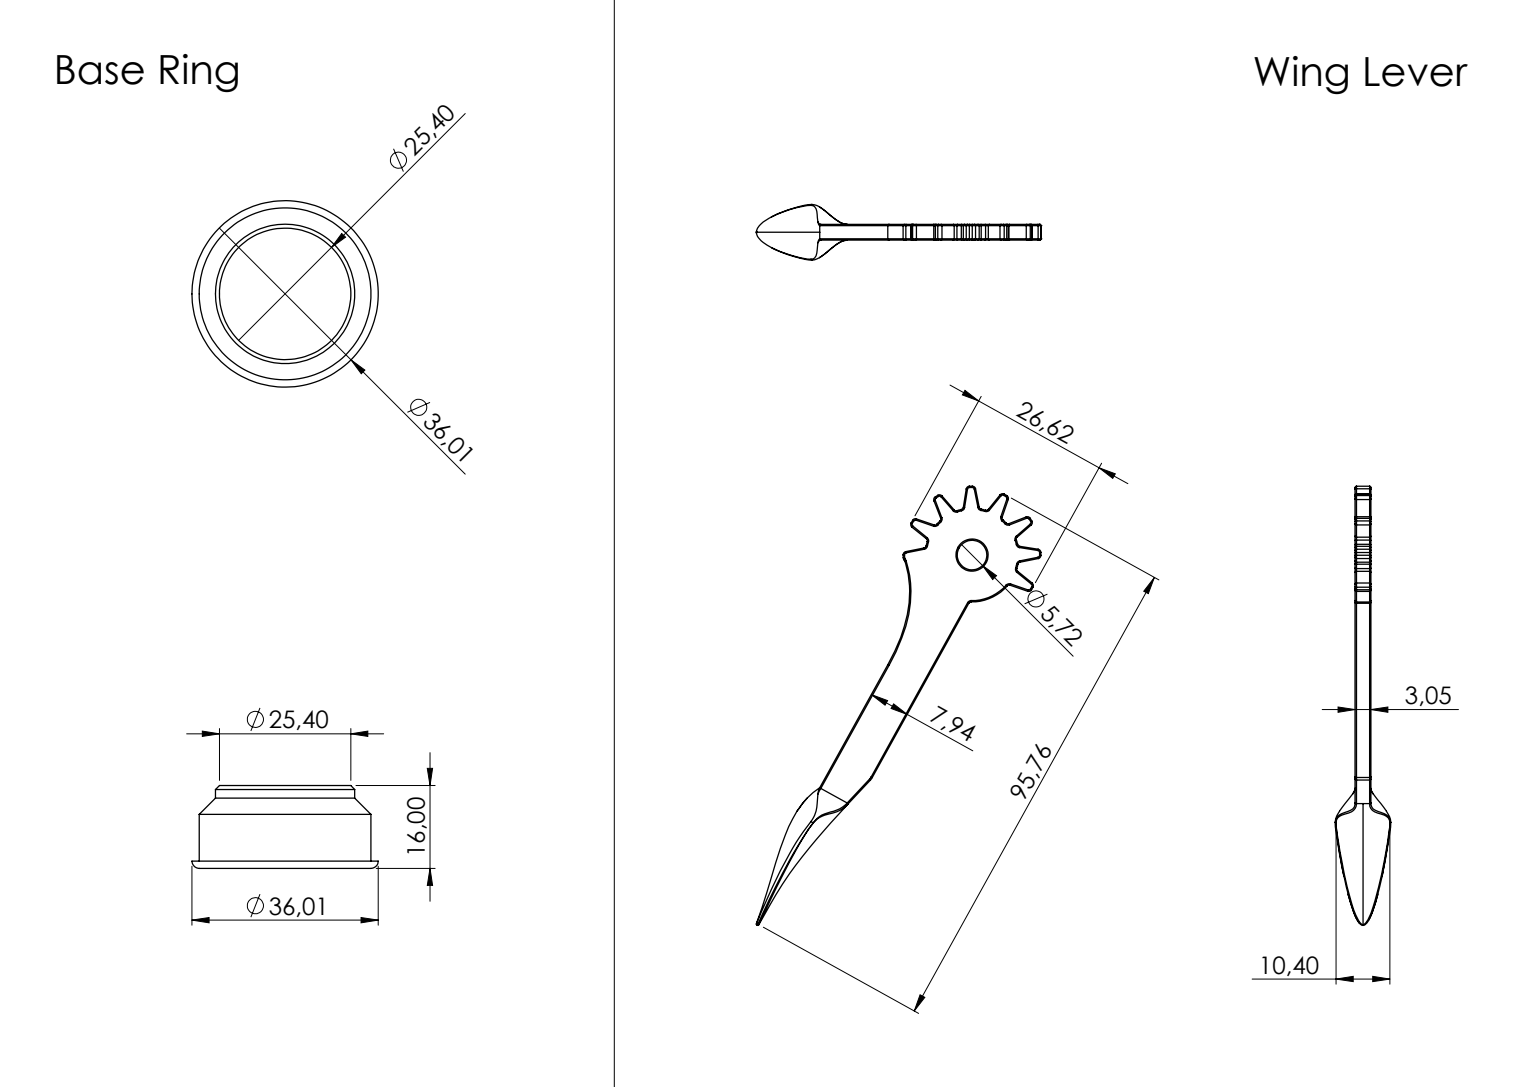
ISO-10303-21;
HEADER;
FILE_DESCRIPTION (('STEP AP214'),
    '1' );
FILE_NAME ('Wing Lever.step',
    '2026-10-06T14:27:08',
    ( '' ),
    ( '' ),
    'SwSTEP 2.0',
    'SolidWorks 2020',
    '' );
FILE_SCHEMA (( 'AUTOMOTIVE_DESIGN' ));
ENDSEC;

DATA;
#7=CARTESIAN_POINT ( 'NONE',  ( -47.84919564605845466, 19.39087073395056393, 5.212699772323899694 ) ) ;
#16=ORIENTED_EDGE ( 'NONE', *, *, #18091, .T. ) ;
#25=VERTEX_POINT ( 'NONE', #23978 ) ;
#26=CARTESIAN_POINT ( 'NONE',  ( -45.52520984822221095, 18.49555408152312452, 0.5880787195337303652 ) ) ;
#39=CARTESIAN_POINT ( 'NONE',  ( -8.428339483816529309, 74.57444062528223583, -1.523999999999996913 ) ) ;
#40=CARTESIAN_POINT ( 'NONE',  ( -58.67410397513675235, -0.3138866149764163449, 0.3147537707000222507 ) ) ;
#41=DIRECTION ( 'NONE',  ( -5.188838149069471174E-16, 1.699382548006136313E-16, 1.000000000000000000 ) ) ;
#44=AXIS2_PLACEMENT_3D ( 'NONE', #23205, #7689, #33679 ) ;
#57=FACE_OUTER_BOUND ( 'NONE', #41013, .T. ) ;
#58=DIRECTION ( 'NONE',  ( 0.6850534820564689875, -0.7284927773988614241, 8.537024980200769556E-16 ) ) ;
#64=( BOUNDED_SURFACE ( )  B_SPLINE_SURFACE ( 3, 2, ( 
 ( #13288, #26273, #2675 ),
 ( #25450, #22223, #6076 ),
 ( #23483, #20083, #948 ),
 ( #10925, #7750, #33106 ),
 ( #39712, #10513, #30310 ),
 ( #17523, #39496, #3725 ),
 ( #3937, #26910, #7329 ),
 ( #23697, #40345, #23915 ),
 ( #16896, #36508, #14119 ),
 ( #36717, #7538, #17320 ),
 ( #27333, #20287, #27119 ),
 ( #20500, #33315, #33527 ),
 ( #4144, #29899, #40134 ),
 ( #37135, #17106, #30523 ),
 ( #16684, #30108, #10716 ),
 ( #4360, #1154, #36307 ) ),
 .UNSPECIFIED., .F., .F., .T. ) 
 B_SPLINE_SURFACE_WITH_KNOTS ( ( 4, 2, 2, 2, 2, 2, 2, 4 ),
 ( 3, 3 ),
 ( -4.336808689942017736E-17, 0.002643305330645566355, 0.003964957995968371000, 0.005286610661291176079, 0.01057322132258239553, 0.01321652665322800395, 0.01585983198387361237, 0.02114644264516483269 ),
 ( 0.000000000000000000, 1.000000000000000000 ),
 .UNSPECIFIED. ) 
 GEOMETRIC_REPRESENTATION_ITEM ( )  RATIONAL_B_SPLINE_SURFACE ( (
 ( 1.000000000000000000, 0.7071067811865429098, 1.000000000000000000),
 ( 1.000000000000000000, 0.7071067811865429098, 1.000000000000000000),
 ( 1.000000000000000000, 0.7071067811865475727, 1.000000000000000000),
 ( 1.000000000000000000, 0.7071067811865475727, 1.000000000000000000),
 ( 1.000000000000000000, 0.7071067811865481278, 1.000000000000000000),
 ( 1.000000000000000000, 0.7071067811865481278, 1.000000000000000000),
 ( 1.000000000000000000, 0.7071067811865477948, 1.000000000000000000),
 ( 1.000000000000000000, 0.7071067811865477948, 1.000000000000000000),
 ( 1.000000000000000000, 0.7071067811865477948, 1.000000000000000000),
 ( 1.000000000000000000, 0.7071067811865477948, 1.000000000000000000),
 ( 1.000000000000000000, 0.7071067811865481278, 1.000000000000000000),
 ( 1.000000000000000000, 0.7071067811865481278, 1.000000000000000000),
 ( 1.000000000000000000, 0.7071067811865477948, 1.000000000000000000),
 ( 1.000000000000000000, 0.7071067811865477948, 1.000000000000000000),
 ( 1.000000000000000000, 0.7071067811865521247, 1.000000000000000000),
 ( 1.000000000000000000, 0.7071067811865521247, 1.000000000000000000) ) ) 
 REPRESENTATION_ITEM ( '' )  SURFACE ( )  );
#65=ORIENTED_EDGE ( 'NONE', *, *, #10499, .F. ) ;
#69=AXIS2_PLACEMENT_3D ( 'NONE', #15499, #34901, #12099 ) ;
#72=EDGE_CURVE ( 'NONE', #18166, #40365, #25788, .T. ) ;
#73=CARTESIAN_POINT ( 'NONE',  ( -58.60980283399052837, -0.2526951616049680216, -0.4333512024961975739 ) ) ;
#75=CARTESIAN_POINT ( 'NONE',  ( -58.36994270878630431, -0.2918297664318836304, -0.01629410684330124051 ) ) ;
#79=DIRECTION ( 'NONE',  ( -0.8745520943968315697, 0.4849315768086414624, -4.878299988686196152E-16 ) ) ;
#84=ORIENTED_EDGE ( 'NONE', *, *, #36137, .T. ) ;
#88=ORIENTED_EDGE ( 'NONE', *, *, #11328, .F. ) ;
#96=CARTESIAN_POINT ( 'NONE',  ( -46.78089565521681692, 25.32111429335293451, 1.738356225806948929 ) ) ;
#100=DIRECTION ( 'NONE',  ( 0.9998501190848640974, 0.01731298258485272981, 8.537024980200786319E-16 ) ) ;
#101=ADVANCED_FACE ( 'NONE', ( #2270 ), #4717, .T. ) ;
#102=EDGE_CURVE ( 'NONE', #36001, #40376, #18003, .T. ) ;
#103=CARTESIAN_POINT ( 'NONE',  ( -49.81365592435692236, 14.60358288955459294, -2.185970286000775253 ) ) ;
#108=FACE_OUTER_BOUND ( 'NONE', #15765, .T. ) ;
#109=CARTESIAN_POINT ( 'NONE',  ( -48.74093372970734350, 18.21380663047653314, 5.157544856658800470 ) ) ;
#111=ADVANCED_FACE ( 'NONE', ( #24605 ), #3343, .T. ) ;
#114=CARTESIAN_POINT ( 'NONE',  ( -53.63638764239521350, 11.23543775674477807, 3.971736527645110648 ) ) ;
#115=CARTESIAN_POINT ( 'NONE',  ( -55.41603145274652320, 6.826612083464994818, 3.210495615568572436 ) ) ;
#118=CARTESIAN_POINT ( 'NONE',  ( -51.90232906080404263, 16.51944673254565643, -2.845700375512763891 ) ) ;
#120=VERTEX_POINT ( 'NONE', #22037 ) ;
#128=CARTESIAN_POINT ( 'NONE',  ( -25.81615557310160369, 74.46796499802707103, -1.270000000000005791 ) ) ;
#135=CARTESIAN_POINT ( 'NONE',  ( -58.30601194912756569, -0.1568608524855368003, -0.3211567528579405972 ) ) ;
#140=AXIS2_PLACEMENT_3D ( 'NONE', #10662, #17050, #30466 ) ;
#147=ORIENTED_EDGE ( 'NONE', *, *, #35169, .T. ) ;
#151=CARTESIAN_POINT ( 'NONE',  ( -47.20791569504334717, 21.28685671521062517, -4.803936552638846891 ) ) ;
#152=ORIENTED_EDGE ( 'NONE', *, *, #37062, .F. ) ;
#155=ADVANCED_FACE ( 'NONE', ( #14807 ), #32569, .T. ) ;
#156=CARTESIAN_POINT ( 'NONE',  ( -9.795036404550216957, 65.29837086945681790, -1.523999999999996025 ) ) ;
#163=AXIS2_PLACEMENT_3D ( 'NONE', #1534, #902, #4938 ) ;
#171=CARTESIAN_POINT ( 'NONE',  ( -31.57591258916109922, 52.94298397416076085, 1.523999999999993582 ) ) ;
#177=DIRECTION ( 'NONE',  ( -0.8745520943968251304, 0.4849315768086532863, -5.424246918827961050E-16 ) ) ;
#187=ORIENTED_EDGE ( 'NONE', *, *, #10423, .F. ) ;
#192=ORIENTED_EDGE ( 'NONE', *, *, #36999, .T. ) ;
#200=CARTESIAN_POINT ( 'NONE',  ( -46.74948388161530488, 25.87427737361800339, 1.400905913749466380 ) ) ;
#201=CARTESIAN_POINT ( 'NONE',  ( -47.14788814370446346, 23.76379789425250166, 2.690610990139707059 ) ) ;
#204=CARTESIAN_POINT ( 'NONE',  ( -53.68435271313694557, 11.12367579685427721, 3.945100831076007619 ) ) ;
#208=ORIENTED_EDGE ( 'NONE', *, *, #17060, .T. ) ;
#214=CARTESIAN_POINT ( 'NONE',  ( -46.68395179480138069, 26.03198510454123848, -1.397000000000007569 ) ) ;
#216=AXIS2_PLACEMENT_3D ( 'NONE', #23878, #24296, #37504 ) ;
#228=ORIENTED_EDGE ( 'NONE', *, *, #36703, .T. ) ;
#229=DIRECTION ( 'NONE',  ( -0.8745520943968235761, 0.4849315768086558398, -5.691349986800547879E-16 ) ) ;
#234=CIRCLE ( 'NONE', #18562, 0.6350000000000036726 ) ;
#237=CARTESIAN_POINT ( 'NONE',  ( -43.02406770836220318, 21.15087974136648086, 0.6363192884523977133 ) ) ;
#250=DIRECTION ( 'NONE',  ( -5.188838149069471174E-16, 1.699382548006136313E-16, 1.000000000000000000 ) ) ;
#252=CARTESIAN_POINT ( 'NONE',  ( -6.135835944515187101, 77.40800365160224317, 1.270000000000003793 ) ) ;
#253=CARTESIAN_POINT ( 'NONE',  ( -58.64207371057519680, -0.3086014758121452539, 0.3447476069572601998 ) ) ;
#257=CIRCLE ( 'NONE', #34949, 0.6350000000000006750 ) ;
#261=EDGE_CURVE ( 'NONE', #2461, #25488, #15017, .T. ) ;
#267=DIRECTION ( 'NONE',  ( -5.188838149069471174E-16, 1.699382548006136313E-16, 1.000000000000000000 ) ) ;
#277=DIRECTION ( 'NONE',  ( 0.8572391118119510045, 0.5149185422762100339, 3.573031421855330583E-16 ) ) ;
#285=CARTESIAN_POINT ( 'NONE',  ( -58.63219855361986532, -0.2943491849813937300, -0.3701125355236437042 ) ) ;
#287=CARTESIAN_POINT ( 'NONE',  ( -17.76856900107737403, 61.81127730225986738, 1.269999999999999352 ) ) ;
#294=CARTESIAN_POINT ( 'NONE',  ( -57.83637253161431602, 2.237724655402451024, -1.757929103219309397 ) ) ;
#295=CIRCLE ( 'NONE', #24741, 0.7620000000000015650 ) ;
#302=EDGE_CURVE ( 'NONE', #37691, #28646, #26431, .T. ) ;
#310=AXIS2_PLACEMENT_3D ( 'NONE', #29921, #20311, #10947 ) ;
#311=EDGE_CURVE ( 'NONE', #34241, #32706, #19639, .T. ) ;
#314=DIRECTION ( 'NONE',  ( -0.8745520943968235761, 0.4849315768086558398, -5.691349986800547879E-16 ) ) ;
#316=CARTESIAN_POINT ( 'NONE',  ( -46.49274047292066570, 18.53875678104565594, -2.063467562158697088 ) ) ;
#318=DIRECTION ( 'NONE',  ( -0.8572391118119438991, -0.5149185422762221354, -3.573031421855274870E-16 ) ) ;
#319=CARTESIAN_POINT ( 'NONE',  ( -46.79329363240532302, 25.76054971305726937, -1.464668473915645253 ) ) ;
#324=CARTESIAN_POINT ( 'NONE',  ( -25.56614996202194590, 73.65611136973726047, -1.524000000000005572 ) ) ;
#325=CARTESIAN_POINT ( 'NONE',  ( -57.34105142390577470, 4.241571993195747403, 0.1395372036359874557 ) ) ;
#326=CARTESIAN_POINT ( 'NONE',  ( -57.57967628038989005, 1.451576601202181349, 1.494865757154131725 ) ) ;
#330=CARTESIAN_POINT ( 'NONE',  ( -50.78366386294959511, 19.84645248585079003, -1.614153572948420212 ) ) ;
#332=VERTEX_POINT ( 'NONE', #9690 ) ;
#347=ORIENTED_EDGE ( 'NONE', *, *, #18115, .F. ) ;
#349=FACE_OUTER_BOUND ( 'NONE', #29106, .T. ) ;
#355=DIRECTION ( 'NONE',  ( -0.8745520943968243532, 0.4849315768086547296, -6.829619984160642269E-16 ) ) ;
#356=EDGE_CURVE ( 'NONE', #12580, #5531, #25752, .T. ) ;
#364=CARTESIAN_POINT ( 'NONE',  ( -47.07934102874902749, 22.98505637820369429, -3.579966862081945145 ) ) ;
#365=ORIENTED_EDGE ( 'NONE', *, *, #1402, .T. ) ;
#367=CYLINDRICAL_SURFACE ( 'NONE', #41319, 0.2540000000000012248 ) ;
#374=CARTESIAN_POINT ( 'NONE',  ( -58.36930655268525214, -0.2905277127126757453, 0.02713858147964411452 ) ) ;
#378=ORIENTED_EDGE ( 'NONE', *, *, #26047, .T. ) ;
#386=ORIENTED_EDGE ( 'NONE', *, *, #4860, .T. ) ;
#390=DIRECTION ( 'NONE',  ( -0.8745520943968240202, 0.4849315768086553402, -6.829619984160650158E-16 ) ) ;
#396=CARTESIAN_POINT ( 'NONE',  ( -14.38915334913366806, 80.27078028363496287, -1.270000000000000906 ) ) ;
#400=ORIENTED_EDGE ( 'NONE', *, *, #39413, .T. ) ;
#405=CARTESIAN_POINT ( 'NONE',  ( -46.47694366848595848, 20.52739116796146135, 4.723822614977957635 ) ) ;
#408=ORIENTED_EDGE ( 'NONE', *, *, #24603, .T. ) ;
#416=CARTESIAN_POINT ( 'NONE',  ( -48.72131418994864305, 18.20897304993750865, 5.123370244626707759 ) ) ;
#417=CARTESIAN_POINT ( 'NONE',  ( -49.93085365557847410, 21.08514737284949803, 1.613137678015111209 ) ) ;
#419=CARTESIAN_POINT ( 'NONE',  ( -53.17586183559576085, 10.67386474145934372, 4.017225210190868978 ) ) ;
#420=CARTESIAN_POINT ( 'NONE',  ( -58.76893202732499333, -0.3048440090616499898, 0.2012342470266328676 ) ) ;
#422=CARTESIAN_POINT ( 'NONE',  ( -58.11144429832075531, 0.1746852717545294142, -1.017628075538466478E-14 ) ) ;
#424=ORIENTED_EDGE ( 'NONE', *, *, #18869, .T. ) ;
#425=CARTESIAN_POINT ( 'NONE',  ( -47.11704014324646295, 20.18577099567727373, 5.127035723291425207 ) ) ;
#437=AXIS2_PLACEMENT_3D ( 'NONE', #20686, #27092, #27925 ) ;
#442=DIRECTION ( 'NONE',  ( -5.188838149069472160E-16, 1.699382548006136559E-16, 1.000000000000000000 ) ) ;
#451=CARTESIAN_POINT ( 'NONE',  ( -46.43071087740785430, 19.11736041196146374, 2.831212230509037031 ) ) ;
#457=DIRECTION ( 'NONE',  ( 5.188838149069472160E-16, -1.699382548006136559E-16, -1.000000000000000000 ) ) ;
#458=EDGE_CURVE ( 'NONE', #25310, #10068, #9439, .T. ) ;
#467=FACE_OUTER_BOUND ( 'NONE', #8526, .T. ) ;
#468=TOROIDAL_SURFACE ( 'NONE', #24241, 0.7620000000000000107, 0.2540000000000000036 ) ;
#472=FACE_OUTER_BOUND ( 'NONE', #6866, .T. ) ;
#480=CARTESIAN_POINT ( 'NONE',  ( -7.921807157844599878, 72.80702234259206307, 1.524000000000002242 ) ) ;
#484=DIRECTION ( 'NONE',  ( 5.188838149069472160E-16, -1.699382548006136559E-16, -1.000000000000000000 ) ) ;
#485=CARTESIAN_POINT ( 'NONE',  ( -19.21741104974024594, 79.92823415920659613, -1.270000000000003348 ) ) ;
#499=CARTESIAN_POINT ( 'NONE',  ( -58.67914983968596232, -0.3139907887120958474, -0.3103399889725807492 ) ) ;
#500=VERTEX_POINT ( 'NONE', #19477 ) ;
#502=AXIS2_PLACEMENT_3D ( 'NONE', #34156, #17941, #1783 ) ;
#509=CARTESIAN_POINT ( 'NONE',  ( -57.69570286664291103, 2.558035660193719529, -1.875687456014384802 ) ) ;
#510=ORIENTED_EDGE ( 'NONE', *, *, #6687, .F. ) ;
#514=VERTEX_POINT ( 'NONE', #32485 ) ;
#518=VECTOR ( 'NONE', #3109, 1000.000000000000114 ) ;
#519=CARTESIAN_POINT ( 'NONE',  ( -58.36994270878681590, -0.2918297664328134422, 0.01629410684326380171 ) ) ;
#525=DIRECTION ( 'NONE',  ( -5.188838149069471174E-16, 1.699382548006136313E-16, 1.000000000000000000 ) ) ;
#526=VECTOR ( 'NONE', #36681, 1000.000000000000000 ) ;
#527=CARTESIAN_POINT ( 'NONE',  ( -55.83515739322318439, 4.224161455597882586, -1.000857388952954637E-14 ) ) ;
#531=CARTESIAN_POINT ( 'NONE',  ( -7.842268484490568348, 73.30875693322846587, -1.269999999999996243 ) ) ;
#534=CARTESIAN_POINT ( 'NONE',  ( -57.40598286442868670, 3.481741809872221260, 1.566274799519910887 ) ) ;
#535=CARTESIAN_POINT ( 'NONE',  ( -58.24002838079472610, 0.001074765447070524793, 0.6562585879479657658 ) ) ;
#537=VERTEX_POINT ( 'NONE', #16279 ) ;
#538=CARTESIAN_POINT ( 'NONE',  ( -51.27035844764527184, 15.91047978596967560, -4.316378984520668816 ) ) ;
#547=CIRCLE ( 'NONE', #3954, 0.3810000000000032250 ) ;
#553=DIRECTION ( 'NONE',  ( 0.9876665170007974393, -0.1565721916417901483, 8.537024980200831679E-16 ) ) ;
#555=ORIENTED_EDGE ( 'NONE', *, *, #38050, .F. ) ;
#557=CARTESIAN_POINT ( 'NONE',  ( -58.01365450750562047, 0.4748094611197187787, -0.8404086423206994505 ) ) ;
#564=EDGE_CURVE ( 'NONE', #9964, #36869, #25095, .T. ) ;
#567=ORIENTED_EDGE ( 'NONE', *, *, #41507, .F. ) ;
#572=CARTESIAN_POINT ( 'NONE',  ( -47.16890147375937659, 22.20336809214646578, -4.187060126831891438 ) ) ;
#573=LINE ( 'NONE', #23318, #10916 ) ;
#575=CARTESIAN_POINT ( 'NONE',  ( -27.88833342972739615, 78.11058938209563962, -1.270000000000007345 ) ) ;
#604=CARTESIAN_POINT ( 'NONE',  ( -47.85244527695891037, 19.39403540832955386, -5.219971639306618449 ) ) ;
#610=EDGE_CURVE ( 'NONE', #41136, #7000, #5386, .T. ) ;
#616=DIRECTION ( 'NONE',  ( -0.4849315768086427392, -0.8745520943968311256, -4.371515779989697137E-15 ) ) ;
#618=ADVANCED_FACE ( 'NONE', ( #13731 ), #41434, .T. ) ;
#629=CARTESIAN_POINT ( 'NONE',  ( -47.23483502501005660, 23.02499599010462816, 3.263444997004413484 ) ) ;
#631=CARTESIAN_POINT ( 'NONE',  ( -55.03109054507046238, 6.816801101491506643, 3.135084751894912980 ) ) ;
#632=CARTESIAN_POINT ( 'NONE',  ( -58.18166364753805908, 0.6689161199004037828, 1.158115574925229874 ) ) ;
#633=EDGE_CURVE ( 'NONE', #4427, #35981, #26379, .T. ) ;
#636=EDGE_LOOP ( 'NONE', ( #9709, #30418, #35800, #17027 ) ) ;
#637=CARTESIAN_POINT ( 'NONE',  ( -43.24646561529713296, 21.63922848039483071, 2.381786957946262273 ) ) ;
#661=CARTESIAN_POINT ( 'NONE',  ( -45.37978287637889707, 19.43610829578849675, 1.699483007375117261 ) ) ;
#674=DIRECTION ( 'NONE',  ( -5.188838149069472160E-16, 1.699382548006136559E-16, 1.000000000000000000 ) ) ;
#675=AXIS2_PLACEMENT_3D ( 'NONE', #9781, #12563, #22749 ) ;
#691=EDGE_CURVE ( 'NONE', #32986, #18705, #32617, .T. ) ;
#692=DIRECTION ( 'NONE',  ( 0.1565721916417901483, 0.9876665170007974393, 0.000000000000000000 ) ) ;
#697=AXIS2_PLACEMENT_3D ( 'NONE', #7791, #34985, #20752 ) ;
#698=ADVANCED_FACE ( 'NONE', ( #22165 ), #38397, .F. ) ;
#699=CARTESIAN_POINT ( 'NONE',  ( -4.095482865093057256, 71.62450171983788039, -1.523999999999994026 ) ) ;
#701=CARTESIAN_POINT ( 'NONE',  ( -8.539387426415398608, 74.43734692935288422, 1.270000000000002460 ) ) ;
#702=VERTEX_POINT ( 'NONE', #31989 ) ;
#708=CARTESIAN_POINT ( 'NONE',  ( -58.61966295912883140, -0.2719594648587958519, -0.4054877843427013850 ) ) ;
#713=DIRECTION ( 'NONE',  ( 0.4849315768086534528, 0.8745520943968250194, 1.030032898892974942E-16 ) ) ;
#717=ORIENTED_EDGE ( 'NONE', *, *, #6839, .T. ) ;
#720=EDGE_LOOP ( 'NONE', ( #24810, #4180, #22560, #38384 ) ) ;
#723=FACE_OUTER_BOUND ( 'NONE', #37524, .T. ) ;
#731=CARTESIAN_POINT ( 'NONE',  ( -55.75614604655159923, 4.795084387130554404, -1.238208353029769393 ) ) ;
#733=DIRECTION ( 'NONE',  ( -0.8745520943968235761, 0.4849315768086558398, -4.268512490100410909E-16 ) ) ;
#734=DIRECTION ( 'NONE',  ( 5.188838149069472160E-16, -1.699382548006136559E-16, -1.000000000000000000 ) ) ;
#735=CARTESIAN_POINT ( 'NONE',  ( -5.719305292821792008, 76.92870498041706639, -1.523999999999995802 ) ) ;
#736=CARTESIAN_POINT ( 'NONE',  ( -26.07955644221209113, 72.55303096390359485, -1.524000000000005794 ) ) ;
#741=CARTESIAN_POINT ( 'NONE',  ( -58.07447437077728125, 1.735896131820596766, 1.499107834811089557 ) ) ;
#742=CARTESIAN_POINT ( 'NONE',  ( -58.40597088826705630, 0.2738206778524349128, 0.9753506901443759203 ) ) ;
#745=CARTESIAN_POINT ( 'NONE',  ( -57.87117896969294861, 2.397448601660856493, -0.9757051360025802422 ) ) ;
#749=VECTOR ( 'NONE', #9550, 1000.000000000000114 ) ;
#759=CARTESIAN_POINT ( 'NONE',  ( -30.44847906516384128, 70.61110078258337808, -1.270000000000007345 ) ) ;
#763=CARTESIAN_POINT ( 'NONE',  ( -57.81393215990352275, 0.9072688167287735750, -1.084054936344124753 ) ) ;
#769=DIRECTION ( 'NONE',  ( 0.9734199927291280474, 0.2290273297124694185, 8.537024980200812943E-16 ) ) ;
#775=CARTESIAN_POINT ( 'NONE',  ( -10.39456080247343905, 81.94606122948148652, -1.523999999999999133 ) ) ;
#778=CARTESIAN_POINT ( 'NONE',  ( -49.66210360255988832, 16.76989353321783227, -4.946330335750499962 ) ) ;
#781=CARTESIAN_POINT ( 'NONE',  ( -5.878298779570172883, 78.21245918282636467, -1.269999999999996243 ) ) ;
#782=VECTOR ( 'NONE', #16189, 1000.000000000000227 ) ;
#787=CARTESIAN_POINT ( 'NONE',  ( -44.21430376968341847, 21.24218795319825404, -2.931160726117711945 ) ) ;
#789=DIRECTION ( 'NONE',  ( 0.5149185422762221354, -0.8572391118119438991, 4.128606161907600514E-16 ) ) ;
#792=EDGE_LOOP ( 'NONE', ( #21978, #15513, #15968, #18508 ) ) ;
#794=DIRECTION ( 'NONE',  ( 0.8745520943968249084, -0.4849315768086533418, 5.311926654347176508E-16 ) ) ;
#799=AXIS2_PLACEMENT_3D ( 'NONE', #34127, #41784, #3016 ) ;
#801=ORIENTED_EDGE ( 'NONE', *, *, #5335, .F. ) ;
#809=CARTESIAN_POINT ( 'NONE',  ( -57.60629982073510291, 1.412843483090786334, -1.546595473639808871 ) ) ;
#810=DIRECTION ( 'NONE',  ( -0.8745520943968243532, 0.4849315768086547296, -6.829619984160642269E-16 ) ) ;
#812=AXIS2_PLACEMENT_3D ( 'NONE', #2923, #3130, #15676 ) ;
#820=ORIENTED_EDGE ( 'NONE', *, *, #9466, .T. ) ;
#823=CARTESIAN_POINT ( 'NONE',  ( -46.59331663807144253, 25.66825226916589031, -1.575831774160291188 ) ) ;
#824=VECTOR ( 'NONE', #37244, 1000.000000000000000 ) ;
#833=CARTESIAN_POINT ( 'NONE',  ( -55.83462464969977646, 5.104280077925408499, 2.555929569707788396 ) ) ;
#834=CARTESIAN_POINT ( 'NONE',  ( -49.70354115100154502, 23.42381831551578486, 0.3024929150989305038 ) ) ;
#836=CARTESIAN_POINT ( 'NONE',  ( -56.80697847991661575, 4.636179106009441497, 2.484889565616565488 ) ) ;
#837=CARTESIAN_POINT ( 'NONE',  ( -58.62921133459555989, -0.2893463222253165879, 0.3783962402783414003 ) ) ;
#842=CARTESIAN_POINT ( 'NONE',  ( -45.39816439898302036, 21.06106408185672763, 4.080402960186377825 ) ) ;
#843=AXIS2_PLACEMENT_3D ( 'NONE', #9004, #2627, #21753 ) ;
#852=EDGE_CURVE ( 'NONE', #35513, #25, #28474, .T. ) ;
#853=LINE ( 'NONE', #4473, #7845 ) ;
#854=CARTESIAN_POINT ( 'NONE',  ( -46.50210365330781315, 20.51386735866382693, 4.739171082384512346 ) ) ;
#864=TOROIDAL_SURFACE ( 'NONE', #11023, 0.3810000000000005604, 0.2540000000000000036 ) ;
#866=ORIENTED_EDGE ( 'NONE', *, *, #18744, .T. ) ;
#867=CARTESIAN_POINT ( 'NONE',  ( -44.09535491252989203, 20.89266065238331294, 2.220044762595780874 ) ) ;
#874=CARTESIAN_POINT ( 'NONE',  ( -3.831877602099685198, 71.07198261757335445, 1.270000000000004459 ) ) ;
#881=CYLINDRICAL_SURFACE ( 'NONE', #38363, 0.6349999999999998979 ) ;
#885=DIRECTION ( 'NONE',  ( -0.8745520943968241312, 0.4849315768086548406, -5.691349986800536046E-16 ) ) ;
#887=VECTOR ( 'NONE', #18519, 1000.000000000000000 ) ;
#889=DIRECTION ( 'NONE',  ( -0.8745520943968240202, 0.4849315768086551737, -5.361993529360572958E-16 ) ) ;
#892=ORIENTED_EDGE ( 'NONE', *, *, #14638, .F. ) ;
#901=DIRECTION ( 'NONE',  ( 0.4849315768086556733, 0.8745520943968236871, -8.647447314816538780E-15 ) ) ;
#902=DIRECTION ( 'NONE',  ( 5.188838149069472160E-16, -1.699382548006136559E-16, -1.000000000000000000 ) ) ;
#908=LINE ( 'NONE', #14083, #2563 ) ;
#915=VERTEX_POINT ( 'NONE', #7696 ) ;
#916=CARTESIAN_POINT ( 'NONE',  ( -41.23752580366542020, 23.26788267949596190, 1.269999999999994245 ) ) ;
#919=CARTESIAN_POINT ( 'NONE',  ( -47.73411474416273137, 19.53609852428665050, 5.217284324673509666 ) ) ;
#925=CIRCLE ( 'NONE', #13125, 0.2540000000000011693 ) ;
#935=CARTESIAN_POINT ( 'NONE',  ( -49.23283723365464937, 17.42967204962415195, 5.014312523175059155 ) ) ;
#942=CARTESIAN_POINT ( 'NONE',  ( -56.37071950982826252, 3.976973756211601874, -2.203872415222129177 ) ) ;
#946=DIRECTION ( 'NONE',  ( -0.8745520943968240202, 0.4849315768086553402, -5.361993529360572958E-16 ) ) ;
#947=CARTESIAN_POINT ( 'NONE',  ( -25.81615557310160014, 74.46796499802707103, -1.524000000000005794 ) ) ;
#948=CARTESIAN_POINT ( 'NONE',  ( -29.67105550542181547, 68.29201113455899019, -1.270000000000484519 ) ) ;
#951=FACE_OUTER_BOUND ( 'NONE', #38983, .T. ) ;
#952=CARTESIAN_POINT ( 'NONE',  ( -58.33777482027512207, 1.113448835244237767, 1.208045587469420701 ) ) ;
#955=ORIENTED_EDGE ( 'NONE', *, *, #9252, .T. ) ;
#956=CARTESIAN_POINT ( 'NONE',  ( -57.93941708942283952, 2.052042089854988483, -1.628789306319528896 ) ) ;
#959=CARTESIAN_POINT ( 'NONE',  ( -17.14500000000466784, 71.11999999999886768, -1.524000000000000909 ) ) ;
#971=ORIENTED_EDGE ( 'NONE', *, *, #2183, .F. ) ;
#974=CARTESIAN_POINT ( 'NONE',  ( -57.67508898341257151, 1.207211884619313835, -1.229746519219142353 ) ) ;
#977=VECTOR ( 'NONE', #10715, 1000.000000000000114 ) ;
#978=CIRCLE ( 'NONE', #24748, 0.7620000000000000107 ) ;
#981=CARTESIAN_POINT ( 'NONE',  ( -44.36446822842629700, 21.81554158013422651, -2.896954608336749892 ) ) ;
#988=CIRCLE ( 'NONE', #32252, 0.5080000000000000071 ) ;
#989=CARTESIAN_POINT ( 'NONE',  ( -58.82991074935231524, -0.2577531494038359794, -1.058401375502683064E-14 ) ) ;
#991=EDGE_CURVE ( 'NONE', #15388, #35792, #6846, .T. ) ;
#992=CARTESIAN_POINT ( 'NONE',  ( -53.75224695799815322, 9.373383622779334345, -3.688627211158436392 ) ) ;
#993=DIRECTION ( 'NONE',  ( -0.8745520943968245753, 0.4849315768086539524, -5.691349986800526185E-16 ) ) ;
#995=CARTESIAN_POINT ( 'NONE',  ( -14.42383115828894624, 69.61113539875873357, 1.270000000000000018 ) ) ;
#1000=CARTESIAN_POINT ( 'NONE',  ( -9.712308604790299782, 65.53852105402241079, -1.523999999999996025 ) ) ;
#1003=VERTEX_POINT ( 'NONE', #3662 ) ;
#1004=CARTESIAN_POINT ( 'NONE',  ( -47.04217617083259029, 23.73857702128102076, -2.948847133965297740 ) ) ;
#1006=FACE_OUTER_BOUND ( 'NONE', #25111, .T. ) ;
#1008=CYLINDRICAL_SURFACE ( 'NONE', #1562, 0.2539999999999931202 ) ;
#1023=CARTESIAN_POINT ( 'NONE',  ( -57.89036626108683237, 0.7933261799619758525, -1.256022413937835092 ) ) ;
#1034=ORIENTED_EDGE ( 'NONE', *, *, #302, .F. ) ;
#1037=CARTESIAN_POINT ( 'NONE',  ( -18.58115504727956591, 80.30342350548193053, -1.524000000000003130 ) ) ;
#1041=CARTESIAN_POINT ( 'NONE',  ( -23.21760062652228385, 78.26400813401573942, -1.270000000000005125 ) ) ;
#1045=CARTESIAN_POINT ( 'NONE',  ( -57.39381155807401313, 1.812545739600947892, 1.491594637569517712 ) ) ;
#1046=CARTESIAN_POINT ( 'NONE',  ( -50.64083584635693569, 22.17031203569813513, -9.591688330814065574E-15 ) ) ;
#1048=CARTESIAN_POINT ( 'NONE',  ( -49.01671973967521012, 18.67808020721676954, 5.174630477995038724 ) ) ;
#1049=CARTESIAN_POINT ( 'NONE',  ( -58.60011173050265398, -0.2330837761818443932, 0.4599256431870107908 ) ) ;
#1053=CARTESIAN_POINT ( 'NONE',  ( -44.90991502375803890, 23.16658271142636139, 2.247441098035892981 ) ) ;
#1062=DIRECTION ( 'NONE',  ( -0.8745520943968367877, 0.4849315768086320255, -4.268512490100441970E-16 ) ) ;
#1065=DIRECTION ( 'NONE',  ( 0.8745520943968253524, -0.4849315768086530087, 8.537024980200771528E-16 ) ) ;
#1074=CARTESIAN_POINT ( 'NONE',  ( -49.14072577824710208, 13.89916973120787524, 0.4067138869237276744 ) ) ;
#1076=AXIS2_PLACEMENT_3D ( 'NONE', #34899, #5731, #18684 ) ;
#1085=CARTESIAN_POINT ( 'NONE',  ( -29.82321757229076908, 71.17901112636586447, -1.524000000000007349 ) ) ;
#1088=VERTEX_POINT ( 'NONE', #7273 ) ;
#1092=CARTESIAN_POINT ( 'NONE',  ( -8.761523658392189162, 74.56051954986229191, 1.270000000000002016 ) ) ;
#1099=VECTOR ( 'NONE', #37403, 1000.000000000000000 ) ;
#1105=CARTESIAN_POINT ( 'NONE',  ( -29.81357423954495189, 70.62209452652477637, 1.269999999999992690 ) ) ;
#1108=DIRECTION ( 'NONE',  ( -0.9876665170007972172, 0.1565721916417913695, -1.707025578116413603E-15 ) ) ;
#1111=ADVANCED_FACE ( 'NONE', ( #472 ), #30359, .T. ) ;
#1115=PLANE ( 'NONE',  #36582 ) ;
#1116=VERTEX_POINT ( 'NONE', #13445 ) ;
#1130=FACE_OUTER_BOUND ( 'NONE', #36755, .T. ) ;
#1135=VECTOR ( 'NONE', #1960, 1000.000000000000114 ) ;
#1136=ORIENTED_EDGE ( 'NONE', *, *, #610, .T. ) ;
#1139=CARTESIAN_POINT ( 'NONE',  ( -49.99157512321825436, 16.20856241626540850, 4.827055480670583876 ) ) ;
#1140=EDGE_CURVE ( 'NONE', #26949, #14480, #27277, .T. ) ;
#1146=CARTESIAN_POINT ( 'NONE',  ( -23.69188486464780752, 78.08202335040543574, 1.523999999999994026 ) ) ;
#1147=EDGE_CURVE ( 'NONE', #25488, #14172, #10631, .T. ) ;
#1148=CARTESIAN_POINT ( 'NONE',  ( -56.40799993875704388, 3.472264316502340797, -0.7602746155037358733 ) ) ;
#1150=AXIS2_PLACEMENT_3D ( 'NONE', #33200, #33825, #37022 ) ;
#1154=CARTESIAN_POINT ( 'NONE',  ( -33.42971872652992005, 49.93539301574497102, -1.524000000000002020 ) ) ;
#1158=CARTESIAN_POINT ( 'NONE',  ( -58.83227707057483968, -0.08366279997992775996, 0.2458995907044888019 ) ) ;
#1162=EDGE_LOOP ( 'NONE', ( #510, #2964, #28536, #33915 ) ) ;
#1163=CARTESIAN_POINT ( 'NONE',  ( -56.90265763162630464, 5.074588416753345044, -1.064700026618667916 ) ) ;
#1164=CARTESIAN_POINT ( 'NONE',  ( -17.14500000000466784, 71.11999999999886768, 1.269999999999998241 ) ) ;
#1178=ORIENTED_EDGE ( 'NONE', *, *, #30777, .T. ) ;
#1181=CARTESIAN_POINT ( 'NONE',  ( -57.38104596627693610, 1.839918025084400055, -1.502438007877956672 ) ) ;
#1186=CARTESIAN_POINT ( 'NONE',  ( -46.40591231939538375, 23.70796668624020853, -2.618124260499401945 ) ) ;
#1187=TOROIDAL_SURFACE ( 'NONE', #27700, 3.111499999999999488, 0.2540000000000000036 ) ;
#1190=EDGE_CURVE ( 'NONE', #24894, #28559, #8603, .T. ) ;
#1192=VERTEX_POINT ( 'NONE', #8730 ) ;
#1195=DIRECTION ( 'NONE',  ( -0.4849315768086535083, -0.8745520943968250194, -1.030032898892974695E-16 ) ) ;
#1197=CARTESIAN_POINT ( 'NONE',  ( -53.68435271313694557, 11.12367579685427721, -3.945100831076026715 ) ) ;
#1198=AXIS2_PLACEMENT_3D ( 'NONE', #531, #13504, #10303 ) ;
#1206=EDGE_CURVE ( 'NONE', #18870, #14176, #19467, .T. ) ;
#1208=CARTESIAN_POINT ( 'NONE',  ( -8.584304875092012566, 68.18838345945393087, 1.270000000000003348 ) ) ;
#1210=CIRCLE ( 'NONE', #37919, 0.3809999999999984510 ) ;
#1211=CARTESIAN_POINT ( 'NONE',  ( -57.76865908382304582, 0.8624112519253351872, 0.3783812474402863946 ) ) ;
#1214=CARTESIAN_POINT ( 'NONE',  ( -46.93283292234357162, 25.30718002661817323, -1.635697237164840834 ) ) ;
#1216=CARTESIAN_POINT ( 'NONE',  ( -47.19079517381227618, 25.11791606914807318, -2.000773461933185615 ) ) ;
#1222=CYLINDRICAL_SURFACE ( 'NONE', #17916, 0.2539999999999997260 ) ;
#1228=CARTESIAN_POINT ( 'NONE',  ( -30.19451713491628198, 70.61549828015994024, -1.270000000000007345 ) ) ;
#1229=CYLINDRICAL_SURFACE ( 'NONE', #37378, 0.5080000000000000071 ) ;
#1236=CARTESIAN_POINT ( 'NONE',  ( -56.60409974985478243, 4.028981045513427617, -2.444348447022182125 ) ) ;
#1241=ORIENTED_EDGE ( 'NONE', *, *, #20043, .F. ) ;
#1245=CARTESIAN_POINT ( 'NONE',  ( -47.32981077577479567, 19.92739019301375336, 5.119713631626648720 ) ) ;
#1256=DIRECTION ( 'NONE',  ( -0.6294287539883864913, -0.7770581983690970640, 0.000000000000000000 ) ) ;
#1258=DIRECTION ( 'NONE',  ( 5.188838149069472160E-16, -1.699382548006136559E-16, -1.000000000000000000 ) ) ;
#1259=CARTESIAN_POINT ( 'NONE',  ( -55.96400101662930382, 4.835333878257412010, 2.481606003085900625 ) ) ;
#1261=CARTESIAN_POINT ( 'NONE',  ( -57.53497731650991653, 2.247686704661286505, 1.882970859819747433 ) ) ;
#1262=CARTESIAN_POINT ( 'NONE',  ( -57.61145207080065234, 1.897832464664358509, 1.722955516460566772 ) ) ;
#1265=VERTEX_POINT ( 'NONE', #17883 ) ;
#1266=CARTESIAN_POINT ( 'NONE',  ( -43.49527490626578441, 22.26612824116996237, 2.150709692269567874 ) ) ;
#1276=CARTESIAN_POINT ( 'NONE',  ( -30.20416046766209917, 71.17241488000101413, 1.269999999999991580 ) ) ;
#1287=ORIENTED_EDGE ( 'NONE', *, *, #17004, .T. ) ;
#1288=CARTESIAN_POINT ( 'NONE',  ( -50.77948459960266092, 12.22376025917672138, 0.7375277020707294851 ) ) ;
#1294=EDGE_LOOP ( 'NONE', ( #9321, #12008, #12666, #41017 ) ) ;
#1295=CIRCLE ( 'NONE', #30513, 0.2540000000000000036 ) ;
#1304=DIRECTION ( 'NONE',  ( 5.188838149069472160E-16, -1.699382548006136559E-16, -1.000000000000000000 ) ) ;
#1306=CIRCLE ( 'NONE', #32565, 0.5080000000000000071 ) ;
#1319=FACE_OUTER_BOUND ( 'NONE', #3397, .T. ) ;
#1321=CARTESIAN_POINT ( 'NONE',  ( -7.842268484490568348, 73.30875693322846587, -1.523999999999996247 ) ) ;
#1326=DIRECTION ( 'NONE',  ( -0.6594218222380416883, -0.7517731442105793915, 0.000000000000000000 ) ) ;
#1332=ORIENTED_EDGE ( 'NONE', *, *, #22941, .T. ) ;
#1333=EDGE_LOOP ( 'NONE', ( #21722, #36591, #25860, #38452 ) ) ;
#1337=CARTESIAN_POINT ( 'NONE',  ( -44.94860120752490218, 21.36157935410335895, 3.600951685817770365 ) ) ;
#1338=CIRCLE ( 'NONE', #14928, 2.857500000000000817 ) ;
#1342=FACE_OUTER_BOUND ( 'NONE', #40799, .T. ) ;
#1345=ORIENTED_EDGE ( 'NONE', *, *, #4341, .F. ) ;
#1347=DIRECTION ( 'NONE',  ( -0.6294287539883844929, -0.7770581983690987293, 0.000000000000000000 ) ) ;
#1348=CARTESIAN_POINT ( 'NONE',  ( -57.55255837555638010, 1.471581310123065700, 1.351947345340770656 ) ) ;
#1355=CARTESIAN_POINT ( 'NONE',  ( -46.79259615289808494, 25.76143605979575923, 1.464524644194001635 ) ) ;
#1356=AXIS2_PLACEMENT_3D ( 'NONE', #28783, #38173, #12177 ) ;
#1358=CARTESIAN_POINT ( 'NONE',  ( -53.01551111795198068, 8.729259440421092364, -0.3204493394367286530 ) ) ;
#1361=CARTESIAN_POINT ( 'NONE',  ( -30.75918919842648336, 69.77432548395512413, 1.269999999999991358 ) ) ;
#1365=DIRECTION ( 'NONE',  ( -0.8745520943968250194, 0.4849315768086532863, -5.361993529360574930E-16 ) ) ;
#1367=CARTESIAN_POINT ( 'NONE',  ( -58.16317756775203662, 1.603007233358586081, 1.028822313162477631 ) ) ;
#1368=EDGE_CURVE ( 'NONE', #6241, #29982, #30885, .T. ) ;
#1372=CARTESIAN_POINT ( 'NONE',  ( -57.96050266256141725, 2.261623006455215634, -0.4698253072426236132 ) ) ;
#1375=DIRECTION ( 'NONE',  ( -0.9998501190848629872, -0.01731298258490746381, -8.537024980200835623E-16 ) ) ;
#1381=CARTESIAN_POINT ( 'NONE',  ( -29.22193451008083542, 63.05474646772795921, 1.269999999999993578 ) ) ;
#1383=CARTESIAN_POINT ( 'NONE',  ( -50.24489010722032845, 15.90173676724104723, -4.871286304140493684 ) ) ;
#1384=ADVANCED_FACE ( 'NONE', ( #1725 ), #14619, .F. ) ;
#1389=CARTESIAN_POINT ( 'NONE',  ( -57.94428360355602337, 0.6253113912629046922, -0.9307620923768729071 ) ) ;
#1393=CARTESIAN_POINT ( 'NONE',  ( -46.91604881613255174, 25.30076613767161220, -1.786867259277528985 ) ) ;
#1400=DIRECTION ( 'NONE',  ( -0.4849315768086535083, -0.8745520943968250194, -1.030032898892974695E-16 ) ) ;
#1402=EDGE_CURVE ( 'NONE', #5536, #5052, #39044, .T. ) ;
#1403=CARTESIAN_POINT ( 'NONE',  ( -51.73272837791831336, 13.19950324185369794, -4.393710239503588078 ) ) ;
#1406=CARTESIAN_POINT ( 'NONE',  ( -11.24191166894635074, 82.34025985790688651, -1.523999999999999799 ) ) ;
#1407=ADVANCED_FACE ( 'NONE', ( #39281 ), #32891, .T. ) ;
#1409=EDGE_CURVE ( 'NONE', #15145, #13978, #34982, .T. ) ;
#1413=CARTESIAN_POINT ( 'NONE',  ( -47.19240717248688810, 20.04893757306798108, -5.078271723505031865 ) ) ;
#1414=AXIS2_PLACEMENT_3D ( 'NONE', #34555, #28573, #25376 ) ;
#1415=DIRECTION ( 'NONE',  ( 0.4849315768086426282, 0.8745520943968310146, 1.030032898892908135E-16 ) ) ;
#1416=CARTESIAN_POINT ( 'NONE',  ( -57.99953387342350908, 0.4830015814202143209, 0.7353922615980046373 ) ) ;
#1419=CARTESIAN_POINT ( 'NONE',  ( -46.81215924274956564, 25.79096025118141711, -0.6894041771339123326 ) ) ;
#1421=LINE ( 'NONE', #23334, #36691 ) ;
#1430=EDGE_LOOP ( 'NONE', ( #22979, #36119, #20047, #567 ) ) ;
#1439=CARTESIAN_POINT ( 'NONE',  ( -55.57144106515218596, 6.156191000079303421, -3.024401744048434537 ) ) ;
#1443=AXIS2_PLACEMENT_3D ( 'NONE', #3067, #22198, #38835 ) ;
#1444=ORIENTED_EDGE ( 'NONE', *, *, #38421, .F. ) ;
#1445=EDGE_CURVE ( 'NONE', #38820, #27671, #9640, .T. ) ;
#1449=CIRCLE ( 'NONE', #38837, 0.6349999999999998979 ) ;
#1450=DIRECTION ( 'NONE',  ( 0.8745520943968240202, -0.4849315768086551182, 4.268512490100404500E-16 ) ) ;
#1452=ORIENTED_EDGE ( 'NONE', *, *, #7804, .T. ) ;
#1455=DIRECTION ( 'NONE',  ( 0.8745520943968240202, -0.4849315768086553402, 6.829619984160650158E-16 ) ) ;
#1462=CARTESIAN_POINT ( 'NONE',  ( -6.318938770521974391, 64.36956080246774548, -1.523999999999994026 ) ) ;
#1464=CARTESIAN_POINT ( 'NONE',  ( -57.72392508873495842, 1.101746749479270093, 1.179667423805870863 ) ) ;
#1467=CARTESIAN_POINT ( 'NONE',  ( -57.09878488423309051, 3.216020309495956742, 2.217633722229532367 ) ) ;
#1468=CARTESIAN_POINT ( 'NONE',  ( -58.46978370654361612, 0.04540555296617620334, 0.7440089614489153735 ) ) ;
#1471=ORIENTED_EDGE ( 'NONE', *, *, #3988, .T. ) ;
#1472=CARTESIAN_POINT ( 'NONE',  ( -53.45432727069204759, 10.77832982246877691, 4.078803160923774485 ) ) ;
#1475=AXIS2_PLACEMENT_3D ( 'NONE', #28043, #11863, #37848 ) ;
#1484=CARTESIAN_POINT ( 'NONE',  ( -47.20408514806452871, 20.03888983422028502, 5.082056583517504222 ) ) ;
#1497=ORIENTED_EDGE ( 'NONE', *, *, #31314, .F. ) ;
#1498=CARTESIAN_POINT ( 'NONE',  ( -48.46138709710082537, 15.22468166490328123, 0.8008350491754776534 ) ) ;
#1503=VERTEX_POINT ( 'NONE', #6481 ) ;
#1504=AXIS2_PLACEMENT_3D ( 'NONE', #20658, #4506, #4090 ) ;
#1506=VECTOR ( 'NONE', #13715, 1000.000000000000227 ) ;
#1515=ADVANCED_FACE ( 'NONE', ( #108 ), #22221, .F. ) ;
#1518=EDGE_CURVE ( 'NONE', #22436, #1811, #13071, .T. ) ;
#1524=ORIENTED_EDGE ( 'NONE', *, *, #34009, .T. ) ;
#1534=CARTESIAN_POINT ( 'NONE',  ( -26.29578028364076658, 73.87584665086983193, -1.270000000000006013 ) ) ;
#1539=ORIENTED_EDGE ( 'NONE', *, *, #17162, .F. ) ;
#1546=ORIENTED_EDGE ( 'NONE', *, *, #5800, .T. ) ;
#1547=PLANE ( 'NONE',  #437 ) ;
#1549=( NAMED_UNIT ( * ) PLANE_ANGLE_UNIT ( ) SI_UNIT ( $, .RADIAN. ) );
#1555=DIRECTION ( 'NONE',  ( -5.188838149069471174E-16, 1.699382548006136313E-16, 1.000000000000000000 ) ) ;
#1556=ORIENTED_EDGE ( 'NONE', *, *, #39881, .F. ) ;
#1562=AXIS2_PLACEMENT_3D ( 'NONE', #13972, #19565, #32574 ) ;
#1563=B_SPLINE_CURVE_WITH_KNOTS ( 'NONE', 3,
 ( #10718, #23699, #40136, #8160, #30110, #11351, #33317, #10515, #17322, #26708 ),
 .UNSPECIFIED., .F., .F.,
 ( 4, 2, 2, 2, 4 ),
 ( -5.999999993416881897E-08, 0.0003259810225990044091, 0.0006520220451979429760, 0.0009780630677968815429, 0.001304104090395820110 ),
 .UNSPECIFIED. ) ;
#1564=CARTESIAN_POINT ( 'NONE',  ( -58.03077483564787542, 0.4858688437074938915, 1.087158688094367331 ) ) ;
#1565=EDGE_CURVE ( 'NONE', #17342, #3974, #14232, .T. ) ;
#1572=CARTESIAN_POINT ( 'NONE',  ( -46.89809204272969367, 25.37679221950173059, 1.718882409580913651 ) ) ;
#1574=CARTESIAN_POINT ( 'NONE',  ( -57.95665747882670615, 0.5159457608236717174, -0.4254811051331304217 ) ) ;
#1577=DIRECTION ( 'NONE',  ( -0.8745520943968240202, 0.4849315768086552292, -5.361993529360572958E-16 ) ) ;
#1579=CARTESIAN_POINT ( 'NONE',  ( -30.15519950990045572, 69.97033940222175374, 1.269999999999991802 ) ) ;
#1581=DIRECTION ( 'NONE',  ( -0.9998501190848635423, -0.01731298258487451447, -5.158639060800523934E-16 ) ) ;
#1582=CARTESIAN_POINT ( 'NONE',  ( -58.64217253742437208, 0.4108157498741576985, 0.3978973257256460672 ) ) ;
#1583=CARTESIAN_POINT ( 'NONE',  ( -58.83227707057486811, -0.08366279997995551554, 0.2458995907044889129 ) ) ;
#1586=CARTESIAN_POINT ( 'NONE',  ( -57.38748718130355542, 3.645894598607590797, -1.236217348619478962 ) ) ;
#1587=ORIENTED_EDGE ( 'NONE', *, *, #19393, .F. ) ;
#1588=CARTESIAN_POINT ( 'NONE',  ( -46.82131867383202461, 20.47688106639290240, -5.000304862135876327 ) ) ;
#1589=COLOUR_RGB ( '', 0.40784314, 0.44705882, 0.49803922) ;
#1593=AXIS2_PLACEMENT_3D ( 'NONE', #22972, #442, #9584 ) ;
#1597=CARTESIAN_POINT ( 'NONE',  ( -49.86239633785145742, 16.51455008844218142, -4.953957629277327968 ) ) ;
#1601=CARTESIAN_POINT ( 'NONE',  ( -56.19876127534764265, 4.345455792799514327, -2.342364202820239605 ) ) ;
#1602=ADVANCED_FACE ( 'NONE', ( #39921 ), #27543, .T. ) ;
#1605=CARTESIAN_POINT ( 'NONE',  ( -42.72397600927682504, 22.83316142988638831, -1.683267422954632275 ) ) ;
#1606=AXIS2_PLACEMENT_3D ( 'NONE', #21223, #5083, #8678 ) ;
#1612=ADVANCED_FACE ( 'NONE', ( #13711 ), #18615, .T. ) ;
#1613=CARTESIAN_POINT ( 'NONE',  ( -56.26318288983030413, 4.268071985104968213, -2.480832006587858185 ) ) ;
#1617=AXIS2_PLACEMENT_3D ( 'NONE', #36632, #26828, #1065 ) ;
#1621=CARTESIAN_POINT ( 'NONE',  ( -11.56352105402813280, 78.55269139521317356, 1.524000000000000465 ) ) ;
#1622=ADVANCED_FACE ( 'NONE', ( #20714 ), #3696, .T. ) ;
#1623=CARTESIAN_POINT ( 'NONE',  ( -42.12253153191132782, 21.94389511927449732, -0.09363185731631336328 ) ) ;
#1625=AXIS2_PLACEMENT_3D ( 'NONE', #5659, #18189, #2460 ) ;
#1626=CARTESIAN_POINT ( 'NONE',  ( -58.32289719230551839, -0.2069853552843642364, 0.1059582036190176574 ) ) ;
#1629=CARTESIAN_POINT ( 'NONE',  ( -46.93527007713159804, 25.91000514300129254, -0.2210822239326209193 ) ) ;
#1632=CIRCLE ( 'NONE', #4390, 0.7620000000000015650 ) ;
#1643=EDGE_CURVE ( 'NONE', #39553, #22515, #28148, .T. ) ;
#1645=CARTESIAN_POINT ( 'NONE',  ( -44.11963993135361051, 21.57970632322487958, -2.906001689204277927 ) ) ;
#1649=CARTESIAN_POINT ( 'NONE',  ( -6.422645615570758970, 77.88548590848095898, 1.524000000000002908 ) ) ;
#1651=CARTESIAN_POINT ( 'NONE',  ( -55.98935619762070104, 5.304184903340836144, -2.807757416349843549 ) ) ;
#1653=CIRCLE ( 'NONE', #9766, 9.048750000000000071 ) ;
#1657=ORIENTED_EDGE ( 'NONE', *, *, #41794, .F. ) ;
#1663=ORIENTED_EDGE ( 'NONE', *, *, #4742, .F. ) ;
#1665=DIRECTION ( 'NONE',  ( -0.4849315768086535083, -0.8745520943968250194, -1.030032898892974695E-16 ) ) ;
#1666=AXIS2_PLACEMENT_3D ( 'NONE', #32390, #6830, #3222 ) ;
#1667=FACE_OUTER_BOUND ( 'NONE', #41630, .T. ) ;
#1672=ADVANCED_FACE ( 'NONE', ( #40343 ), #3935, .T. ) ;
#1676=CARTESIAN_POINT ( 'NONE',  ( -57.32388393874000343, 1.962507715601113034, 1.551164999238653142 ) ) ;
#1677=CARTESIAN_POINT ( 'NONE',  ( -56.40362312693983426, 4.444843175407298119, 2.562861284854979882 ) ) ;
#1681=EDGE_LOOP ( 'NONE', ( #10008, #19257, #555, #25784 ) ) ;
#1682=EDGE_CURVE ( 'NONE', #27418, #37655, #29897, .T. ) ;
#1683=CARTESIAN_POINT ( 'NONE',  ( -50.58884987432006852, 15.93229845861179861, 5.010371253631904942 ) ) ;
#1690=VERTEX_POINT ( 'NONE', #36715 ) ;
#1693=DIRECTION ( 'NONE',  ( -0.8745520943968246863, 0.4849315768086538414, -5.122214988120500191E-16 ) ) ;
#1694=CARTESIAN_POINT ( 'NONE',  ( -44.81960200544693151, 21.09415034428922908, 3.442746975522605002 ) ) ;
#1697=DIRECTION ( 'NONE',  ( -0.8745520943968301264, 0.4849315768086440159, -5.271987356194192020E-16 ) ) ;
#1705=ADVANCED_FACE ( 'NONE', ( #7327 ), #7648, .T. ) ;
#1708=CARTESIAN_POINT ( 'NONE',  ( -47.79679003974130325, 17.22715854250130718, 2.282645788202369186 ) ) ;
#1718=EDGE_LOOP ( 'NONE', ( #13114, #32605, #28225, #34544 ) ) ;
#1725=FACE_OUTER_BOUND ( 'NONE', #7264, .T. ) ;
#1751=ORIENTED_EDGE ( 'NONE', *, *, #28742, .F. ) ;
#1753=DIRECTION ( 'NONE',  ( -0.3582377630123937395, 0.9336303900108844367, -1.442042072394378310E-15 ) ) ;
#1757=CARTESIAN_POINT ( 'NONE',  ( -42.67774669360623108, 22.12976309729135593, 1.921043817380094332 ) ) ;
#1761=DIRECTION ( 'NONE',  ( -0.6294287539884059202, -0.7770581983690814099, -1.945484789722797322E-16 ) ) ;
#1762=ORIENTED_EDGE ( 'NONE', *, *, #691, .F. ) ;
#1765=ORIENTED_EDGE ( 'NONE', *, *, #33196, .F. ) ;
#1768=CARTESIAN_POINT ( 'NONE',  ( -58.07568876781240164, 0.3868594689447146795, 1.028118745743028084 ) ) ;
#1777=CARTESIAN_POINT ( 'NONE',  ( -57.24575050778504703, 1.871741192705528301, -0.5496743666259116257 ) ) ;
#1780=DIRECTION ( 'NONE',  ( 0.9807655518882886225, -0.1951894777626621558, 5.420735302995426205E-16 ) ) ;
#1781=DIRECTION ( 'NONE',  ( 5.188838149069472160E-16, -1.699382548006136559E-16, -1.000000000000000000 ) ) ;
#1782=CARTESIAN_POINT ( 'NONE',  ( -7.994219716368544226, 68.36415334912796027, 1.270000000000003570 ) ) ;
#1783=DIRECTION ( 'NONE',  ( -0.8745520943968241312, 0.4849315768086548406, -5.691349986800536046E-16 ) ) ;
#1786=CARTESIAN_POINT ( 'NONE',  ( -7.868930244179279221, 69.75330307926518003, 1.270000000000003348 ) ) ;
#1791=CARTESIAN_POINT ( 'NONE',  ( -58.55612285180487930, 0.6590214021355705887, -0.05016670522519821318 ) ) ;
#1792=ORIENTED_EDGE ( 'NONE', *, *, #37372, .F. ) ;
#1793=CARTESIAN_POINT ( 'NONE',  ( -44.83891394770831340, 21.39113109692858217, -3.507332325250104965 ) ) ;
#1800=CARTESIAN_POINT ( 'NONE',  ( -51.28922332432183140, 14.16478490540409219, -4.617129769900083502 ) ) ;
#1801=ORIENTED_EDGE ( 'NONE', *, *, #16774, .F. ) ;
#1804=DIRECTION ( 'NONE',  ( 0.9998501190848635423, 0.01731298258487451447, 5.158639060800523934E-16 ) ) ;
#1806=CARTESIAN_POINT ( 'NONE',  ( -49.36007427823454918, 17.22477551487747149, -4.982732351148011496 ) ) ;
#1809=CARTESIAN_POINT ( 'NONE',  ( -48.56815661899837977, 19.24492339269602681, -5.224590812749990931 ) ) ;
#1811=VERTEX_POINT ( 'NONE', #24333 ) ;
#1815=CARTESIAN_POINT ( 'NONE',  ( -57.29531047346088712, 2.067549486662559222, -1.749273462387503031 ) ) ;
#1818=CARTESIAN_POINT ( 'NONE',  ( -5.924740142096584172, 65.21691166894066782, -1.269999999999994023 ) ) ;
#1821=CARTESIAN_POINT ( 'NONE',  ( -57.52317756609133426, 3.014644041894651405, -1.981665235817958948 ) ) ;
#1822=AXIS2_PLACEMENT_3D ( 'NONE', #36149, #6534, #19301 ) ;
#1823=CARTESIAN_POINT ( 'NONE',  ( -44.02811856515548783, 21.20684991433588351, -2.650346054289419495 ) ) ;
#1826=FACE_OUTER_BOUND ( 'NONE', #41958, .T. ) ;
#1827=CARTESIAN_POINT ( 'NONE',  ( -58.37241122568488549, -0.2962816677227891882, -1.036115889661433750E-14 ) ) ;
#1828=CARTESIAN_POINT ( 'NONE',  ( -51.10637697011796377, 21.44594517096482633, -9.676659029908143380E-15 ) ) ;
#1831=CARTESIAN_POINT ( 'NONE',  ( -47.66286930719411430, 20.62480072838431155, -5.054501799269508489 ) ) ;
#1847=ORIENTED_EDGE ( 'NONE', *, *, #4341, .T. ) ;
#1849=EDGE_LOOP ( 'NONE', ( #16707, #10753, #3320, #6175 ) ) ;
#1851=DIRECTION ( 'NONE',  ( -5.188838149069472160E-16, 1.699382548006136559E-16, 1.000000000000000000 ) ) ;
#1853=CARTESIAN_POINT ( 'NONE',  ( -58.63691926683795685, -0.7730888055834101991, -0.03927874230347657564 ) ) ;
#1859=VERTEX_POINT ( 'NONE', #31361 ) ;
#1860=CIRCLE ( 'NONE', #30417, 0.2540000000000013358 ) ;
#1868=DIRECTION ( 'NONE',  ( 0.9454731675810352787, -0.3256999990547799206, 8.013021739297562628E-15 ) ) ;
#1877=CARTESIAN_POINT ( 'NONE',  ( -58.30132030250355513, -0.1468297825097129305, 0.3337338984326744251 ) ) ;
#1882=AXIS2_PLACEMENT_3D ( 'NONE', #15387, #11358, #24546 ) ;
#1884=CARTESIAN_POINT ( 'NONE',  ( -52.26939619200407350, 13.58078015197115818, 4.476849201000069556 ) ) ;
#1889=DIRECTION ( 'NONE',  ( -0.3582377630123937950, 0.9336303900108844367, -3.445432962228676930E-16 ) ) ;
#1896=DIRECTION ( 'NONE',  ( 0.3582377630123966261, -0.9336303900108832154, 0.000000000000000000 ) ) ;
#1897=DIRECTION ( 'NONE',  ( -5.188838149069471174E-16, 1.699382548006136313E-16, 1.000000000000000000 ) ) ;
#1899=DIRECTION ( 'NONE',  ( -0.7770581983690837413, 0.6294287539884032556, -5.101669463485834765E-16 ) ) ;
#1911=CARTESIAN_POINT ( 'NONE',  ( -50.02669608763528686, 12.78473261814649931, -8.015744983012485712E-15 ) ) ;
#1925=EDGE_CURVE ( 'NONE', #11774, #22436, #31578, .T. ) ;
#1928=EDGE_CURVE ( 'NONE', #37721, #4510, #36907, .T. ) ;
#1934=DIRECTION ( 'NONE',  ( 5.188838149069471174E-16, -1.699382548006136313E-16, -1.000000000000000000 ) ) ;
#1937=ORIENTED_EDGE ( 'NONE', *, *, #8400, .F. ) ;
#1938=CYLINDRICAL_SURFACE ( 'NONE', #11847, 0.5080000000000000071 ) ;
#1944=CARTESIAN_POINT ( 'NONE',  ( -10.73808814597608574, 77.14487411131504757, -1.523999999999998467 ) ) ;
#1945=FACE_OUTER_BOUND ( 'NONE', #41913, .T. ) ;
#1946=DIRECTION ( 'NONE',  ( -0.8745520943968243532, 0.4849315768086547296, -6.829619984160642269E-16 ) ) ;
#1952=EDGE_LOOP ( 'NONE', ( #3276, #12265, #13796, #35170 ) ) ;
#1958=ORIENTED_EDGE ( 'NONE', *, *, #31551, .T. ) ;
#1959=ORIENTED_EDGE ( 'NONE', *, *, #28804, .T. ) ;
#1960=DIRECTION ( 'NONE',  ( -0.4849315768086426282, -0.8745520943968310146, -1.030032898892908135E-16 ) ) ;
#1971=ADVANCED_FACE ( 'NONE', ( #38187 ), #8579, .F. ) ;
#1974=CIRCLE ( 'NONE', #6741, 0.7620000000000015650 ) ;
#1975=VECTOR ( 'NONE', #16197, 1000.000000000000000 ) ;
#1977=CARTESIAN_POINT ( 'NONE',  ( -58.42460811326324688, -0.3780437665152627247, 0.3615838660048876774 ) ) ;
#1985=EDGE_CURVE ( 'NONE', #25154, #18870, #41173, .T. ) ;
#1987=CARTESIAN_POINT ( 'NONE',  ( -57.48728866487982714, 1.341405240446180702, -0.2210608495301590037 ) ) ;
#1989=CYLINDRICAL_SURFACE ( 'NONE', #14889, 0.2539999999999996705 ) ;
#1990=CARTESIAN_POINT ( 'NONE',  ( -14.53564353655538177, 79.78436006922240153, 1.269999999999997353 ) ) ;
#1997=EDGE_LOOP ( 'NONE', ( #2346, #1937, #13889, #16961 ) ) ;
#1998=CARTESIAN_POINT ( 'NONE',  ( -58.50860430493788300, 0.7049166599848583070, -0.9756837515128594651 ) ) ;
#2001=VERTEX_POINT ( 'NONE', #41389 ) ;
#2002=CARTESIAN_POINT ( 'NONE',  ( -47.72307967018490871, 19.52623448395591765, -5.191226814325721861 ) ) ;
#2009=CARTESIAN_POINT ( 'NONE',  ( -49.81232696645592029, 16.59374381583211999, -4.964399749387115257 ) ) ;
#2010=VERTEX_POINT ( 'NONE', #21971 ) ;
#2014=CARTESIAN_POINT ( 'NONE',  ( -56.75031417288079183, 3.184683474932036518, -1.986967496122973520 ) ) ;
#2017=CARTESIAN_POINT ( 'NONE',  ( -49.19743978460682143, 17.65503563884207594, -5.190924102448302158 ) ) ;
#2019=ORIENTED_EDGE ( 'NONE', *, *, #35051, .F. ) ;
#2023=CARTESIAN_POINT ( 'NONE',  ( -58.10099831372669854, 0.3475205698689753930, -0.9728495803591354907 ) ) ;
#2024=CIRCLE ( 'NONE', #10859, 0.2540000000000017799 ) ;
#2028=ADVANCED_FACE ( 'NONE', ( #12194 ), #33502, .T. ) ;
#2029=TOROIDAL_SURFACE ( 'NONE', #21730, 0.3810000000000014486, 0.2540000000000000036 ) ;
#2030=ADVANCED_FACE ( 'NONE', ( #40961 ), #17939, .T. ) ;
#2034=CARTESIAN_POINT ( 'NONE',  ( -44.40685758373553682, 19.43703734468912714, -0.2085933842879179878 ) ) ;
#2035=ORIENTED_EDGE ( 'NONE', *, *, #39593, .F. ) ;
#2036=DIRECTION ( 'NONE',  ( 0.9336303900108808840, 0.3582377630124026768, -4.808225039248730429E-15 ) ) ;
#2037=CARTESIAN_POINT ( 'NONE',  ( -57.47393550255000605, 1.325481720219651161, 0.09114234605507165465 ) ) ;
#2038=CARTESIAN_POINT ( 'NONE',  ( -52.43464216547582879, 18.97776253636583732, -1.004568992552039040E-14 ) ) ;
#2040=ORIENTED_EDGE ( 'NONE', *, *, #27411, .T. ) ;
#2041=CARTESIAN_POINT ( 'NONE',  ( -49.70354115100154502, 23.42381831551578486, -0.3024929150989502658 ) ) ;
#2062=CARTESIAN_POINT ( 'NONE',  ( -55.76611385812176280, 5.250064693407995975, -2.603441191291675949 ) ) ;
#2068=EDGE_LOOP ( 'NONE', ( #28107, #7520, #34020, #14291 ) ) ;
#2072=DIRECTION ( 'NONE',  ( 5.188838149069472160E-16, -1.699382548006136559E-16, -1.000000000000000000 ) ) ;
#2073=CARTESIAN_POINT ( 'NONE',  ( -8.480639930781094904, 68.51064353654967931, -1.269999999999995799 ) ) ;
#2076=DIRECTION ( 'NONE',  ( -0.9998501190848638753, -0.01731298258485278532, -8.537024980200814916E-16 ) ) ;
#2077=TOROIDAL_SURFACE ( 'NONE', #9541, 0.3809999999999990616, 0.2540000000000000036 ) ;
#2086=CARTESIAN_POINT ( 'NONE',  ( -58.36801712489022975, -0.2878572300611665358, 0.05073317217019857051 ) ) ;
#2087=FACE_OUTER_BOUND ( 'NONE', #40476, .T. ) ;
#2089=CYLINDRICAL_SURFACE ( 'NONE', #4237, 0.2539999999999942859 ) ;
#2093=CARTESIAN_POINT ( 'NONE',  ( -54.34142964503966056, 9.837102586603037935, 3.694930414371496052 ) ) ;
#2099=VECTOR ( 'NONE', #41623, 1000.000000000000000 ) ;
#2103=CARTESIAN_POINT ( 'NONE',  ( -32.35039025330549123, 51.35812770460057664, 1.523999999999994248 ) ) ;
#2104=CARTESIAN_POINT ( 'NONE',  ( -10.39456080247343905, 81.94606122948148652, -1.269999999999998908 ) ) ;
#2105=DIRECTION ( 'NONE',  ( 0.8745520943968249084, -0.4849315768086533418, 5.271987356194193006E-16 ) ) ;
#2118=ORIENTED_EDGE ( 'NONE', *, *, #37313, .T. ) ;
#2119=CARTESIAN_POINT ( 'NONE',  ( -57.38720131040756200, 1.641502911523470942, 0.7119259365333153733 ) ) ;
#2121=ADVANCED_FACE ( 'NONE', ( #27744 ), #4254, .T. ) ;
#2124=EDGE_LOOP ( 'NONE', ( #28766, #34062, #4168, #38468 ) ) ;
#2127=EDGE_CURVE ( 'NONE', #34427, #9964, #34360, .T. ) ;
#2129=VERTEX_POINT ( 'NONE', #1990 ) ;
#2131=DIRECTION ( 'NONE',  ( -0.8745520943968253524, 0.4849315768086530087, -8.537024980200771528E-16 ) ) ;
#2142=EDGE_CURVE ( 'NONE', #11267, #28559, #22172, .T. ) ;
#2144=ORIENTED_EDGE ( 'NONE', *, *, #14403, .F. ) ;
#2160=EDGE_CURVE ( 'NONE', #15671, #35981, #41599, .T. ) ;
#2171=ADVANCED_FACE ( 'NONE', ( #9830 ), #42101, .T. ) ;
#2173=ORIENTED_EDGE ( 'NONE', *, *, #33952, .F. ) ;
#2180=AXIS2_PLACEMENT_3D ( 'NONE', #28788, #35189, #38591 ) ;
#2182=CARTESIAN_POINT ( 'NONE',  ( -5.580495364573205386, 77.10007210032874525, -1.269999999999995799 ) ) ;
#2183=EDGE_CURVE ( 'NONE', #2010, #24767, #25067, .T. ) ;
#2192=CARTESIAN_POINT ( 'NONE',  ( -52.02227077088271301, 12.92666902008283358, 4.429676403336999968 ) ) ;
#2197=TOROIDAL_SURFACE ( 'NONE', #25981, 0.7620000000000000107, 0.2540000000000000036 ) ;
#2201=CARTESIAN_POINT ( 'NONE',  ( -57.94149553976682654, 0.5275954726333825784, -0.3053296928521576636 ) ) ;
#2208=CARTESIAN_POINT ( 'NONE',  ( -23.43300365160792964, 82.12916405548841681, -1.270000000000006013 ) ) ;
#2214=CARTESIAN_POINT ( 'NONE',  ( -58.83227707057485389, -0.08366279997994163775, -5.798466560119647675E-15 ) ) ;
#2224=CARTESIAN_POINT ( 'NONE',  ( -52.46109226273545545, 12.10756162195068875, -4.274556252865695072 ) ) ;
#2229=CARTESIAN_POINT ( 'NONE',  ( -53.71463501147313480, 9.386209292303481888, -3.577838831676722009 ) ) ;
#2230=EDGE_CURVE ( 'NONE', #40395, #23452, #12158, .T. ) ;
#2233=CARTESIAN_POINT ( 'NONE',  ( -55.41603145274652320, 6.826612083464994818, -3.210495615568592420 ) ) ;
#2241=CARTESIAN_POINT ( 'NONE',  ( -58.73801720703743001, -0.4998429216807459552, -0.2437502737749605297 ) ) ;
#2243=CARTESIAN_POINT ( 'NONE',  ( -33.42971872652992005, 49.93539301574497102, -1.270000000000005569 ) ) ;
#2245=FACE_OUTER_BOUND ( 'NONE', #28960, .T. ) ;
#2249=CARTESIAN_POINT ( 'NONE',  ( -36.43259636504752308, 28.15155085495446485, 1.269999999999995799 ) ) ;
#2251=CARTESIAN_POINT ( 'NONE',  ( -57.92346726745822849, 0.7446056814934959300, 1.206286704679851107 ) ) ;
#2253=VECTOR ( 'NONE', #36473, 1000.000000000000114 ) ;
#2254=DIRECTION ( 'NONE',  ( -0.8745520943968243532, 0.4849315768086547296, -6.829619984160642269E-16 ) ) ;
#2255=CARTESIAN_POINT ( 'NONE',  ( -51.10637696787394191, 21.44594517334857287, 0.3731469903906310948 ) ) ;
#2258=CARTESIAN_POINT ( 'NONE',  ( -48.45250714818473625, 19.88962760504932348, -4.734234960886007926 ) ) ;
#2261=ORIENTED_EDGE ( 'NONE', *, *, #21856, .F. ) ;
#2270=FACE_OUTER_BOUND ( 'NONE', #16307, .T. ) ;
#2273=CARTESIAN_POINT ( 'NONE',  ( -41.09676540851935300, 23.04694042099051998, -1.524000000000031996 ) ) ;
#2275=VERTEX_POINT ( 'NONE', #2833 ) ;
#2277=DIRECTION ( 'NONE',  ( 5.188838149069472160E-16, -1.699382548006136559E-16, -1.000000000000000000 ) ) ;
#2288=CIRCLE ( 'NONE', #26061, 0.3810000000000000053 ) ;
#2289=CARTESIAN_POINT ( 'NONE',  ( -7.994219716368544226, 68.36415334912796027, -1.523999999999995580 ) ) ;
#2292=ORIENTED_EDGE ( 'NONE', *, *, #26205, .F. ) ;
#2294=CARTESIAN_POINT ( 'NONE',  ( -13.99440778436217592, 79.95103047660883533, 1.523999999999998023 ) ) ;
#2300=CARTESIAN_POINT ( 'NONE',  ( -41.97746338594183868, 23.60773098774231826, -1.524000000000005794 ) ) ;
#2303=CARTESIAN_POINT ( 'NONE',  ( -58.12591287054759448, 0.2317919070111071345, 0.6797015115164672938 ) ) ;
#2305=DIRECTION ( 'NONE',  ( 0.9876665170007968841, -0.1565721916417945614, 5.390917751951445902E-16 ) ) ;
#2308=EDGE_LOOP ( 'NONE', ( #25105, #6406, #17355, #34621 ) ) ;
#2309=CARTESIAN_POINT ( 'NONE',  ( -52.50198181065980663, 11.96455506022023307, 4.263607785004571937 ) ) ;
#2315=FACE_OUTER_BOUND ( 'NONE', #3086, .T. ) ;
#2316=VERTEX_POINT ( 'NONE', #3043 ) ;
#2318=CARTESIAN_POINT ( 'NONE',  ( -29.61277755908112042, 68.29894143245043381, 1.523999999991891618 ) ) ;
#2320=CARTESIAN_POINT ( 'NONE',  ( -8.313969523394650452, 67.96940778435646280, -1.269999999999995355 ) ) ;
#2321=AXIS2_PLACEMENT_3D ( 'NONE', #12658, #26490, #15841 ) ;
#2322=CARTESIAN_POINT ( 'NONE',  ( -41.06680163122278060, 23.07855206975584395, 1.270000052244668831 ) ) ;
#2332=AXIS2_PLACEMENT_3D ( 'NONE', #33270, #26866, #7494 ) ;
#2335=CARTESIAN_POINT ( 'NONE',  ( -57.28860081656939229, 2.041040056096066202, 1.590330371070447946 ) ) ;
#2339=AXIS2_PLACEMENT_3D ( 'NONE', #14743, #20499, #27118 ) ;
#2343=EDGE_LOOP ( 'NONE', ( #20259, #24315, #40824, #35579 ) ) ;
#2346=ORIENTED_EDGE ( 'NONE', *, *, #13172, .T. ) ;
#2351=CARTESIAN_POINT ( 'NONE',  ( -17.14500000000466784, 71.11999999999886768, -1.524000000000000909 ) ) ;
#2356=CARTESIAN_POINT ( 'NONE',  ( -16.46263872254443683, 83.91929436251373886, -1.524000000000002464 ) ) ;
#2368=CARTESIAN_POINT ( 'NONE',  ( -58.07447437077728125, 1.735896131820596766, 1.499107834811089557 ) ) ;
#2385=EDGE_CURVE ( 'NONE', #24894, #11397, #1295, .T. ) ;
#2386=ORIENTED_EDGE ( 'NONE', *, *, #21078, .T. ) ;
#2388=DIRECTION ( 'NONE',  ( -0.9876665170007968841, 0.1565721916417935344, -5.390917751951443929E-16 ) ) ;
#2399=ORIENTED_EDGE ( 'NONE', *, *, #29542, .F. ) ;
#2401=DIRECTION ( 'NONE',  ( -0.6559537821943223213, 0.7548010569845299278, -8.537024980200762654E-16 ) ) ;
#2403=CARTESIAN_POINT ( 'NONE',  ( -58.30061145522722654, -0.1075020354536087575, 0.6732717543611356215 ) ) ;
#2414=CARTESIAN_POINT ( 'NONE',  ( -56.89020484191215132, 2.444072280526621288, -0.3054065742134425832 ) ) ;
#2418=DIRECTION ( 'NONE',  ( 5.188838149069472160E-16, -1.699382548006136559E-16, -1.000000000000000000 ) ) ;
#2422=CARTESIAN_POINT ( 'NONE',  ( -28.60507221318228943, 76.72702915747851193, 1.523999999999991806 ) ) ;
#2426=CARTESIAN_POINT ( 'NONE',  ( -58.75091225067960465, 0.1325880516401256592, -0.03773457465075338857 ) ) ;
#2427=ORIENTED_EDGE ( 'NONE', *, *, #7427, .T. ) ;
#2428=CARTESIAN_POINT ( 'NONE',  ( -41.28107547821695533, 23.22158991241120063, -1.524000000000005794 ) ) ;
#2434=EDGE_CURVE ( 'NONE', #33959, #31070, #23011, .T. ) ;
#2436=CARTESIAN_POINT ( 'NONE',  ( -55.85087417899054429, 5.582623226463158339, -2.873287190156892379 ) ) ;
#2439=CARTESIAN_POINT ( 'NONE',  ( -4.466782427718574588, 71.06098887363195615, 1.270000000000004903 ) ) ;
#2442=CARTESIAN_POINT ( 'NONE',  ( -53.77126677436539381, 9.275061619689314085, -3.554206636766655159 ) ) ;
#2445=CARTESIAN_POINT ( 'NONE',  ( -53.65759266121656879, 11.01975743955735432, -4.003319250743225588 ) ) ;
#2446=EDGE_CURVE ( 'NONE', #33959, #30709, #40062, .T. ) ;
#2452=CARTESIAN_POINT ( 'NONE',  ( -58.43690671596436914, -0.4125963578781866037, -0.2423173958219211055 ) ) ;
#2455=CARTESIAN_POINT ( 'NONE',  ( -47.16908398257314872, 25.15707121737544938, 1.640988021989188805 ) ) ;
#2458=CARTESIAN_POINT ( 'NONE',  ( -58.83227707057486811, -0.08366279997995551554, -0.2458995907045101459 ) ) ;
#2460=DIRECTION ( 'NONE',  ( 0.8572391118119481179, 0.5149185422762151410, 0.000000000000000000 ) ) ;
#2461=VERTEX_POINT ( 'NONE', #15793 ) ;
#2463=CARTESIAN_POINT ( 'NONE',  ( -58.11258158571958177, 1.603013069906233934, 1.501710181103012465 ) ) ;
#2464=CARTESIAN_POINT ( 'NONE',  ( -48.96082574602279180, 17.89581470837939747, 5.125304694085289547 ) ) ;
#2468=CARTESIAN_POINT ( 'NONE',  ( -51.41777536269126614, 18.15702087101736595, 2.173118852594992045 ) ) ;
#2472=CARTESIAN_POINT ( 'NONE',  ( -50.64083583777225073, 22.17031204481727258, -0.3653657693499831605 ) ) ;
#2483=DIRECTION ( 'NONE',  ( -0.8745520943968250194, 0.4849315768086534528, -5.361993529360573944E-16 ) ) ;
#2486=CARTESIAN_POINT ( 'NONE',  ( -24.16603736854983708, 76.82831944025377879, 1.269999999999993801 ) ) ;
#2489=ORIENTED_EDGE ( 'NONE', *, *, #26047, .F. ) ;
#2503=CARTESIAN_POINT ( 'NONE',  ( -36.43259636504752308, 28.15155085495446485, -1.524000000000003352 ) ) ;
#2504=EDGE_CURVE ( 'NONE', #35500, #30610, #27110, .T. ) ;
#2505=VECTOR ( 'NONE', #1415, 1000.000000000000114 ) ;
#2506=ORIENTED_EDGE ( 'NONE', *, *, #18795, .T. ) ;
#2513=CARTESIAN_POINT ( 'NONE',  ( -41.18107378286554621, 22.95619949144852967, -1.523999999999998023 ) ) ;
#2515=DIRECTION ( 'NONE',  ( -5.188838149069472160E-16, 1.699382548006136559E-16, 1.000000000000000000 ) ) ;
#2516=CARTESIAN_POINT ( 'NONE',  ( -58.13732371667832410, 0.2071221698984457016, 0.6618190132251328128 ) ) ;
#2519=DIRECTION ( 'NONE',  ( -0.8745520943968243532, 0.4849315768086547296, -6.829619984160642269E-16 ) ) ;
#2522=ORIENTED_EDGE ( 'NONE', *, *, #33625, .T. ) ;
#2523=CARTESIAN_POINT ( 'NONE',  ( -58.50860430493789721, 0.7049166599848305514, 0.9756837515128383709 ) ) ;
#2526=CIRCLE ( 'NONE', #26406, 0.2540000000000013913 ) ;
#2528=CARTESIAN_POINT ( 'NONE',  ( -7.917360960270791281, 70.00264313970245666, 1.270000000000003348 ) ) ;
#2530=ORIENTED_EDGE ( 'NONE', *, *, #33905, .T. ) ;
#2532=CARTESIAN_POINT ( 'NONE',  ( -29.35321563035234149, 61.36487289460320227, 1.269999999999993801 ) ) ;
#2535=CIRCLE ( 'NONE', #502, 0.7620000000000015650 ) ;
#2536=CARTESIAN_POINT ( 'NONE',  ( -28.76494711669534610, 76.52965637509277030, -1.524000000000007793 ) ) ;
#2540=CARTESIAN_POINT ( 'NONE',  ( -26.42106975583004314, 72.48669692073261217, 1.269999999999993356 ) ) ;
#2548=CARTESIAN_POINT ( 'NONE',  ( -56.42052199906244425, 3.302738315264078128, 0.3606658556335657906 ) ) ;
#2552=ORIENTED_EDGE ( 'NONE', *, *, #20644, .F. ) ;
#2557=ORIENTED_EDGE ( 'NONE', *, *, #17066, .T. ) ;
#2563=VECTOR ( 'NONE', #17486, 1000.000000000000114 ) ;
#2565=DIRECTION ( 'NONE',  ( -0.8745520943968235761, 0.4849315768086558398, -5.691349986800547879E-16 ) ) ;
#2566=CARTESIAN_POINT ( 'NONE',  ( -46.93533292561973269, 25.16125026830412281, 1.870414060841448567 ) ) ;
#2570=CARTESIAN_POINT ( 'NONE',  ( -42.79661761208809168, 21.81806929429799879, 2.089873509012810882 ) ) ;
#2571=CARTESIAN_POINT ( 'NONE',  ( -20.79116009376201291, 79.67004825550966984, -1.524000000000004018 ) ) ;
#2573=ORIENTED_EDGE ( 'NONE', *, *, #27983, .T. ) ;
#2578=DIRECTION ( 'NONE',  ( -5.188838149069472160E-16, 1.699382548006136559E-16, 1.000000000000000000 ) ) ;
#2597=ORIENTED_EDGE ( 'NONE', *, *, #13418, .F. ) ;
#2598=EDGE_LOOP ( 'NONE', ( #15570, #5040, #12685, #2552 ) ) ;
#2607=LINE ( 'NONE', #15566, #39955 ) ;
#2611=ORIENTED_EDGE ( 'NONE', *, *, #26308, .F. ) ;
#2614=DIRECTION ( 'NONE',  ( 0.8745520943968240202, -0.4849315768086551182, 4.268512490100404500E-16 ) ) ;
#2615=CARTESIAN_POINT ( 'NONE',  ( -58.66375602224792374, -0.3143320623662654301, 0.3221285174457437228 ) ) ;
#2618=CARTESIAN_POINT ( 'NONE',  ( -13.79703500197642896, 79.79115557309579287, -1.524000000000000687 ) ) ;
#2621=CIRCLE ( 'NONE', #15417, 0.2539999999999967839 ) ;
#2627=DIRECTION ( 'NONE',  ( -0.6825627711659453256, -0.7308269722843194760, -2.299753143848296480E-16 ) ) ;
#2635=ORIENTED_EDGE ( 'NONE', *, *, #39644, .T. ) ;
#2636=CARTESIAN_POINT ( 'NONE',  ( -17.14500000000466784, 71.11999999999886768, -1.270000000000000684 ) ) ;
#2637=ORIENTED_EDGE ( 'NONE', *, *, #17533, .T. ) ;
#2644=CARTESIAN_POINT ( 'NONE',  ( -53.83244890055875231, 9.568295475555508744, -3.789950525193721109 ) ) ;
#2645=ORIENTED_EDGE ( 'NONE', *, *, #24067, .T. ) ;
#2650=VECTOR ( 'NONE', #16472, 1000.000000000000000 ) ;
#2652=VECTOR ( 'NONE', #2483, 1000.000000000000227 ) ;
#2654=CARTESIAN_POINT ( 'NONE',  ( -53.75224695799815322, 9.373383622779334345, -3.688627211158436392 ) ) ;
#2660=CARTESIAN_POINT ( 'NONE',  ( -58.11144429832075531, 0.1746852717545294142, -1.017628075538466478E-14 ) ) ;
#2664=ADVANCED_FACE ( 'NONE', ( #20872 ), #29642, .T. ) ;
#2667=CYLINDRICAL_SURFACE ( 'NONE', #3162, 0.2540000000000046665 ) ;
#2668=AXIS2_PLACEMENT_3D ( 'NONE', #38146, #31316, #11937 ) ;
#2669=CARTESIAN_POINT ( 'NONE',  ( -47.44699234454018466, 15.94620872345373108, -7.864955498886620583E-15 ) ) ;
#2670=VERTEX_POINT ( 'NONE', #11091 ) ;
#2673=CARTESIAN_POINT ( 'NONE',  ( -58.10099831372669854, 0.3475205698689753930, 0.9728495803591148405 ) ) ;
#2674=CARTESIAN_POINT ( 'NONE',  ( -54.68081972647571831, 7.927468599487359491, 3.439372298942311446 ) ) ;
#2675=CARTESIAN_POINT ( 'NONE',  ( -30.15519950990045572, 69.97033940222175374, -1.270000000000007123 ) ) ;
#2676=DIRECTION ( 'NONE',  ( -5.188838149069472160E-16, 1.699382548006136559E-16, 1.000000000000000000 ) ) ;
#2677=CARTESIAN_POINT ( 'NONE',  ( -50.15972161391663064, 17.13814111569222121, 4.955022299345066550 ) ) ;
#2680=ORIENTED_EDGE ( 'NONE', *, *, #14971, .F. ) ;
#2681=CARTESIAN_POINT ( 'NONE',  ( -47.97936104919185851, 23.38005451144316993, -1.568716696360817675 ) ) ;
#2683=CARTESIAN_POINT ( 'NONE',  ( -23.09297118196009890, 77.93920196072180318, 1.269999999999994023 ) ) ;
#2689=FACE_OUTER_BOUND ( 'NONE', #1162, .T. ) ;
#2700=CARTESIAN_POINT ( 'NONE',  ( -58.35383657723647843, -0.2581369473864316699, -0.1573926582942791197 ) ) ;
#2710=EDGE_CURVE ( 'NONE', #1116, #5222, #5495, .T. ) ;
#2716=EDGE_LOOP ( 'NONE', ( #13515, #30906, #40079, #3146, #16029 ) ) ;
#2725=CARTESIAN_POINT ( 'NONE',  ( -58.28013857485719029, -0.1013628303895854899, 0.3875891849807499567 ) ) ;
#2739=CARTESIAN_POINT ( 'NONE',  ( -31.57591258858714767, 52.94298397388165256, 1.523999999999994692 ) ) ;
#2741=CARTESIAN_POINT ( 'NONE',  ( -42.03620417734941839, 22.24401450883962639, 1.718184518069207245 ) ) ;
#2742=EDGE_CURVE ( 'NONE', #41570, #5222, #32715, .T. ) ;
#2743=CARTESIAN_POINT ( 'NONE',  ( -7.772068811996249771, 69.25462295839062676, -1.523999999999995580 ) ) ;
#2746=EDGE_CURVE ( 'NONE', #28854, #5531, #12951, .T. ) ;
#2755=CARTESIAN_POINT ( 'NONE',  ( -56.38098843839168950, 3.837951075127326916, 1.838241461164903612 ) ) ;
#2760=EDGE_CURVE ( 'NONE', #28898, #15081, #36787, .T. ) ;
#2765=FACE_OUTER_BOUND ( 'NONE', #13866, .T. ) ;
#2766=DIRECTION ( 'NONE',  ( -0.8745520943968240202, 0.4849315768086553402, -6.829619984160650158E-16 ) ) ;
#2770=DIRECTION ( 'NONE',  ( 5.188838149069472160E-16, -1.699382548006136559E-16, -1.000000000000000000 ) ) ;
#2775=CARTESIAN_POINT ( 'NONE',  ( -44.90991502375803890, 23.16658271142636139, 2.247441098035892981 ) ) ;
#2780=VERTEX_POINT ( 'NONE', #39543 ) ;
#2785=CARTESIAN_POINT ( 'NONE',  ( -53.77660785250559883, 21.61116079084608188, -1.167830173942146849E-14 ) ) ;
#2789=CARTESIAN_POINT ( 'NONE',  ( -17.64290547347870941, 83.78857423953914463, -1.270000000000003126 ) ) ;
#2797=ORIENTED_EDGE ( 'NONE', *, *, #37350, .T. ) ;
#2812=CARTESIAN_POINT ( 'NONE',  ( -17.76856900107737403, 61.81127730225986738, -1.269999999999999352 ) ) ;
#2813=CIRCLE ( 'NONE', #17073, 0.5080000000000000071 ) ;
#2814=EDGE_CURVE ( 'NONE', #9109, #8970, #573, .T. ) ;
#2818=ORIENTED_EDGE ( 'NONE', *, *, #28206, .T. ) ;
#2820=CARTESIAN_POINT ( 'NONE',  ( -8.723850037987370243, 68.58388863026053173, 1.270000000000003126 ) ) ;
#2821=CARTESIAN_POINT ( 'NONE',  ( -58.81784827865774190, -0.2724209480193806598, 0.09409996577156981568 ) ) ;
#2833=CARTESIAN_POINT ( 'NONE',  ( -11.73534362491071903, 82.73994711668952107, -1.269999999999999796 ) ) ;
#2837=CARTESIAN_POINT ( 'NONE',  ( -47.07934102874902749, 22.98505637820369429, -3.579966862081945145 ) ) ;
#2842=VERTEX_POINT ( 'NONE', #2243 ) ;
#2843=CARTESIAN_POINT ( 'NONE',  ( -10.53334313995851801, 65.32054992887103140, 1.270000000000002904 ) ) ;
#2844=ORIENTED_EDGE ( 'NONE', *, *, #17977, .F. ) ;
#2846=VECTOR ( 'NONE', #6322, 1000.000000000000000 ) ;
#2851=CARTESIAN_POINT ( 'NONE',  ( -53.72989673830909396, 9.763294051742398949, -3.829717019284551771 ) ) ;
#2853=CARTESIAN_POINT ( 'NONE',  ( -56.97096143714185246, 2.717004285893137805, -1.832255202883321443 ) ) ;
#2861=CARTESIAN_POINT ( 'NONE',  ( -55.60486134785667645, 7.243031971518515633, -3.140198620020504094 ) ) ;
#2864=ORIENTED_EDGE ( 'NONE', *, *, #3748, .F. ) ;
#2867=AXIS2_PLACEMENT_3D ( 'NONE', #22531, #29586, #12551 ) ;
#2875=CARTESIAN_POINT ( 'NONE',  ( -50.82551848962686591, 16.13924203555649228, -4.804203053272171786 ) ) ;
#2876=CARTESIAN_POINT ( 'NONE',  ( -47.14728576169839869, 19.79714445405676670, -4.666695388795785604 ) ) ;
#2878=CARTESIAN_POINT ( 'NONE',  ( -17.32429653712378936, 61.56493206124108042, -1.269999999999999130 ) ) ;
#2879=CARTESIAN_POINT ( 'NONE',  ( -46.68310778696854157, 26.02399849596702097, -1.327428962946700874 ) ) ;
#2880=CARTESIAN_POINT ( 'NONE',  ( -49.69646605450807186, 16.77610880525235970, 4.988286919712930256 ) ) ;
#2883=CARTESIAN_POINT ( 'NONE',  ( -57.80205714066466527, 2.371715784325115095, 1.753227392946289154 ) ) ;
#2885=EDGE_LOOP ( 'NONE', ( #25918, #9135, #41042, #16 ) ) ;
#2886=CARTESIAN_POINT ( 'NONE',  ( -50.36444701916330047, 17.30043933429478642, -4.508886934713599359 ) ) ;
#2889=CARTESIAN_POINT ( 'NONE',  ( -8.690931667554782081, 74.34623700195145091, -1.523999999999996913 ) ) ;
#2890=ORIENTED_EDGE ( 'NONE', *, *, #22006, .F. ) ;
#2896=AXIS2_PLACEMENT_3D ( 'NONE', #11932, #9169, #21293 ) ;
#2903=ORIENTED_EDGE ( 'NONE', *, *, #39425, .T. ) ;
#2906=DIRECTION ( 'NONE',  ( 0.7548010569845150508, 0.6559537821943391966, 0.000000000000000000 ) ) ;
#2913=CARTESIAN_POINT ( 'NONE',  ( -17.14500000000466784, 71.11999999999886768, 1.523999999999998689 ) ) ;
#2919=CARTESIAN_POINT ( 'NONE',  ( -43.49527490626578441, 22.26612824116996237, -2.150709692269579865 ) ) ;
#2923=CARTESIAN_POINT ( 'NONE',  ( -28.36525985791271154, 77.02308833105713859, -1.524000000000007571 ) ) ;
#2924=TOROIDAL_SURFACE ( 'NONE', #32831, 0.3810000000000001719, 0.2540000000000000036 ) ;
#2929=DIRECTION ( 'NONE',  ( -0.4849315768086535638, -0.8745520943968251304, -1.030032898892975065E-16 ) ) ;
#2931=AXIS2_PLACEMENT_3D ( 'NONE', #32096, #2929, #10142 ) ;
#2932=EDGE_CURVE ( 'NONE', #31858, #41583, #14310, .T. ) ;
#2938=CARTESIAN_POINT ( 'NONE',  ( -41.25198945386251381, 23.25239630053170714, 1.523999999999992916 ) ) ;
#2940=VERTEX_POINT ( 'NONE', #15201 ) ;
#2942=CARTESIAN_POINT ( 'NONE',  ( -28.95189557067410746, 64.41341631820462510, 1.523999999999993360 ) ) ;
#2944=DIRECTION ( 'NONE',  ( -5.188838149069471174E-16, 1.699382548006136313E-16, 1.000000000000000000 ) ) ;
#2949=CARTESIAN_POINT ( 'NONE',  ( -52.95179419874195048, 11.24610246600658137, -4.133922171301945170 ) ) ;
#2955=AXIS2_PLACEMENT_3D ( 'NONE', #13412, #41977, #3849 ) ;
#2956=EDGE_LOOP ( 'NONE', ( #36714, #1765, #34518, #33198 ) ) ;
#2960=VECTOR ( 'NONE', #14167, 1000.000000000000000 ) ;
#2962=EDGE_CURVE ( 'NONE', #30889, #12049, #40264, .T. ) ;
#2964=ORIENTED_EDGE ( 'NONE', *, *, #11343, .T. ) ;
#2974=CARTESIAN_POINT ( 'NONE',  ( -52.53679969070437750, 11.65360597696575873, 4.035185998988639611 ) ) ;
#2977=CARTESIAN_POINT ( 'NONE',  ( -47.00787117332040310, 24.49876931072293829, 2.333946431867817584 ) ) ;
#2978=CARTESIAN_POINT ( 'NONE',  ( -58.82785807807199063, -0.2608716074412517072, 0.04555283349572796653 ) ) ;
#2982=ORIENTED_EDGE ( 'NONE', *, *, #14629, .T. ) ;
#2983=CARTESIAN_POINT ( 'NONE',  ( -24.32950799593924884, 77.42192949967211746, -1.524000000000005572 ) ) ;
#2990=AXIS2_PLACEMENT_3D ( 'NONE', #3329, #12692, #29300 ) ;
#2994=CARTESIAN_POINT ( 'NONE',  ( -4.345705637489785111, 70.43763872253877878, -1.269999999999994023 ) ) ;
#3002=ORIENTED_EDGE ( 'NONE', *, *, #23149, .F. ) ;
#3004=CIRCLE ( 'NONE', #21326, 8.794749999999993406 ) ;
#3009=VERTEX_POINT ( 'NONE', #5921 ) ;
#3011=CARTESIAN_POINT ( 'NONE',  ( -41.31025181302593552, 22.81788724727718076, 1.523999999999983146 ) ) ;
#3012=EDGE_CURVE ( 'NONE', #34369, #4125, #30049, .T. ) ;
#3016=DIRECTION ( 'NONE',  ( -0.1906721105965087926, 0.9816537812491085147, 0.000000000000000000 ) ) ;
#3019=AXIS2_PLACEMENT_3D ( 'NONE', #16498, #25672, #28871 ) ;
#3021=FACE_OUTER_BOUND ( 'NONE', #32541, .T. ) ;
#3032=LINE ( 'NONE', #15987, #30102 ) ;
#3043=CARTESIAN_POINT ( 'NONE',  ( -23.34387769576312621, 77.71194901948682343, 1.269999999999993134 ) ) ;
#3047=EDGE_CURVE ( 'NONE', #16319, #16174, #16899, .T. ) ;
#3048=DIRECTION ( 'NONE',  ( -0.9454731675810336133, 0.3256999990547843615, -5.459396135145337199E-16 ) ) ;
#3053=DIRECTION ( 'NONE',  ( -0.6594218222380214822, -0.7517731442105972661, -2.144082946226365319E-16 ) ) ;
#3056=CARTESIAN_POINT ( 'NONE',  ( -43.04734275525184728, 21.71211564561841101, -2.244749861974538074 ) ) ;
#3061=CARTESIAN_POINT ( 'NONE',  ( -56.38145225766449187, 4.490824468634439626, -2.575949247650338503 ) ) ;
#3063=CARTESIAN_POINT ( 'NONE',  ( -48.97544177847666447, 17.83334834807594049, -5.075951225172628867 ) ) ;
#3067=CARTESIAN_POINT ( 'NONE',  ( -17.14500000000466784, 71.11999999999886768, 1.523999999999998689 ) ) ;
#3070=CARTESIAN_POINT ( 'NONE',  ( -57.57967628038989005, 1.451576601202181349, -1.494865757154152153 ) ) ;
#3071=ORIENTED_EDGE ( 'NONE', *, *, #31245, .T. ) ;
#3084=DIRECTION ( 'NONE',  ( -0.3582377630123906309, 0.9336303900108855469, 0.000000000000000000 ) ) ;
#3085=CARTESIAN_POINT ( 'NONE',  ( -49.14072577824710208, 13.89916973120787524, -0.4067138869237436061 ) ) ;
#3086=EDGE_LOOP ( 'NONE', ( #8479, #22620, #4696, #3580 ) ) ;
#3088=CARTESIAN_POINT ( 'NONE',  ( -47.66286930719412851, 20.62480072838431155, 5.054501799269492501 ) ) ;
#3089=CARTESIAN_POINT ( 'NONE',  ( -53.96359711957523331, 9.317927474182681635, 3.738358014028002607 ) ) ;
#3092=DIRECTION ( 'NONE',  ( 5.188838149069472160E-16, -1.699382548006136559E-16, -1.000000000000000000 ) ) ;
#3093=CARTESIAN_POINT ( 'NONE',  ( -55.38777061991515183, 7.924152594517688719, 2.969223861581042012 ) ) ;
#3096=CARTESIAN_POINT ( 'NONE',  ( -54.80060171144386771, 10.20856468236482684, -2.175828276708582365 ) ) ;
#3098=ORIENTED_EDGE ( 'NONE', *, *, #15474, .T. ) ;
#3103=CARTESIAN_POINT ( 'NONE',  ( -17.14500000000466784, 71.11999999999886768, 1.269999999999998241 ) ) ;
#3106=DIRECTION ( 'NONE',  ( 5.188838149069472160E-16, -1.699382548006136559E-16, -1.000000000000000000 ) ) ;
#3109=DIRECTION ( 'NONE',  ( 0.01731298258488772612, -0.9998501190848633202, 1.788962107505314604E-16 ) ) ;
#3111=CIRCLE ( 'NONE', #24828, 0.2540000000000052771 ) ;
#3113=ORIENTED_EDGE ( 'NONE', *, *, #18091, .F. ) ;
#3114=CARTESIAN_POINT ( 'NONE',  ( -58.36160036302118215, -0.2744091231881636284, -0.1136734763339792287 ) ) ;
#3124=CARTESIAN_POINT ( 'NONE',  ( -13.99440778436217414, 79.95103047660883533, -1.270000000000000462 ) ) ;
#3125=CARTESIAN_POINT ( 'NONE',  ( -45.76673701974917208, 25.51931200435043934, -1.524000000000008237 ) ) ;
#3126=ORIENTED_EDGE ( 'NONE', *, *, #14081, .F. ) ;
#3130=DIRECTION ( 'NONE',  ( 5.188838149069472160E-16, -1.699382548006136559E-16, -1.000000000000000000 ) ) ;
#3144=CYLINDRICAL_SURFACE ( 'NONE', #17880, 0.5080000000000000071 ) ;
#3146=ORIENTED_EDGE ( 'NONE', *, *, #3265, .T. ) ;
#3150=DIRECTION ( 'NONE',  ( -0.8745520943968243532, 0.4849315768086547296, -5.361993529360573944E-16 ) ) ;
#3160=AXIS2_PLACEMENT_3D ( 'NONE', #38302, #6142, #38510 ) ;
#3162=AXIS2_PLACEMENT_3D ( 'NONE', #9047, #22423, #3084 ) ;
#3164=VECTOR ( 'NONE', #24276, 1000.000000000000000 ) ;
#3166=CARTESIAN_POINT ( 'NONE',  ( -25.81615557310160369, 74.46796499802707103, 1.269999999999993578 ) ) ;
#3175=CARTESIAN_POINT ( 'NONE',  ( -46.65771312250404179, 26.07706844218929731, 1.303905986063749411 ) ) ;
#3178=ORIENTED_EDGE ( 'NONE', *, *, #27512, .T. ) ;
#3179=CARTESIAN_POINT ( 'NONE',  ( -43.93316818929329770, 24.49458088220322338, 1.523999999999992916 ) ) ;
#3181=ADVANCED_FACE ( 'NONE', ( #33108 ), #41626, .T. ) ;
#3186=DIRECTION ( 'NONE',  ( -0.8745520943968148053, 0.4849315768086717160, -5.691349986800521255E-16 ) ) ;
#3194=CARTESIAN_POINT ( 'NONE',  ( -23.62918761621517305, 82.45577215708875940, 1.523999999999993360 ) ) ;
#3197=ADVANCED_FACE ( 'NONE', ( #29690 ), #34806, .T. ) ;
#3204=LINE ( 'NONE', #32803, #23997 ) ;
#3213=ORIENTED_EDGE ( 'NONE', *, *, #38388, .F. ) ;
#3214=CARTESIAN_POINT ( 'NONE',  ( -47.69647088358534859, 18.57426963660985209, 3.960430087866664284 ) ) ;
#3222=DIRECTION ( 'NONE',  ( -0.8745520943968241312, 0.4849315768086548406, -5.691349986800536046E-16 ) ) ;
#3227=CIRCLE ( 'NONE', #8661, 0.2539999999999992819 ) ;
#3229=DIRECTION ( 'NONE',  ( 0.6559537821943236535, -0.7548010569845287066, 4.686333752532406881E-16 ) ) ;
#3232=ADVANCED_FACE ( 'NONE', ( #14324 ), #35503, .T. ) ;
#3233=FACE_OUTER_BOUND ( 'NONE', #39932, .T. ) ;
#3246=DIRECTION ( 'NONE',  ( -0.8745520943968243532, 0.4849315768086547296, -6.829619984160642269E-16 ) ) ;
#3250=DIRECTION ( 'NONE',  ( -0.8745520943968235761, 0.4849315768086558398, -4.268512490100410909E-16 ) ) ;
#3257=DIRECTION ( 'NONE',  ( -0.9998501190848629872, -0.01731298258490740830, -8.537024980200807027E-16 ) ) ;
#3258=ORIENTED_EDGE ( 'NONE', *, *, #6887, .T. ) ;
#3264=CARTESIAN_POINT ( 'NONE',  ( -58.69116746987842959, -0.3144157293073903681, -0.2986533189990187576 ) ) ;
#3265=EDGE_CURVE ( 'NONE', #25412, #27671, #1563, .T. ) ;
#3266=VERTEX_POINT ( 'NONE', #26912 ) ;
#3267=CARTESIAN_POINT ( 'NONE',  ( -58.40429423216704663, -0.3346038877942508760, -0.4235997928873705964 ) ) ;
#3271=DIRECTION ( 'NONE',  ( -5.188838149069472160E-16, 1.699382548006136559E-16, 1.000000000000000000 ) ) ;
#3275=AXIS2_PLACEMENT_3D ( 'NONE', #6670, #19223, #39468 ) ;
#3276=ORIENTED_EDGE ( 'NONE', *, *, #3870, .T. ) ;
#3279=EDGE_LOOP ( 'NONE', ( #29860, #37245, #7086, #6080 ) ) ;
#3287=CARTESIAN_POINT ( 'NONE',  ( -46.58649794690494872, 25.68081001442251221, 1.571531081468684032 ) ) ;
#3290=DIRECTION ( 'NONE',  ( -0.2883665106726627791, -0.9575201071113198514, -8.211810011157224448E-16 ) ) ;
#3291=CARTESIAN_POINT ( 'NONE',  ( -47.74911022259793469, 17.86741523025699152, -3.129844374475875934 ) ) ;
#3293=PLANE ( 'NONE',  #20297 ) ;
#3294=CARTESIAN_POINT ( 'NONE',  ( -48.00704091872448487, 20.04541143072568232, 5.176114466449816653 ) ) ;
#3295=CARTESIAN_POINT ( 'NONE',  ( -17.97610982144389524, 83.97333317030323485, 1.269999999999995799 ) ) ;
#3298=DIRECTION ( 'NONE',  ( 0.8745520943968235761, -0.4849315768086558398, 4.268512490100410909E-16 ) ) ;
#3299=CARTESIAN_POINT ( 'NONE',  ( -6.194847070882102180, 64.72978607931611350, 1.270000000000005125 ) ) ;
#3300=CARTESIAN_POINT ( 'NONE',  ( -55.64884842185075087, 8.819639511685364752, 1.021878145082198763 ) ) ;
#3301=CARTESIAN_POINT ( 'NONE',  ( -57.09878488423309051, 3.216020309495956742, 2.217633722229532367 ) ) ;
#3303=ORIENTED_EDGE ( 'NONE', *, *, #19897, .T. ) ;
#3304=CARTESIAN_POINT ( 'NONE',  ( -50.72152632752359125, 17.59631655692102470, -3.767527310968358911 ) ) ;
#3306=ORIENTED_EDGE ( 'NONE', *, *, #35725, .T. ) ;
#3310=DIRECTION ( 'NONE',  ( -0.9816537812491089587, -0.1906721105965065444, -4.769617732184475162E-16 ) ) ;
#3317=CARTESIAN_POINT ( 'NONE',  ( -18.19824605342069290, 84.09650579081264254, 1.269999999999996465 ) ) ;
#3318=ORIENTED_EDGE ( 'NONE', *, *, #27124, .T. ) ;
#3320=ORIENTED_EDGE ( 'NONE', *, *, #24903, .T. ) ;
#3329=CARTESIAN_POINT ( 'NONE',  ( -19.33375693323417366, 80.42273151551299293, 1.523999999999995802 ) ) ;
#3332=ORIENTED_EDGE ( 'NONE', *, *, #19873, .T. ) ;
#3334=ADVANCED_FACE ( 'NONE', ( #40347 ), #8283, .T. ) ;
#3338=CARTESIAN_POINT ( 'NONE',  ( -48.04822308881582416, 19.89521662531995005, -5.294633059834412236 ) ) ;
#3343=TOROIDAL_SURFACE ( 'NONE', #27792, 0.3810000000000002829, 0.2540000000000000036 ) ;
#3344=DIRECTION ( 'NONE',  ( -5.188838149069472160E-16, 1.699382548006136559E-16, 1.000000000000000000 ) ) ;
#3349=CARTESIAN_POINT ( 'NONE',  ( -47.84356795211461844, 19.38525671449500010, -5.197506975155170572 ) ) ;
#3352=ORIENTED_EDGE ( 'NONE', *, *, #19649, .F. ) ;
#3354=DIRECTION ( 'NONE',  ( 0.9336303900108815501, 0.3582377630124009560, 4.235673982319039874E-16 ) ) ;
#3359=ORIENTED_EDGE ( 'NONE', *, *, #10292, .F. ) ;
#3368=DIRECTION ( 'NONE',  ( -5.188838149069472160E-16, 1.699382548006136559E-16, 1.000000000000000000 ) ) ;
#3369=VECTOR ( 'NONE', #13402, 1000.000000000000000 ) ;
#3374=VERTEX_POINT ( 'NONE', #37137 ) ;
#3383=DIRECTION ( 'NONE',  ( -5.188838149069471174E-16, 1.699382548006136313E-16, 1.000000000000000000 ) ) ;
#3385=TOROIDAL_SURFACE ( 'NONE', #26527, 0.7620000000000000107, 0.2540000000000000036 ) ;
#3387=AXIS2_PLACEMENT_3D ( 'NONE', #32321, #6550, #16756 ) ;
#3390=CARTESIAN_POINT ( 'NONE',  ( -51.34742739204327222, 13.85210956937153348, 4.439032809404257485 ) ) ;
#3393=CARTESIAN_POINT ( 'NONE',  ( -51.09990735641632398, 14.52648110433587370, 4.713018929684107405 ) ) ;
#3397=EDGE_LOOP ( 'NONE', ( #41828, #17194, #23312, #35964 ) ) ;
#3402=CARTESIAN_POINT ( 'NONE',  ( -47.01067208220106863, 24.90190543975541360, -1.870441909736414221 ) ) ;
#3405=LINE ( 'NONE', #22962, #37379 ) ;
#3411=CARTESIAN_POINT ( 'NONE',  ( -28.36525985791271154, 77.02308833105713859, 1.269999999999991580 ) ) ;
#3423=ORIENTED_EDGE ( 'NONE', *, *, #6687, .T. ) ;
#3425=AXIS2_PLACEMENT_3D ( 'NONE', #9397, #250, #6420 ) ;
#3427=CARTESIAN_POINT ( 'NONE',  ( -42.09164859969784089, 21.98995510696678934, 0.2271816505417205145 ) ) ;
#3433=CARTESIAN_POINT ( 'NONE',  ( -47.85244527695891037, 19.39403540832952544, -5.219971639306605127 ) ) ;
#3438=ORIENTED_EDGE ( 'NONE', *, *, #14708, .F. ) ;
#3441=CARTESIAN_POINT ( 'NONE',  ( -28.09515292912719175, 77.51021392068167870, -1.270000000000007345 ) ) ;
#3442=TOROIDAL_SURFACE ( 'NONE', #4817, 8.794749999999996959, 0.2540000000000000036 ) ;
#3443=CYLINDRICAL_SURFACE ( 'NONE', #2180, 0.5080000000000000071 ) ;
#3448=AXIS2_PLACEMENT_3D ( 'NONE', #4549, #17507, #1347 ) ;
#3453=EDGE_CURVE ( 'NONE', #37511, #3974, #10137, .T. ) ;
#3465=AXIS2_PLACEMENT_3D ( 'NONE', #40175, #13957, #10348 ) ;
#3471=ORIENTED_EDGE ( 'NONE', *, *, #4804, .T. ) ;
#3478=B_SPLINE_CURVE_WITH_KNOTS ( 'NONE', 3,
 ( #21225, #37857, #21431, #8253, #18241, #11032, #27224, #30412, #34256, #5085, #14840, #27845, #24861, #4873, #11654, #28052 ),
 .UNSPECIFIED., .F., .F.,
 ( 4, 2, 2, 2, 2, 2, 2, 4 ),
 ( 0.000000000000000000, 0.005261262525262890531, 0.007891893787894345771, 0.01052252505052580014, 0.01578378757578872624, 0.01709910320710445950, 0.01841441883842019275, 0.02104505010105165580 ),
 .UNSPECIFIED. ) ;
#3480=CARTESIAN_POINT ( 'NONE',  ( -58.65524206761604376, -0.3162046652864728413, -0.3252180803564949096 ) ) ;
#3482=LINE ( 'NONE', #16442, #39497 ) ;
#3491=CARTESIAN_POINT ( 'NONE',  ( -58.50860430493789721, 0.7049166599848305514, -0.9756837515128595761 ) ) ;
#3492=ORIENTED_EDGE ( 'NONE', *, *, #14908, .F. ) ;
#3495=ORIENTED_EDGE ( 'NONE', *, *, #4575, .T. ) ;
#3500=ADVANCED_FACE ( 'NONE', ( #32420 ), #32214, .T. ) ;
#3507=DIRECTION ( 'NONE',  ( -0.7770581983690836303, 0.6294287539884032556, -5.101669463485833779E-16 ) ) ;
#3508=CARTESIAN_POINT ( 'NONE',  ( -46.62078961162516322, 17.34433182989875277, -0.7188397291161608971 ) ) ;
#3513=DIRECTION ( 'NONE',  ( 0.000000000000000000, 0.000000000000000000, -1.000000000000000000 ) ) ;
#3517=CARTESIAN_POINT ( 'NONE',  ( -23.14542444889682216, 82.37908244650444090, 1.269999999999993578 ) ) ;
#3518=CARTESIAN_POINT ( 'NONE',  ( -57.71825614945207406, 2.868614883688350048, 0.7691332274306142969 ) ) ;
#3519=CARTESIAN_POINT ( 'NONE',  ( -57.71946847630993460, 1.146847591362354368, 1.351507486235933975 ) ) ;
#3522=CARTESIAN_POINT ( 'NONE',  ( -53.89938688035451975, 11.68864614896874343, -3.017114338529875095 ) ) ;
#3529=VECTOR ( 'NONE', #29481, 1000.000000000000000 ) ;
#3531=LINE ( 'NONE', #32057, #31548 ) ;
#3533=EDGE_CURVE ( 'NONE', #12640, #35416, #15741, .T. ) ;
#3540=VERTEX_POINT ( 'NONE', #32629 ) ;
#3542=CARTESIAN_POINT ( 'NONE',  ( -58.36955422849574404, -0.2910357702952456882, -0.02058977239408909393 ) ) ;
#3546=VECTOR ( 'NONE', #22113, 1000.000000000000114 ) ;
#3550=CARTESIAN_POINT ( 'NONE',  ( -23.91048590848665967, 81.84235438443283783, 1.269999999999993801 ) ) ;
#3551=AXIS2_PLACEMENT_3D ( 'NONE', #28708, #40875, #5108 ) ;
#3558=CARTESIAN_POINT ( 'NONE',  ( -48.65005484009959957, 18.46594748123760965, -5.297328305960443018 ) ) ;
#3562=LINE ( 'NONE', #156, #2846 ) ;
#3568=DIRECTION ( 'NONE',  ( 0.6294287539883864913, 0.7770581983690970640, 0.000000000000000000 ) ) ;
#3577=DIRECTION ( 'NONE',  ( -0.8745520943968250194, 0.4849315768086532863, -5.361993529360574930E-16 ) ) ;
#3580=ORIENTED_EDGE ( 'NONE', *, *, #24523, .F. ) ;
#3583=DIRECTION ( 'NONE',  ( -0.8745520943968383420, 0.4849315768086291945, -4.268512490100416826E-16 ) ) ;
#3589=CARTESIAN_POINT ( 'NONE',  ( -22.85582906289733529, 78.03019435252696212, 1.269999999999994245 ) ) ;
#3597=CARTESIAN_POINT ( 'NONE',  ( -30.20416046766210272, 71.17241488000101413, -1.524000000000007571 ) ) ;
#3598=AXIS2_PLACEMENT_3D ( 'NONE', #41612, #15389, #25413 ) ;
#3608=CARTESIAN_POINT ( 'NONE',  ( -49.36011206067185242, 17.22521247008247158, 4.983413103225731611 ) ) ;
#3609=CARTESIAN_POINT ( 'NONE',  ( -49.59145623469802899, 21.58002366008788542, 1.574391596335662058 ) ) ;
#3611=CARTESIAN_POINT ( 'NONE',  ( -49.13940628111213016, 17.59503125033257120, 5.062072503518671773 ) ) ;
#3615=ORIENTED_EDGE ( 'NONE', *, *, #3047, .F. ) ;
#3616=ORIENTED_EDGE ( 'NONE', *, *, #14158, .F. ) ;
#3621=CARTESIAN_POINT ( 'NONE',  ( -46.68114719912644262, 26.04180998113828238, -1.171086909392329956 ) ) ;
#3629=DIRECTION ( 'NONE',  ( -5.188838149069472160E-16, 1.699382548006136559E-16, 1.000000000000000000 ) ) ;
#3643=CARTESIAN_POINT ( 'NONE',  ( -45.58494389689084869, 18.10922195552001313, -6.304117962515870643E-15 ) ) ;
#3653=DIRECTION ( 'NONE',  ( -5.188838149069471174E-16, 1.699382548006136313E-16, 1.000000000000000000 ) ) ;
#3655=CARTESIAN_POINT ( 'NONE',  ( -23.75665686005077504, 76.91945007112674659, 1.523999999999994248 ) ) ;
#3659=PLANE ( 'NONE',  #32946 ) ;
#3662=CARTESIAN_POINT ( 'NONE',  ( -28.65049350906917880, 77.81814547195517662, -1.270000000000007789 ) ) ;
#3677=EDGE_CURVE ( 'NONE', #29032, #25412, #35408, .T. ) ;
#3681=DIRECTION ( 'NONE',  ( -0.3582377630123915746, 0.9336303900108851028, -3.445432962228667069E-16 ) ) ;
#3683=CARTESIAN_POINT ( 'NONE',  ( -11.34554992887676406, 77.73165686004495001, 1.270000000000000462 ) ) ;
#3686=CIRCLE ( 'NONE', #1617, 0.2540000000000015024 ) ;
#3691=CARTESIAN_POINT ( 'NONE',  ( -58.82051709867915434, -0.2694835746722941683, -0.08083543577478463638 ) ) ;
#3693=CARTESIAN_POINT ( 'NONE',  ( -27.82636559844506152, 59.51700088791086074, -1.270000000000004237 ) ) ;
#3696=TOROIDAL_SURFACE ( 'NONE', #9122, 8.794749999999998735, 0.2540000000000000036 ) ;
#3701=CARTESIAN_POINT ( 'NONE',  ( -57.15088083682995546, 2.378576142695001838, -1.865916551128065981 ) ) ;
#3702=CIRCLE ( 'NONE', #14550, 8.794749999999993406 ) ;
#3709=AXIS2_PLACEMENT_3D ( 'NONE', #28921, #41524, #42150 ) ;
#3711=ADVANCED_FACE ( 'NONE', ( #57 ), #10980, .T. ) ;
#3712=CARTESIAN_POINT ( 'NONE',  ( -58.34169784303173856, -0.2326338189565652081, 0.2089577666115795540 ) ) ;
#3720=CARTESIAN_POINT ( 'NONE',  ( -54.90394170586843359, 6.776736168479208011, -2.460356751892069038 ) ) ;
#3723=CARTESIAN_POINT ( 'NONE',  ( -47.35944255389389923, 21.37623662739411401, 4.722871667523157235 ) ) ;
#3724=DIRECTION ( 'NONE',  ( 0.8745520943968235761, -0.4849315768086558398, 0.000000000000000000 ) ) ;
#3725=CARTESIAN_POINT ( 'NONE',  ( -29.27789202445837091, 65.71096991539570809, -1.269999999999910090 ) ) ;
#3726=CARTESIAN_POINT ( 'NONE',  ( -58.63679809531443965, -0.7731007215655836262, -1.422417852365874970E-12 ) ) ;
#3728=DIRECTION ( 'NONE',  ( -0.7548010569845451379, -0.6559537821943047797, 0.000000000000000000 ) ) ;
#3729=CARTESIAN_POINT ( 'NONE',  ( -57.67985703563598321, 3.143487229238031588, 0.2637475255842167132 ) ) ;
#3730=ADVANCED_FACE ( 'NONE', ( #16638 ), #18445, .T. ) ;
#3731=CARTESIAN_POINT ( 'NONE',  ( -57.22363667057550884, 2.289652018204080264, 1.875138655370640173 ) ) ;
#3734=CARTESIAN_POINT ( 'NONE',  ( -53.35592009511452716, 14.94916803242400682, -1.377413129700665539 ) ) ;
#3737=FACE_OUTER_BOUND ( 'NONE', #19043, .T. ) ;
#3748=EDGE_CURVE ( 'NONE', #38326, #37552, #39233, .T. ) ;
#3754=CARTESIAN_POINT ( 'NONE',  ( -58.25346979615795817, -0.04388205940947602357, -0.4484691845572629787 ) ) ;
#3768=EDGE_CURVE ( 'NONE', #5200, #39243, #23208, .T. ) ;
#3769=CARTESIAN_POINT ( 'NONE',  ( -46.31144060707497090, 24.05480373873685451, -2.308638262703932575 ) ) ;
#3772=DIRECTION ( 'NONE',  ( -5.188838149069471174E-16, 1.699382548006136313E-16, 1.000000000000000000 ) ) ;
#3773=ADVANCED_FACE ( 'NONE', ( #40509 ), #21173, .T. ) ;
#3781=CARTESIAN_POINT ( 'NONE',  ( -17.58995245299100674, 75.15621874538170744, -1.270000000000001572 ) ) ;
#3783=AXIS2_PLACEMENT_3D ( 'NONE', #18313, #31315, #41556 ) ;
#3784=ORIENTED_EDGE ( 'NONE', *, *, #12552, .T. ) ;
#3790=DIRECTION ( 'NONE',  ( 0.3256999990547897461, 0.9454731675810318370, 0.000000000000000000 ) ) ;
#3792=ORIENTED_EDGE ( 'NONE', *, *, #38602, .T. ) ;
#3804=ORIENTED_EDGE ( 'NONE', *, *, #34186, .F. ) ;
#3810=CARTESIAN_POINT ( 'NONE',  ( -5.861642722916909243, 64.54502714855203749, 1.270000000000005347 ) ) ;
#3812=AXIS2_PLACEMENT_3D ( 'NONE', #5101, #8489, #1693 ) ;
#3813=ORIENTED_EDGE ( 'NONE', *, *, #24095, .T. ) ;
#3818=ADVANCED_FACE ( 'NONE', ( #4314 ), #10467, .T. ) ;
#3821=EDGE_CURVE ( 'NONE', #31300, #40156, #33694, .T. ) ;
#3824=CARTESIAN_POINT ( 'NONE',  ( -50.84765044967730319, 14.73090700864087488, 4.586134481135779595 ) ) ;
#3825=CARTESIAN_POINT ( 'NONE',  ( -48.35471193741586404, 22.70554656608007704, 1.835820227619837208 ) ) ;
#3827=CARTESIAN_POINT ( 'NONE',  ( -55.60508136934060275, 7.116827924314645060, 3.170888472016278214 ) ) ;
#3828=CARTESIAN_POINT ( 'NONE',  ( -58.68986611463690650, -0.3143780598132880910, 0.3000052052140327885 ) ) ;
#3830=CARTESIAN_POINT ( 'NONE',  ( -58.15296624161964445, 0.1186235457594081444, -0.2061892363120086946 ) ) ;
#3833=CARTESIAN_POINT ( 'NONE',  ( -46.89970385779243855, 22.02655025333852379, 4.237790764466920379 ) ) ;
#3838=CARTESIAN_POINT ( 'NONE',  ( -15.42835734045148399, 79.74558783746839197, -1.524000000000001576 ) ) ;
#3839=DIRECTION ( 'NONE',  ( -0.8745520943968240202, 0.4849315768086553402, -6.829619984160650158E-16 ) ) ;
#3844=AXIS2_PLACEMENT_3D ( 'NONE', #20970, #5658, #5232 ) ;
#3849=DIRECTION ( 'NONE',  ( -0.8745520943968937422, 0.4849315768085294409, -5.691349986800560698E-16 ) ) ;
#3855=VERTEX_POINT ( 'NONE', #30064 ) ;
#3856=CARTESIAN_POINT ( 'NONE',  ( -41.36952270831616119, 22.75442529069328401, 0.6632742133606186474 ) ) ;
#3869=FACE_OUTER_BOUND ( 'NONE', #12428, .T. ) ;
#3870=EDGE_CURVE ( 'NONE', #6455, #3855, #29194, .T. ) ;
#3872=EDGE_CURVE ( 'NONE', #1116, #38897, #4101, .T. ) ;
#3874=DIRECTION ( 'NONE',  ( 5.188838149069472160E-16, -1.699382548006136559E-16, -1.000000000000000000 ) ) ;
#3890=FACE_OUTER_BOUND ( 'NONE', #12202, .T. ) ;
#3907=DIRECTION ( 'NONE',  ( -0.3256999990547876367, -0.9454731675810326141, -8.328397965208553695E-18 ) ) ;
#3912=CARTESIAN_POINT ( 'NONE',  ( -7.961576494521615643, 72.55615504727386167, 1.524000000000003130 ) ) ;
#3916=ORIENTED_EDGE ( 'NONE', *, *, #34254, .T. ) ;
#3919=ORIENTED_EDGE ( 'NONE', *, *, #34423, .F. ) ;
#3922=VECTOR ( 'NONE', #24190, 1000.000000000000000 ) ;
#3924=EDGE_CURVE ( 'NONE', #38171, #39389, #41472, .T. ) ;
#3932=CARTESIAN_POINT ( 'NONE',  ( -54.85284047870325708, 7.073525668766899699, -2.945785012852154772 ) ) ;
#3935=CYLINDRICAL_SURFACE ( 'NONE', #11146, 0.2539999999999992819 ) ;
#3937=CARTESIAN_POINT ( 'NONE',  ( -28.99046981646804966, 65.28995187596837013, -1.524000000000005572 ) ) ;
#3938=DIRECTION ( 'NONE',  ( -0.8745520943968240202, 0.4849315768086551737, -5.361993529360572958E-16 ) ) ;
#3941=CARTESIAN_POINT ( 'NONE',  ( -58.77954282417582732, 0.05649391281087323691, 0.1080441935232383244 ) ) ;
#3942=CARTESIAN_POINT ( 'NONE',  ( -58.20820809768403592, 1.420579653404085985, 1.355822160094593443 ) ) ;
#3944=ORIENTED_EDGE ( 'NONE', *, *, #10274, .F. ) ;
#3945=CARTESIAN_POINT ( 'NONE',  ( -57.78461401849437351, 2.885363594410703225, -1.068429527248437518E-14 ) ) ;
#3947=ORIENTED_EDGE ( 'NONE', *, *, #19933, .T. ) ;
#3954=AXIS2_PLACEMENT_3D ( 'NONE', #6987, #22924, #39574 ) ;
#3961=EDGE_LOOP ( 'NONE', ( #36008, #12328, #25567, #20981 ) ) ;
#3964=CARTESIAN_POINT ( 'NONE',  ( -58.07329405781845111, 0.3456141243580676536, -0.7578522352846541743 ) ) ;
#3974=VERTEX_POINT ( 'NONE', #20670 ) ;
#3977=FACE_OUTER_BOUND ( 'NONE', #33584, .T. ) ;
#3979=ADVANCED_FACE ( 'NONE', ( #14488 ), #20877, .F. ) ;
#3980=CARTESIAN_POINT ( 'NONE',  ( -50.82551848962686591, 16.13924203555649228, -4.804203053272171786 ) ) ;
#3988=EDGE_CURVE ( 'NONE', #31840, #37219, #33988, .T. ) ;
#3990=CARTESIAN_POINT ( 'NONE',  ( -41.09670346151854403, 23.04688172093030829, -1.270085369932534958 ) ) ;
#3995=ADVANCED_FACE ( 'NONE', ( #27501 ), #30477, .F. ) ;
#3997=CARTESIAN_POINT ( 'NONE',  ( -17.14500000000466784, 71.11999999999886768, -1.524000000000000909 ) ) ;
#4005=ADVANCED_FACE ( 'NONE', ( #3890 ), #11096, .T. ) ;
#4013=CARTESIAN_POINT ( 'NONE',  ( -57.94306413390934551, 1.184802614100144424, -1.419326152557812248 ) ) ;
#4014=DIRECTION ( 'NONE',  ( 5.188838149069472160E-16, -1.699382548006136559E-16, -1.000000000000000000 ) ) ;
#4018=ADVANCED_FACE ( 'NONE', ( #1945 ), #11720, .T. ) ;
#4021=CIRCLE ( 'NONE', #8781, 8.794749999999993406 ) ;
#4023=DIRECTION ( 'NONE',  ( -0.8745520943968225769, 0.4849315768086578382, -5.691349986800571545E-16 ) ) ;
#4027=CARTESIAN_POINT ( 'NONE',  ( -17.97610982144389524, 83.97333317030323485, -1.524000000000003130 ) ) ;
#4033=CARTESIAN_POINT ( 'NONE',  ( -53.63336534079370921, 9.545430312881217461, 3.611512385389820334 ) ) ;
#4034=CARTESIAN_POINT ( 'NONE',  ( -47.30609498763488574, 23.90227454495589399, 2.251708124038033443 ) ) ;
#4036=CARTESIAN_POINT ( 'NONE',  ( -56.22331024217277928, 5.808995339285999648, 2.850545730341239814 ) ) ;
#4037=CARTESIAN_POINT ( 'NONE',  ( -56.69685687618531489, 3.834144682062132770, 2.383935162208182579 ) ) ;
#4039=CARTESIAN_POINT ( 'NONE',  ( -58.33591949829837375, -0.2304704932390572170, -0.1444701089452840037 ) ) ;
#4042=CARTESIAN_POINT ( 'NONE',  ( -46.91604881613255174, 25.30076613767161220, 1.786867259277511666 ) ) ;
#4043=AXIS2_PLACEMENT_3D ( 'NONE', #34153, #21332, #10922 ) ;
#4054=DIRECTION ( 'NONE',  ( -5.188838149069472160E-16, 1.699382548006136559E-16, 1.000000000000000000 ) ) ;
#4061=CARTESIAN_POINT ( 'NONE',  ( -4.085839532347240066, 71.06758511999679229, 1.524000000000005350 ) ) ;
#4066=EDGE_CURVE ( 'NONE', #28056, #38820, #24844, .T. ) ;
#4069=CARTESIAN_POINT ( 'NONE',  ( -44.16391282238571847, 20.57229585060895616, 1.749602973179248844 ) ) ;
#4075=EDGE_CURVE ( 'NONE', #23556, #12215, #10162, .T. ) ;
#4081=AXIS2_PLACEMENT_3D ( 'NONE', #25688, #38693, #9501 ) ;
#4082=VERTEX_POINT ( 'NONE', #31309 ) ;
#4086=CARTESIAN_POINT ( 'NONE',  ( -4.394136353581306054, 70.68697878297604120, -1.269999999999994023 ) ) ;
#4090=DIRECTION ( 'NONE',  ( -0.8745520943968235761, 0.4849315768086558398, -4.268512490100410909E-16 ) ) ;
#4101=LINE ( 'NONE', #26868, #38056 ) ;
#4108=CARTESIAN_POINT ( 'NONE',  ( -36.65473259702431363, 28.27472347546386544, 1.269999999999995577 ) ) ;
#4109=ORIENTED_EDGE ( 'NONE', *, *, #37792, .T. ) ;
#4115=CARTESIAN_POINT ( 'NONE',  ( -58.61869681968132539, -0.2701152165257065252, -0.4082390686273099090 ) ) ;
#4116=VERTEX_POINT ( 'NONE', #31524 ) ;
#4121=CARTESIAN_POINT ( 'NONE',  ( -47.85244527695896011, 19.39403540832957518, 5.219971639306693056 ) ) ;
#4124=DIRECTION ( 'NONE',  ( -0.8745520943968249084, 0.4849315768086534528, -5.361993529360573944E-16 ) ) ;
#4125=VERTEX_POINT ( 'NONE', #41125 ) ;
#4128=VERTEX_POINT ( 'NONE', #11931 ) ;
#4130=AXIS2_PLACEMENT_3D ( 'NONE', #20440, #3874, #33467 ) ;
#4132=CARTESIAN_POINT ( 'NONE',  ( -50.01754050905309867, 16.20622680600125420, 4.878148848498067736 ) ) ;
#4138=DIRECTION ( 'NONE',  ( -0.9876665170007969952, 0.1565721916417935344, -5.390917751951444915E-16 ) ) ;
#4139=CARTESIAN_POINT ( 'NONE',  ( -51.42025106686629243, 13.11195823927271320, -3.453838694686346855 ) ) ;
#4142=CARTESIAN_POINT ( 'NONE',  ( -4.476425760464393555, 71.61790547347303004, -1.269999999999994245 ) ) ;
#4143=CARTESIAN_POINT ( 'NONE',  ( -31.37023363772181028, 53.64958092169537451, -1.270000000000005125 ) ) ;
#4144=CARTESIAN_POINT ( 'NONE',  ( -30.60466991297690242, 55.37784481745784149, -1.524000000000004906 ) ) ;
#4145=VECTOR ( 'NONE', #25826, 1000.000000000000114 ) ;
#4148=CARTESIAN_POINT ( 'NONE',  ( -57.78461401849435930, 2.885363594410716992, 0.1114619696582708486 ) ) ;
#4149=CARTESIAN_POINT ( 'NONE',  ( -58.43690671596436914, -0.4125963578781866037, -1.035377653829272970E-14 ) ) ;
#4152=CARTESIAN_POINT ( 'NONE',  ( -56.22979136716762838, 7.596919248368375399, -0.4408371032393147426 ) ) ;
#4154=ORIENTED_EDGE ( 'NONE', *, *, #39143, .T. ) ;
#4156=AXIS2_PLACEMENT_3D ( 'NONE', #20648, #30879, #4712 ) ;
#4168=ORIENTED_EDGE ( 'NONE', *, *, #36999, .F. ) ;
#4171=CARTESIAN_POINT ( 'NONE',  ( -57.85400989612196554, 0.8207036343174740622, -1.039311302907389933 ) ) ;
#4176=CARTESIAN_POINT ( 'NONE',  ( -44.40534991575952972, 23.82367036525651116, -1.730788704199199834 ) ) ;
#4180=ORIENTED_EDGE ( 'NONE', *, *, #6820, .F. ) ;
#4187=CARTESIAN_POINT ( 'NONE',  ( -48.98489377192316852, 18.65252824715059177, -5.272350768541925525 ) ) ;
#4189=B_SPLINE_SURFACE_WITH_KNOTS ( 'NONE', 3, 3, ( 
 ( #28254, #41259, #38058, #8876, #34867 ),
 ( #5699, #15466, #28469, #3125, #29092 ),
 ( #41899, #19080, #42110, #12699, #6522 ),
 ( #9714, #35499, #36138, #26318, #38902 ),
 ( #16728, #16517, #39325, #19497, #29524 ),
 ( #9502, #2919, #12905, #3769, #38694 ),
 ( #6954, #15881, #22263, #16086, #10131 ),
 ( #38484, #26110, #25689, #25894, #32508 ),
 ( #22680, #29732, #13546, #28887, #364 ),
 ( #13119, #13330, #39115, #22468, #572 ),
 ( #23104, #35714, #6318, #151, #19923 ),
 ( #9302, #32939, #35287, #19291, #6115 ),
 ( #32084, #32296, #9920, #3338, #16306 ),
 ( #29308, #6737, #22890, #32725, #35927 ),
 ( #19708, #3558, #4404, #4187, #33356 ),
 ( #17149, #36971, #29939, #36552, #20754 ),
 ( #778, #10555, #30150, #7371, #39967 ),
 ( #23953, #10968, #40174, #14157, #3980 ),
 ( #26537, #30563, #20127, #7168, #30348 ),
 ( #1403, #16940, #7793, #11176, #33779 ),
 ( #37170, #23317, #39760, #33152, #4811 ),
 ( #4606, #27371, #10759, #26750, #1197 ),
 ( #992, #23524, #13956, #24161, #33570 ),
 ( #7579, #17562, #26954, #14359, #20330 ),
 ( #36354, #23740, #40381, #36761, #7993 ),
 ( #20962, #30762, #33983, #17764, #27161 ),
 ( #1613, #20540, #17361, #39542, #13754 ),
 ( #10347, #14570, #30975, #40790, #34393 ),
 ( #27990, #12229, #12012, #41211, #28203 ),
 ( #5650, #34192, #5017, #14989, #27778 ),
 ( #1815, #17978, #31399, #14778, #11590 ),
 ( #18180, #21160, #40997, #35037, #37374 ),
 ( #40583, #15413, #24573, #15200, #8406 ),
 ( #38007, #25220, #37578, #5432, #11802 ),
 ( #5226, #24792, #21366, #8191, #31182 ),
 ( #37788, #2023, #8615, #21577, #38225 ),
 ( #34604, #18389, #5857, #34816, #28417 ),
 ( #18607, #2452, #2241, #25007, #8828 ),
 ( #21789, #31613, #9040, #41423, #11380 ) ),
 .UNSPECIFIED., .F., .F., .F.,
 ( 4, 1, 1, 1, 1, 1, 1, 1, 1, 1, 1, 2, 1, 1, 1, 1, 1, 1, 1, 1, 1, 1, 1, 1, 1, 1, 1, 1, 1, 1, 1, 1, 1, 1, 1, 4 ),
 ( 4, 1, 4 ),
 ( 0.000000000000000000, 0.01653533301974152367, 0.03307066603948304734, 0.04960599905922460223, 0.06614133207896609468, 0.08267666509870763569, 0.09921199811844919059, 0.1322826641579321894, 0.1653533301974152714, 0.1984239962368983812, 0.2314946622763813522, 0.2645653283158643787, 0.3105299952961229071, 0.3335123287862520880, 0.3564946622763812689, 0.4024593292566397418, 0.4484239962368982702, 0.4943886632171566875, 0.5403533301974150493, 0.5863179971776735222, 0.6322826641579321061, 0.6782473311381906900, 0.7242119981184491628, 0.7701766650987074136, 0.8161413320789658865, 0.8621059990592241373, 0.8735971658042887000, 0.8850883325493537068, 0.8965794992944182695, 0.9080706660394826102, 0.9195618327845473949, 0.9310529995296121797, 0.9425441662746769644, 0.9540353330197415271, 0.9770176665098706525, 1.000000000000000000 ),
 ( 0.000000000000000000, 0.5000000000000000000, 1.000000000000000000 ),
 .UNSPECIFIED. ) ;
#4197=CARTESIAN_POINT ( 'NONE',  ( -46.76714659696671106, 20.35889133747131652, -4.890039387021453798 ) ) ;
#4198=FACE_OUTER_BOUND ( 'NONE', #24679, .T. ) ;
#4200=ORIENTED_EDGE ( 'NONE', *, *, #26140, .T. ) ;
#4202=DIRECTION ( 'NONE',  ( -5.188838149069471174E-16, 1.699382548006136313E-16, 1.000000000000000000 ) ) ;
#4212=VERTEX_POINT ( 'NONE', #19564 ) ;
#4216=CARTESIAN_POINT ( 'NONE',  ( -11.34554992887676228, 77.73165686004496422, -1.269999999999998685 ) ) ;
#4218=ORIENTED_EDGE ( 'NONE', *, *, #33196, .T. ) ;
#4222=CARTESIAN_POINT ( 'NONE',  ( -57.79605042197182030, 0.9991760233560177396, -1.356629168144531494 ) ) ;
#4223=CARTESIAN_POINT ( 'NONE',  ( -24.24369025645184905, 82.02711331519694227, -1.524000000000006239 ) ) ;
#4225=AXIS2_PLACEMENT_3D ( 'NONE', #13379, #38740, #25939 ) ;
#4231=DIRECTION ( 'NONE',  ( -5.188838149069471174E-16, 1.699382548006136313E-16, 1.000000000000000000 ) ) ;
#4235=FACE_OUTER_BOUND ( 'NONE', #12298, .T. ) ;
#4237=AXIS2_PLACEMENT_3D ( 'NONE', #15053, #24862, #37858 ) ;
#4242=DIRECTION ( 'NONE',  ( -0.3256999990547897461, -0.9454731675810318370, 0.000000000000000000 ) ) ;
#4245=CARTESIAN_POINT ( 'NONE',  ( -52.59820521890329559, 11.53769016215144916, 4.012948236587642548 ) ) ;
#4246=CARTESIAN_POINT ( 'NONE',  ( -49.18322560636019602, 21.37428572888716616, 2.217132718382739398 ) ) ;
#4248=CARTESIAN_POINT ( 'NONE',  ( -54.12303657725384198, 9.464413707472848714, 3.807237671326749506 ) ) ;
#4249=CARTESIAN_POINT ( 'NONE',  ( -58.48165732182965115, 0.01964004061440082285, 0.7222573681096682296 ) ) ;
#4252=VERTEX_POINT ( 'NONE', #15745 ) ;
#4253=CARTESIAN_POINT ( 'NONE',  ( -42.33919149967392315, 22.05006338260229271, 1.842566675324087022 ) ) ;
#4254=TOROIDAL_SURFACE ( 'NONE', #9666, 0.7620000000000000107, 0.2540000000000000036 ) ;
#4264=DIRECTION ( 'NONE',  ( -0.01731298258488073172, 0.9998501190848634312, -1.788962107505278366E-16 ) ) ;
#4277=EDGE_CURVE ( 'NONE', #6546, #33508, #41967, .T. ) ;
#4278=CARTESIAN_POINT ( 'NONE',  ( -53.95448410595108157, 8.335714161839828051, 2.220323970834196636 ) ) ;
#4289=AXIS2_PLACEMENT_3D ( 'NONE', #28583, #41, #12185 ) ;
#4290=ORIENTED_EDGE ( 'NONE', *, *, #17204, .T. ) ;
#4291=EDGE_CURVE ( 'NONE', #2129, #6380, #3405, .T. ) ;
#4295=CARTESIAN_POINT ( 'NONE',  ( -6.135835944515187101, 77.40800365160224317, -1.269999999999996243 ) ) ;
#4298=DIRECTION ( 'NONE',  ( -5.188838149069471174E-16, 1.699382548006136313E-16, 1.000000000000000000 ) ) ;
#4314=FACE_OUTER_BOUND ( 'NONE', #38588, .T. ) ;
#4328=CARTESIAN_POINT ( 'NONE',  ( -25.80936006922821591, 73.72935646344811289, -1.524000000000005794 ) ) ;
#4335=CARTESIAN_POINT ( 'NONE',  ( -26.37263903973852663, 72.23735686029533554, 1.269999999999993356 ) ) ;
#4336=EDGE_LOOP ( 'NONE', ( #26135, #10096, #5482, #24627 ) ) ;
#4338=EDGE_CURVE ( 'NONE', #39389, #42027, #14224, .T. ) ;
#4339=AXIS2_PLACEMENT_3D ( 'NONE', #3810, #616, #7210 ) ;
#4341=EDGE_CURVE ( 'NONE', #37188, #3374, #27167, .T. ) ;
#4342=EDGE_LOOP ( 'NONE', ( #33538, #12154, #24889, #37628 ) ) ;
#4354=CARTESIAN_POINT ( 'NONE',  ( -51.32320689156235005, 13.70825103427969438, -4.126761985266684363 ) ) ;
#4356=DIRECTION ( 'NONE',  ( -0.8745520943968241312, 0.4849315768086548406, -5.691349986800536046E-16 ) ) ;
#4358=CARTESIAN_POINT ( 'NONE',  ( -46.84023172327227513, 25.61286091221859351, -1.557636486551099875 ) ) ;
#4360=CARTESIAN_POINT ( 'NONE',  ( -33.20758249455312239, 49.81222039523557044, -1.524000000000005350 ) ) ;
#4363=DIRECTION ( 'NONE',  ( -5.188838149069471174E-16, 1.699382548006136313E-16, 1.000000000000000000 ) ) ;
#4364=CARTESIAN_POINT ( 'NONE',  ( -58.66661043166477896, 0.3408866871785626307, 0.5032371457779101220 ) ) ;
#4365=CARTESIAN_POINT ( 'NONE',  ( -58.73801720703743001, -0.4998429216807459552, 0.2437502737749395465 ) ) ;
#4368=CARTESIAN_POINT ( 'NONE',  ( -57.90853684698413417, 2.514838786807874094, -0.1030880274589022344 ) ) ;
#4370=EDGE_LOOP ( 'NONE', ( #28632, #8684, #18738, #17872 ) ) ;
#4379=CARTESIAN_POINT ( 'NONE',  ( -29.20126717796659577, 63.92883165588695960, 1.269999999999993578 ) ) ;
#4387=CARTESIAN_POINT ( 'NONE',  ( -57.96913128882820132, 0.5713783965472770676, -0.8987469434438276616 ) ) ;
#4390=AXIS2_PLACEMENT_3D ( 'NONE', #10087, #23482, #23696 ) ;
#4391=TOROIDAL_SURFACE ( 'NONE', #26123, 0.7620000000000000107, 0.2540000000000000036 ) ;
#4394=CARTESIAN_POINT ( 'NONE',  ( -47.11704014324645584, 20.18577099567727373, -5.127035723291441194 ) ) ;
#4401=AXIS2_PLACEMENT_3D ( 'NONE', #38679, #39306, #32281 ) ;
#4402=CARTESIAN_POINT ( 'NONE',  ( -30.20416046766209917, 71.17241488000101413, -1.524000000000007571 ) ) ;
#4404=CARTESIAN_POINT ( 'NONE',  ( -48.82738941085167284, 18.57305038084609095, -5.399437279161923620 ) ) ;
#4412=CARTESIAN_POINT ( 'NONE',  ( -42.63057730194584849, 21.82620848986230300, -1.774738817929691237 ) ) ;
#4414=CARTESIAN_POINT ( 'NONE',  ( -57.50808096206083775, 1.366199858870195794, 0.4699486091021412570 ) ) ;
#4417=CARTESIAN_POINT ( 'NONE',  ( -47.62964748377234514, 25.45032632311202647, -0.1281092358103206041 ) ) ;
#4419=DIRECTION ( 'NONE',  ( 5.188838149069471174E-16, -1.699382548006136313E-16, -1.000000000000000000 ) ) ;
#4427=VERTEX_POINT ( 'NONE', #30219 ) ;
#4430=CARTESIAN_POINT ( 'NONE',  ( -17.99070523305417169, 61.93444992276926797, 1.523999999999999799 ) ) ;
#4436=CARTESIAN_POINT ( 'NONE',  ( -58.68789525397659190, -0.3143212917568471987, -0.3020521592213566975 ) ) ;
#4443=CARTESIAN_POINT ( 'NONE',  ( -45.90302585792925782, 20.78970012321182992, 4.334318749026192741 ) ) ;
#4448=CARTESIAN_POINT ( 'NONE',  ( -26.42106975583004314, 72.48669692073261217, -1.270000000000005791 ) ) ;
#4449=CARTESIAN_POINT ( 'NONE',  ( -29.81952093677235993, 58.81079514833387378, -1.270000000000005125 ) ) ;
#4454=CIRCLE ( 'NONE', #26199, 0.5079999999999963434 ) ;
#4457=CARTESIAN_POINT ( 'NONE',  ( -56.65145866349825354, 3.394461374620260763, 2.057387993278029015 ) ) ;
#4458=CARTESIAN_POINT ( 'NONE',  ( -48.87999295267864142, 23.89022491863793718, 0.5351834272454346619 ) ) ;
#4459=CARTESIAN_POINT ( 'NONE',  ( -57.78858274104275949, 1.044662872677112997, 1.355440516197746303 ) ) ;
#4460=CARTESIAN_POINT ( 'NONE',  ( -58.13496148655324447, 0.7694742097100807365, 1.214799913285357302 ) ) ;
#4464=CARTESIAN_POINT ( 'NONE',  ( -46.30033180095409762, 21.65562830348028456, 4.292083522273594909 ) ) ;
#4469=FILL_AREA_STYLE ('',( #7654 ) ) ;
#4473=CARTESIAN_POINT ( 'NONE',  ( -10.00099186598785117, 77.19260062651656540, -1.269999999999998019 ) ) ;
#4474=CYLINDRICAL_SURFACE ( 'NONE', #23055, 0.2540000000000013358 ) ;
#4485=CARTESIAN_POINT ( 'NONE',  ( -51.86985193027736329, 10.34936321858908492, -8.341425858057926505E-15 ) ) ;
#4487=TOROIDAL_SURFACE ( 'NONE', #23506, 0.3809999999999999498, 0.2540000000000000036 ) ;
#4493=DIRECTION ( 'NONE',  ( 0.6825627711659331132, 0.7308269722843310223, 2.299753143848214142E-16 ) ) ;
#4503=DIRECTION ( 'NONE',  ( 0.000000000000000000, 0.000000000000000000, 1.000000000000000000 ) ) ;
#4506=DIRECTION ( 'NONE',  ( 5.188838149069472160E-16, -1.699382548006136559E-16, -1.000000000000000000 ) ) ;
#4507=EDGE_CURVE ( 'NONE', #5717, #25039, #6768, .T. ) ;
#4509=CIRCLE ( 'NONE', #14686, 9.048749999999998295 ) ;
#4510=VERTEX_POINT ( 'NONE', #7026 ) ;
#4518=DIRECTION ( 'NONE',  ( -5.188838149069471174E-16, 1.699382548006136313E-16, 1.000000000000000000 ) ) ;
#4523=CARTESIAN_POINT ( 'NONE',  ( -28.36525985791271154, 77.02308833105713859, -1.270000000000007345 ) ) ;
#4524=ORIENTED_EDGE ( 'NONE', *, *, #41616, .T. ) ;
#4532=FACE_OUTER_BOUND ( 'NONE', #27252, .T. ) ;
#4536=CARTESIAN_POINT ( 'NONE',  ( -45.77009227191969387, 21.09669921233918544, 4.287731683635674251 ) ) ;
#4547=EDGE_LOOP ( 'NONE', ( #7311, #36567, #14602, #25830 ) ) ;
#4549=CARTESIAN_POINT ( 'NONE',  ( -5.684927786827005392, 65.51297084251929448, 1.270000000000005347 ) ) ;
#4550=CARTESIAN_POINT ( 'NONE',  ( -48.44329217233245544, 18.62907245612966634, 5.187175938574861256 ) ) ;
#4557=LINE ( 'NONE', #26699, #35144 ) ;
#4558=CARTESIAN_POINT ( 'NONE',  ( -56.91016477577836952, 2.896953902749091370, -2.060321699029003195 ) ) ;
#4561=CARTESIAN_POINT ( 'NONE',  ( -7.842268484490568348, 73.30875693322846587, 1.524000000000003130 ) ) ;
#4562=CARTESIAN_POINT ( 'NONE',  ( -46.83538438062986842, 25.62937243838004520, -1.546882883115203500 ) ) ;
#4564=CARTESIAN_POINT ( 'NONE',  ( -11.53797084252497385, 82.58007221317646440, -1.524000000000000021 ) ) ;
#4566=DIRECTION ( 'NONE',  ( 5.188838149069472160E-16, -1.699382548006136559E-16, -1.000000000000000000 ) ) ;
#4568=CARTESIAN_POINT ( 'NONE',  ( -58.73915225836899623, 0.1638436772961326948, 0.01855759196810149655 ) ) ;
#4571=CIRCLE ( 'NONE', #1198, 0.5080000000000000071 ) ;
#4572=ORIENTED_EDGE ( 'NONE', *, *, #12305, .F. ) ;
#4573=CARTESIAN_POINT ( 'NONE',  ( -57.37345908981379949, 3.796002467274087078, -0.9053535129859066055 ) ) ;
#4575=EDGE_CURVE ( 'NONE', #30491, #10192, #11249, .T. ) ;
#4576=ORIENTED_EDGE ( 'NONE', *, *, #28731, .T. ) ;
#4577=CARTESIAN_POINT ( 'NONE',  ( -47.20932677516409370, 20.06242161047478234, -5.120036295481038557 ) ) ;
#4585=CARTESIAN_POINT ( 'NONE',  ( -53.23100645945389431, 10.70077955446924456, -4.015069180613662247 ) ) ;
#4587=B_SPLINE_CURVE_WITH_KNOTS ( 'NONE', 3,
 ( #3349, #16315, #26121, #39125, #1413, #17159, #4197, #33994, #13556, #37180, #24169, #7379, #17571, #787, #30159, #16949, #7179, #4412, #20139, #29948, #26545, #10355, #33364, #3990 ),
 .UNSPECIFIED., .F., .F.,
 ( 4, 2, 2, 2, 2, 2, 2, 2, 2, 2, 2, 4 ),
 ( 0.000000000000000000, 0.0005646226568491961037, 0.001129245313698392207, 0.001693867970547588203, 0.002258490627396784415, 0.003387735941095171635, 0.004516981254793559289, 0.005646226568491947810, 0.006775471882190335464, 0.007340094539039522352, 0.007904717195888708373, 0.009033962509587089088 ),
 .UNSPECIFIED. ) ;
#4590=CARTESIAN_POINT ( 'NONE',  ( -57.65211917320155521, 1.256797420531753584, -1.252854774673126670 ) ) ;
#4594=CARTESIAN_POINT ( 'NONE',  ( -47.04837031381860157, 23.61299024743492581, -3.054033755318078303 ) ) ;
#4600=VERTEX_POINT ( 'NONE', #12091 ) ;
#4606=CARTESIAN_POINT ( 'NONE',  ( -53.09398923718962493, 10.65108322687173548, -3.938325876039776574 ) ) ;
#4607=CIRCLE ( 'NONE', #12749, 0.2539999999999967839 ) ;
#4610=DIRECTION ( 'NONE',  ( 0.4849315768086533973, 0.8745520943968251304, 1.030032898892973955E-16 ) ) ;
#4615=DIRECTION ( 'NONE',  ( -0.6825627711659328911, -0.7308269722843309113, -2.299753143848213649E-16 ) ) ;
#4617=CIRCLE ( 'NONE', #31137, 9.048749999999998295 ) ;
#4618=CARTESIAN_POINT ( 'NONE',  ( -57.74348367832291018, 0.8661236967133778553, 0.1780388485286100997 ) ) ;
#4620=EDGE_LOOP ( 'NONE', ( #37823, #14152, #10989, #35771, #65 ) ) ;
#4621=CARTESIAN_POINT ( 'NONE',  ( -46.94769949131580233, 25.36820868695422604, -1.370102228390909005 ) ) ;
#4623=DIRECTION ( 'NONE',  ( 0.8745520943968249084, -0.4849315768086533418, 5.271987356194193006E-16 ) ) ;
#4625=DIRECTION ( 'NONE',  ( 5.188838149069472160E-16, -1.699382548006136559E-16, -1.000000000000000000 ) ) ;
#4631=ORIENTED_EDGE ( 'NONE', *, *, #24776, .F. ) ;
#4634=CARTESIAN_POINT ( 'NONE',  ( -41.81365047723964068, 22.72037957756173654, -1.583806717505435335 ) ) ;
#4636=ORIENTED_EDGE ( 'NONE', *, *, #22473, .F. ) ;
#4640=CARTESIAN_POINT ( 'NONE',  ( -51.96382246822415851, 12.83266463568538285, -4.369925997638347326 ) ) ;
#4646=ORIENTED_EDGE ( 'NONE', *, *, #13888, .F. ) ;
#4656=CIRCLE ( 'NONE', #30386, 0.5080000000000000071 ) ;
#4663=CARTESIAN_POINT ( 'NONE',  ( -55.74547202057183881, 5.289068369273755010, 2.605933947425615571 ) ) ;
#4665=CARTESIAN_POINT ( 'NONE',  ( -57.15088083682995546, 2.378576142695001838, 1.865916551128045553 ) ) ;
#4666=CARTESIAN_POINT ( 'NONE',  ( -56.86472485052055248, 3.482560045344686994, 2.276423594962388997 ) ) ;
#4670=LINE ( 'NONE', #7231, #13818 ) ;
#4676=PRESENTATION_STYLE_ASSIGNMENT (( #33848 ) ) ;
#4682=CARTESIAN_POINT ( 'NONE',  ( -44.26155013454228992, 21.23036713626273553, 2.970720547513075793 ) ) ;
#4688=CARTESIAN_POINT ( 'NONE',  ( -28.92060043785469503, 77.33101988233063651, -1.270000000000007789 ) ) ;
#4696=ORIENTED_EDGE ( 'NONE', *, *, #2710, .F. ) ;
#4697=ADVANCED_FACE ( 'NONE', ( #2315 ), #15275, .T. ) ;
#4698=CARTESIAN_POINT ( 'NONE',  ( -48.84381969468221030, 17.12102923570560975, 3.921819500614938558 ) ) ;
#4705=CYLINDRICAL_SURFACE ( 'NONE', #30196, 0.2540000000000028901 ) ;
#4709=ORIENTED_EDGE ( 'NONE', *, *, #31004, .F. ) ;
#4712=DIRECTION ( 'NONE',  ( -0.8745520943968126959, 0.4849315768086755463, -5.691349986800565628E-16 ) ) ;
#4716=DIRECTION ( 'NONE',  ( -0.8745520943968232430, 0.4849315768086567280, -4.878299988686192207E-16 ) ) ;
#4717=TOROIDAL_SURFACE ( 'NONE', #35987, 0.7620000000000000107, 0.2540000000000000036 ) ;
#4719=CARTESIAN_POINT ( 'NONE',  ( -11.24191166894635430, 82.34025985790688651, 1.523999999999999799 ) ) ;
#4728=CARTESIAN_POINT ( 'NONE',  ( -19.86616884172038766, 72.62886460123898758, -1.524000000000002242 ) ) ;
#4731=DIRECTION ( 'NONE',  ( 0.000000000000000000, 0.000000000000000000, -1.000000000000000000 ) ) ;
#4737=ORIENTED_EDGE ( 'NONE', *, *, #1368, .T. ) ;
#4742=EDGE_CURVE ( 'NONE', #19837, #2010, #28587, .T. ) ;
#4743=EDGE_LOOP ( 'NONE', ( #34011, #26760, #15171, #23379, #37037, #37261 ) ) ;
#4745=CARTESIAN_POINT ( 'NONE',  ( -22.98045850745951313, 78.35500052582088415, 1.269999999999994245 ) ) ;
#4749=AXIS2_PLACEMENT_3D ( 'NONE', #38301, #9325, #2105 ) ;
#4754=DIRECTION ( 'NONE',  ( 0.8745520943968243532, -0.4849315768086547296, 6.829619984160642269E-16 ) ) ;
#4759=EDGE_LOOP ( 'NONE', ( #9421, #36492, #4631, #5176 ) ) ;
#4762=CARTESIAN_POINT ( 'NONE',  ( -51.96382246819224093, 12.83266463571058580, 4.369925997604237722 ) ) ;
#4769=CARTESIAN_POINT ( 'NONE',  ( -46.91947222136995066, 25.25986047197467599, 1.801467191766157327 ) ) ;
#4770=EDGE_CURVE ( 'NONE', #35416, #37188, #30059, .T. ) ;
#4771=AXIS2_PLACEMENT_3D ( 'NONE', #25997, #3229, #6216 ) ;
#4773=CARTESIAN_POINT ( 'NONE',  ( -57.35932467317038430, 1.578336987915054834, -0.2403330148844060599 ) ) ;
#4776=CARTESIAN_POINT ( 'NONE',  ( -17.14500000000466784, 71.11999999999886768, -1.270000000000000684 ) ) ;
#4778=CARTESIAN_POINT ( 'NONE',  ( -5.591489108514605455, 77.73497692594764885, -1.523999999999996025 ) ) ;
#4783=CARTESIAN_POINT ( 'NONE',  ( -58.16194989728257525, 1.772972946764567181, 0.08436090182516464697 ) ) ;
#4787=CARTESIAN_POINT ( 'NONE',  ( -57.80205714066466527, 2.371715784325115095, -1.753227392946310026 ) ) ;
#4788=ORIENTED_EDGE ( 'NONE', *, *, #19029, .F. ) ;
#4789=CARTESIAN_POINT ( 'NONE',  ( -44.81960200543956319, 21.09415034429482461, -3.442746975522120945 ) ) ;
#4796=CARTESIAN_POINT ( 'NONE',  ( -49.70193759272228107, 16.76737306193518151, -4.987092963739070406 ) ) ;
#4797=ORIENTED_EDGE ( 'NONE', *, *, #35842, .F. ) ;
#4800=CARTESIAN_POINT ( 'NONE',  ( -56.17224506125053551, 4.400912353714958591, -2.358402907739791221 ) ) ;
#4803=CARTESIAN_POINT ( 'NONE',  ( -44.90991502375803890, 23.16658271142636139, -2.247441098035906748 ) ) ;
#4804=EDGE_CURVE ( 'NONE', #28149, #21592, #10993, .T. ) ;
#4806=DIRECTION ( 'NONE',  ( -0.8745520943968235761, 0.4849315768086558398, -8.537024980200821818E-16 ) ) ;
#4807=EDGE_LOOP ( 'NONE', ( #6821, #24873, #35145, #39081 ) ) ;
#4811=CARTESIAN_POINT ( 'NONE',  ( -53.00789483126595769, 12.40033530745290236, -4.180047681284821515 ) ) ;
#4812=DIRECTION ( 'NONE',  ( -5.188838149069472160E-16, 1.699382548006136559E-16, 1.000000000000000000 ) ) ;
#4817=AXIS2_PLACEMENT_3D ( 'NONE', #13260, #32862, #30078 ) ;
#4821=EDGE_CURVE ( 'NONE', #4600, #39773, #30674, .T. ) ;
#4822=CARTESIAN_POINT ( 'NONE',  ( -15.37877921309976870, 79.99470228764801050, -1.270000000000001350 ) ) ;
#4824=CARTESIAN_POINT ( 'NONE',  ( -15.27962295839633811, 80.49293118800726177, 1.269999999999997797 ) ) ;
#4826=CARTESIAN_POINT ( 'NONE',  ( -57.61542428582638564, 1.103772655929896596, 0.1998674755708474138 ) ) ;
#4829=CARTESIAN_POINT ( 'NONE',  ( -46.60530155212501313, 26.17382724835480445, -0.9172222222222309318 ) ) ;
#4837=CARTESIAN_POINT ( 'NONE',  ( -3.841520934845505941, 71.62889921741444255, -1.269999999999994023 ) ) ;
#4843=CARTESIAN_POINT ( 'NONE',  ( -41.95243232931379396, 22.60620181788836192, -1.619729722610462552 ) ) ;
#4844=FACE_OUTER_BOUND ( 'NONE', #16542, .T. ) ;
#4849=CARTESIAN_POINT ( 'NONE',  ( -58.27365357892946918, 0.4699239364167467903, -1.042275140646608422 ) ) ;
#4859=CYLINDRICAL_SURFACE ( 'NONE', #39009, 0.5080000000000007843 ) ;
#4860=EDGE_CURVE ( 'NONE', #22153, #4943, #11292, .T. ) ;
#4864=CARTESIAN_POINT ( 'NONE',  ( -26.51793118801306548, 72.98537704160715123, 1.269999999999993134 ) ) ;
#4865=DIRECTION ( 'NONE',  ( -0.6559537821943239866, 0.7548010569845283735, -4.686333752532408853E-16 ) ) ;
#4869=CARTESIAN_POINT ( 'NONE',  ( -27.97106122948731510, 77.87043919753004673, 1.269999999999991802 ) ) ;
#4872=CARTESIAN_POINT ( 'NONE',  ( -52.74846150007513046, 11.25334410283610254, 3.958079477545757729 ) ) ;
#4873=CARTESIAN_POINT ( 'NONE',  ( -29.42319995517901887, 68.34872547562956413, -1.524000000000006239 ) ) ;
#4876=CARTESIAN_POINT ( 'NONE',  ( -58.73801720703743001, -0.4998429216807459552, -1.049519136981926467E-14 ) ) ;
#4877=CARTESIAN_POINT ( 'NONE',  ( -57.60796681880061243, 1.905299612284082400, 1.725903007441225601 ) ) ;
#4878=LINE ( 'NONE', #8476, #18456 ) ;
#4881=ORIENTED_EDGE ( 'NONE', *, *, #36327, .F. ) ;
#4882=CARTESIAN_POINT ( 'NONE',  ( -54.98111839650035648, 8.542840639972862249, 3.427624633821322320 ) ) ;
#4885=CIRCLE ( 'NONE', #4225, 0.2540000000000000036 ) ;
#4889=ORIENTED_EDGE ( 'NONE', *, *, #25853, .F. ) ;
#4892=CARTESIAN_POINT ( 'NONE',  ( -4.466782427718574588, 71.06098887363195615, -1.523999999999994248 ) ) ;
#4893=CARTESIAN_POINT ( 'NONE',  ( -47.73297240351937631, 19.53746995445935042, 5.217258361112828702 ) ) ;
#4894=CARTESIAN_POINT ( 'NONE',  ( -41.05192305526440322, 23.09448250258610713, 1.270000000023969067 ) ) ;
#4907=CARTESIAN_POINT ( 'NONE',  ( -51.86985193027732066, 10.34936321858913999, 0.3560079035464910335 ) ) ;
#4929=VERTEX_POINT ( 'NONE', #2571 ) ;
#4938=DIRECTION ( 'NONE',  ( -0.8745520943968235761, 0.4849315768086558953, -5.361993529360570985E-16 ) ) ;
#4943=VERTEX_POINT ( 'NONE', #21481 ) ;
#4949=CIRCLE ( 'NONE', #32138, 0.7619999999999969020 ) ;
#4954=CARTESIAN_POINT ( 'NONE',  ( -6.096037513970406607, 78.08166987308820239, 1.524000000000003130 ) ) ;
#4958=DIRECTION ( 'NONE',  ( -0.8745520943968235761, 0.4849315768086558398, -4.268512490100410909E-16 ) ) ;
#4962=ORIENTED_EDGE ( 'NONE', *, *, #26109, .T. ) ;
#4967=CARTESIAN_POINT ( 'NONE',  ( -57.93805369095628777, 0.6893004133205121731, 1.202053765808312802 ) ) ;
#4972=AXIS2_PLACEMENT_3D ( 'NONE', #8251, #2515, #11437 ) ;
#4978=CARTESIAN_POINT ( 'NONE',  ( -57.89731077922510849, 0.5615449381113774008, -0.05962325924458922871 ) ) ;
#4982=DIRECTION ( 'NONE',  ( 5.188838149069472160E-16, -1.699382548006136559E-16, -1.000000000000000000 ) ) ;
#4991=CARTESIAN_POINT ( 'NONE',  ( -58.83227707057483968, -0.08366279997992775996, -0.2458995907045100349 ) ) ;
#4992=VERTEX_POINT ( 'NONE', #24695 ) ;
#4993=CARTESIAN_POINT ( 'NONE',  ( -43.90699889932841415, 21.43881162649502770, -2.872437248222870387 ) ) ;
#4998=VECTOR ( 'NONE', #10634, 1000.000000000000000 ) ;
#5002=CARTESIAN_POINT ( 'NONE',  ( -49.20375664226762069, 17.53306181478205161, -5.082897273857148512 ) ) ;
#5006=CARTESIAN_POINT ( 'NONE',  ( -53.88338131392961827, 9.054548675370849509, -3.507011937191574003 ) ) ;
#5009=CARTESIAN_POINT ( 'NONE',  ( -48.38589991294941939, 19.15920805527091630, -5.452675306770326635 ) ) ;
#5017=CARTESIAN_POINT ( 'NONE',  ( -57.53497731650991653, 2.247686704661286505, -1.882970859819768306 ) ) ;
#5026=DIRECTION ( 'NONE',  ( 0.9998501190848640974, 0.01731298258485272981, 8.537024980200786319E-16 ) ) ;
#5027=CIRCLE ( 'NONE', #20617, 0.2540000000000000036 ) ;
#5028=CARTESIAN_POINT ( 'NONE',  ( -43.13073682054399427, 20.84535665847942454, -0.1327613832364097080 ) ) ;
#5031=CARTESIAN_POINT ( 'NONE',  ( -57.95665747882670615, 0.5159457608236717174, 0.4254811051331099381 ) ) ;
#5032=CARTESIAN_POINT ( 'NONE',  ( -51.27035844764527184, 15.91047978596967560, 4.316378984520650164 ) ) ;
#5035=ORIENTED_EDGE ( 'NONE', *, *, #13479, .T. ) ;
#5036=CARTESIAN_POINT ( 'NONE',  ( -50.06424591225965059, 20.16147316606144813, -2.291703678227673180 ) ) ;
#5040=ORIENTED_EDGE ( 'NONE', *, *, #3988, .F. ) ;
#5048=DIRECTION ( 'NONE',  ( 5.188838149069472160E-16, -1.699382548006136559E-16, -1.000000000000000000 ) ) ;
#5051=CARTESIAN_POINT ( 'NONE',  ( -41.54364448253001285, 22.96340085312751356, -1.538956392779695648 ) ) ;
#5052=VERTEX_POINT ( 'NONE', #37701 ) ;
#5053=PLANE ( 'NONE',  #5060 ) ;
#5054=VERTEX_POINT ( 'NONE', #28103 ) ;
#5056=DIRECTION ( 'NONE',  ( 5.188838149069472160E-16, -1.699382548006136559E-16, -1.000000000000000000 ) ) ;
#5058=CARTESIAN_POINT ( 'NONE',  ( -57.97024931889890809, 0.5691613924952432235, -0.8993266954183887218 ) ) ;
#5060=AXIS2_PLACEMENT_3D ( 'NONE', #27814, #34426, #18212 ) ;
#5069=CARTESIAN_POINT ( 'NONE',  ( -17.14500000000466784, 71.11999999999886768, 1.269999999999998241 ) ) ;
#5070=AXIS2_PLACEMENT_3D ( 'NONE', #39164, #39596, #35340 ) ;
#5075=DIRECTION ( 'NONE',  ( 0.01731298258487879230, -0.9998501190848636533, -9.150538185806814706E-15 ) ) ;
#5083=DIRECTION ( 'NONE',  ( -0.4849315768086535083, -0.8745520943968250194, -1.030032898892974695E-16 ) ) ;
#5084=CARTESIAN_POINT ( 'NONE',  ( -58.36135728304071080, -0.2738979606847323778, 0.1145308973088972754 ) ) ;
#5085=CARTESIAN_POINT ( 'NONE',  ( -28.99046981630712949, 65.28995187595535299, -1.524000000000006017 ) ) ;
#5086=CARTESIAN_POINT ( 'NONE',  ( -52.58202682230450620, 11.88959489689803561, 4.235729473019533842 ) ) ;
#5091=CARTESIAN_POINT ( 'NONE',  ( -49.72660956849071567, 16.83360665160238412, 5.072308565479690223 ) ) ;
#5093=DIRECTION ( 'NONE',  ( -5.188838149069471174E-16, 1.699382548006136313E-16, 1.000000000000000000 ) ) ;
#5101=CARTESIAN_POINT ( 'NONE',  ( -38.65395868481546415, 29.38327706004843876, 1.269999999999994245 ) ) ;
#5102=CARTESIAN_POINT ( 'NONE',  ( -47.60342124589670476, 19.66962190512531805, 5.193532021785222774 ) ) ;
#5103=EDGE_CURVE ( 'NONE', #12049, #35679, #18297, .T. ) ;
#5104=LINE ( 'NONE', #41505, #9955 ) ;
#5108=DIRECTION ( 'NONE',  ( -3.414809992080330305E-15, 0.000000000000000000, 1.000000000000000000 ) ) ;
#5116=CARTESIAN_POINT ( 'NONE',  ( -51.60883138897295908, 11.95321700621929040, 1.992363451474690628 ) ) ;
#5123=EDGE_CURVE ( 'NONE', #24344, #9964, #20759, .T. ) ;
#5124=ORIENTED_EDGE ( 'NONE', *, *, #19889, .T. ) ;
#5129=ORIENTED_EDGE ( 'NONE', *, *, #13651, .T. ) ;
#5137=CARTESIAN_POINT ( 'NONE',  ( -41.97746338594183868, 23.60773098774231826, 1.523999999999994026 ) ) ;
#5141=ORIENTED_EDGE ( 'NONE', *, *, #25593, .T. ) ;
#5162=ORIENTED_EDGE ( 'NONE', *, *, #35780, .T. ) ;
#5176=ORIENTED_EDGE ( 'NONE', *, *, #34877, .F. ) ;
#5180=CARTESIAN_POINT ( 'NONE',  ( -58.58343337229857184, -0.6799398409029571155, 0.1767901212645599796 ) ) ;
#5189=CARTESIAN_POINT ( 'NONE',  ( -57.37715403173692152, 1.618736692213004869, -0.5106765013061207448 ) ) ;
#5191=DIRECTION ( 'NONE',  ( 5.188838149069472160E-16, -1.699382548006136559E-16, -1.000000000000000000 ) ) ;
#5193=LINE ( 'NONE', #8580, #29733 ) ;
#5197=CARTESIAN_POINT ( 'NONE',  ( -58.82991074935231524, -0.2577531494038359794, -1.058401375502683064E-14 ) ) ;
#5200=VERTEX_POINT ( 'NONE', #15315 ) ;
#5201=CARTESIAN_POINT ( 'NONE',  ( -58.21785149106106871, 1.559091779220117546, -0.3785645914143067059 ) ) ;
#5202=ORIENTED_EDGE ( 'NONE', *, *, #35747, .F. ) ;
#5203=CARTESIAN_POINT ( 'NONE',  ( -46.34235131104743743, 20.67093754025578534, -4.736928721793741914 ) ) ;
#5210=CARTESIAN_POINT ( 'NONE',  ( -49.91180784202388310, 16.43617519331882804, -4.943574328148589991 ) ) ;
#5211=ORIENTED_EDGE ( 'NONE', *, *, #2760, .T. ) ;
#5212=AXIS2_PLACEMENT_3D ( 'NONE', #11950, #28562, #34546 ) ;
#5214=DIRECTION ( 'NONE',  ( -0.8745520943968240202, 0.4849315768086553402, -5.361993529360572958E-16 ) ) ;
#5216=CARTESIAN_POINT ( 'NONE',  ( -56.64449391386203558, 3.408586874113735288, -2.059255000246300149 ) ) ;
#5219=CARTESIAN_POINT ( 'NONE',  ( -54.98111839650035648, 8.542840639972862249, -3.427624633821342304 ) ) ;
#5222=VERTEX_POINT ( 'NONE', #25124 ) ;
#5226=CARTESIAN_POINT ( 'NONE',  ( -57.85534701229748578, 0.8496279762696679061, -1.203237356453227047 ) ) ;
#5232=DIRECTION ( 'NONE',  ( 0.9998501190848629872, 0.01731298258490743258, 8.537024980200819846E-16 ) ) ;
#5237=DIRECTION ( 'NONE',  ( 5.188838149069472160E-16, -1.699382548006136559E-16, -1.000000000000000000 ) ) ;
#5238=CARTESIAN_POINT ( 'NONE',  ( -57.60038635073814817, 1.097546858218806376, -1.001372043670648409E-14 ) ) ;
#5239=CARTESIAN_POINT ( 'NONE',  ( -48.81380759447691275, 19.38479668107215304, 4.754960688114458378 ) ) ;
#5242=CARTESIAN_POINT ( 'NONE',  ( -47.36975192132249646, 22.26287704218617236, -3.814390537888114441 ) ) ;
#5244=CARTESIAN_POINT ( 'NONE',  ( -23.91048590848665967, 81.84235438443283783, 1.269999999999993801 ) ) ;
#5245=ORIENTED_EDGE ( 'NONE', *, *, #12340, .T. ) ;
#5257=CARTESIAN_POINT ( 'NONE',  ( -44.94860098973432372, 21.36157941369687308, -3.600951499729750704 ) ) ;
#5262=CARTESIAN_POINT ( 'NONE',  ( -35.99603394726484851, 64.04701136959550922, 1.523999999999990029 ) ) ;
#5264=CARTESIAN_POINT ( 'NONE',  ( -58.21232023750493312, 0.08677210334285366533, -0.8315773506267210013 ) ) ;
#5270=EDGE_CURVE ( 'NONE', #4943, #14176, #28686, .T. ) ;
#5273=AXIS2_PLACEMENT_3D ( 'NONE', #12456, #39074, #6483 ) ;
#5278=EDGE_CURVE ( 'NONE', #19512, #3855, #16360, .T. ) ;
#5279=ORIENTED_EDGE ( 'NONE', *, *, #7178, .F. ) ;
#5289=EDGE_CURVE ( 'NONE', #8441, #23676, #21186, .T. ) ;
#5291=CARTESIAN_POINT ( 'NONE',  ( -58.36255351679519521, -0.2764007135021583905, 0.1060264582682535484 ) ) ;
#5292=EDGE_CURVE ( 'NONE', #41065, #30610, #19972, .T. ) ;
#5295=CARTESIAN_POINT ( 'NONE',  ( -24.32950799593924884, 77.42192949967211746, -1.270000000000005569 ) ) ;
#5296=AXIS2_PLACEMENT_3D ( 'NONE', #1105, #26226, #20667 ) ;
#5298=CARTESIAN_POINT ( 'NONE',  ( -47.65206802627297833, 20.46304711373551299, 5.210715034831059356 ) ) ;
#5303=CARTESIAN_POINT ( 'NONE',  ( -5.369399562154598904, 64.90898011766716991, 1.270000000000005569 ) ) ;
#5308=CARTESIAN_POINT ( 'NONE',  ( -30.83281893200567936, 55.49295607027229238, 1.269999999999994467 ) ) ;
#5310=CARTESIAN_POINT ( 'NONE',  ( -47.98391741143318256, 19.46693557046443246, 5.364172754690429201 ) ) ;
#5322=CARTESIAN_POINT ( 'NONE',  ( -57.43023524350843445, 1.739013888464230329, 1.477089945056089704 ) ) ;
#5333=CARTESIAN_POINT ( 'NONE',  ( -30.45812239790965492, 71.16801738242446618, 1.269999999999990470 ) ) ;
#5335=EDGE_CURVE ( 'NONE', #37322, #28854, #3004, .T. ) ;
#5337=CARTESIAN_POINT ( 'NONE',  ( -3.909619041219702495, 60.89059347946586342, -1.269999999999992024 ) ) ;
#5353=EDGE_CURVE ( 'NONE', #22436, #16174, #26797, .T. ) ;
#5354=CARTESIAN_POINT ( 'NONE',  ( -53.63638764239521350, 11.23543775674477807, 3.971736527645110648 ) ) ;
#5355=CARTESIAN_POINT ( 'NONE',  ( -15.77830307927088249, 80.39606975582424297, -1.524000000000001798 ) ) ;
#5358=CARTESIAN_POINT ( 'NONE',  ( -26.37263903973852663, 72.23735686029533554, -1.524000000000005794 ) ) ;
#5371=ORIENTED_EDGE ( 'NONE', *, *, #4575, .F. ) ;
#5372=CARTESIAN_POINT ( 'NONE',  ( -41.33672448130794663, 22.78954268934618810, 1.170983984347486961 ) ) ;
#5386=CIRCLE ( 'NONE', #18269, 0.6349999999999993427 ) ;
#5388=CARTESIAN_POINT ( 'NONE',  ( -48.44802435119614614, 18.63281525352784129, 5.198089189977588731 ) ) ;
#5396=CARTESIAN_POINT ( 'NONE',  ( -56.89469692534096623, 2.545995565645275960, -0.6470027801917211940 ) ) ;
#5404=CARTESIAN_POINT ( 'NONE',  ( -23.34387769576312621, 77.71194901948682343, -1.270000000000005125 ) ) ;
#5408=CARTESIAN_POINT ( 'NONE',  ( -58.26284211471887176, 1.387681237079871455, -0.7239480823116948294 ) ) ;
#5410=ORIENTED_EDGE ( 'NONE', *, *, #27398, .F. ) ;
#5418=CARTESIAN_POINT ( 'NONE',  ( -49.90791155052789918, 16.44236289295141873, -4.944395792362849207 ) ) ;
#5421=CARTESIAN_POINT ( 'NONE',  ( -17.14500000000466784, 71.11999999999886768, -1.270000000000000684 ) ) ;
#5423=CARTESIAN_POINT ( 'NONE',  ( -51.00679592072113877, 14.45111400903523169, -4.539175725115415005 ) ) ;
#5426=CARTESIAN_POINT ( 'NONE',  ( -52.50198181065980663, 11.96455506022023307, -4.263607785004590589 ) ) ;
#5428=ORIENTED_EDGE ( 'NONE', *, *, #19832, .F. ) ;
#5432=CARTESIAN_POINT ( 'NONE',  ( -58.24807683554808335, 1.288543178753334573, -1.357556113208963744 ) ) ;
#5437=CIRCLE ( 'NONE', #20363, 0.5080000000000014504 ) ;
#5441=CARTESIAN_POINT ( 'NONE',  ( -41.05189575270516400, 23.09451173561988213, -0.9172222222222270460 ) ) ;
#5442=ORIENTED_EDGE ( 'NONE', *, *, #38816, .F. ) ;
#5444=CARTESIAN_POINT ( 'NONE',  ( -23.91048590848665611, 81.84235438443283783, -1.270000000000006235 ) ) ;
#5445=CARTESIAN_POINT ( 'NONE',  ( -38.65395868481546415, 29.38327706004843876, -1.270000000000004903 ) ) ;
#5446=CARTESIAN_POINT ( 'NONE',  ( -52.43464216530867361, 18.97776253654341616, 0.3470174342361194708 ) ) ;
#5449=CARTESIAN_POINT ( 'NONE',  ( -48.26009918843823954, 20.16784055841990764, -4.711418872450288120 ) ) ;
#5460=DIRECTION ( 'NONE',  ( -5.188838149069472160E-16, 1.699382548006136559E-16, 1.000000000000000000 ) ) ;
#5463=DIRECTION ( 'NONE',  ( 0.9807655518882955059, -0.1951894777626270172, 8.537024980200854359E-16 ) ) ;
#5475=ORIENTED_EDGE ( 'NONE', *, *, #32093, .T. ) ;
#5479=LINE ( 'NONE', #37217, #23356 ) ;
#5481=FACE_OUTER_BOUND ( 'NONE', #32919, .T. ) ;
#5482=ORIENTED_EDGE ( 'NONE', *, *, #29960, .F. ) ;
#5485=AXIS2_PLACEMENT_3D ( 'NONE', #1085, #8088, #10443 ) ;
#5493=CARTESIAN_POINT ( 'NONE',  ( -58.05284929258671411, 0.3898940286592555982, 0.7867345219013538449 ) ) ;
#5495=CIRCLE ( 'NONE', #29299, 0.2539999999999956737 ) ;
#5496=EDGE_CURVE ( 'NONE', #41032, #12622, #5711, .T. ) ;
#5497=ADVANCED_FACE ( 'NONE', ( #9875 ), #26122, .T. ) ;
#5502=CARTESIAN_POINT ( 'NONE',  ( -49.66210360255988832, 16.76989353321783227, 4.946330335750482199 ) ) ;
#5506=CARTESIAN_POINT ( 'NONE',  ( -19.86616884172038766, 72.62886460123898758, 1.523999999999996691 ) ) ;
#5507=AXIS2_PLACEMENT_3D ( 'NONE', #15024, #2277, #34429 ) ;
#5511=CARTESIAN_POINT ( 'NONE',  ( -30.83281893229463932, 55.49295607038747846, 1.523999999999994914 ) ) ;
#5512=CARTESIAN_POINT ( 'NONE',  ( -41.08172402297500270, 23.06268970576013189, -1.270028526666295621 ) ) ;
#5514=CARTESIAN_POINT ( 'NONE',  ( -41.05189575270519242, 23.09451173561980042, 1.269999999999989582 ) ) ;
#5516=CYLINDRICAL_SURFACE ( 'NONE', #34093, 0.2539999999999942859 ) ;
#5527=CARTESIAN_POINT ( 'NONE',  ( -55.03835892454119261, 5.996057868307938854, 1.012875379724323288 ) ) ;
#5531=VERTEX_POINT ( 'NONE', #947 ) ;
#5536=VERTEX_POINT ( 'NONE', #19664 ) ;
#5540=AXIS2_PLACEMENT_3D ( 'NONE', #20060, #13686, #33081 ) ;
#5541=DIRECTION ( 'NONE',  ( 5.188838149069472160E-16, -1.699382548006136559E-16, -1.000000000000000000 ) ) ;
#5548=CARTESIAN_POINT ( 'NONE',  ( -41.26650320839694785, 23.23696823412480583, -1.524000000000005128 ) ) ;
#5549=EDGE_CURVE ( 'NONE', #16059, #22469, #1632, .T. ) ;
#5551=ORIENTED_EDGE ( 'NONE', *, *, #15474, .F. ) ;
#5552=EDGE_LOOP ( 'NONE', ( #27301, #37486, #19163, #32871 ) ) ;
#5557=AXIS2_PLACEMENT_3D ( 'NONE', #24369, #4812, #18182 ) ;
#5571=ORIENTED_EDGE ( 'NONE', *, *, #14629, .F. ) ;
#5577=VECTOR ( 'NONE', #19668, 1000.000000000000227 ) ;
#5579=ORIENTED_EDGE ( 'NONE', *, *, #31004, .T. ) ;
#5580=ORIENTED_EDGE ( 'NONE', *, *, #34715, .F. ) ;
#5591=CARTESIAN_POINT ( 'NONE',  ( -29.48103325898055971, 60.42855201934086296, 1.523999999999994026 ) ) ;
#5597=CARTESIAN_POINT ( 'NONE',  ( -4.466782427718574588, 71.06098887363195615, -1.269999999999994245 ) ) ;
#5598=EDGE_CURVE ( 'NONE', #27342, #23556, #41098, .T. ) ;
#5600=ADVANCED_FACE ( 'NONE', ( #26272 ), #8525, .F. ) ;
#5601=CARTESIAN_POINT ( 'NONE',  ( -57.99063839910164830, 1.082714195262735046, 1.370926835928194976 ) ) ;
#5604=DIRECTION ( 'NONE',  ( 5.188838149069472160E-16, -1.699382548006136559E-16, -1.000000000000000000 ) ) ;
#5611=CARTESIAN_POINT ( 'NONE',  ( -57.51979792895002674, 1.380172231454854348, -0.6550001595470087423 ) ) ;
#5615=DIRECTION ( 'NONE',  ( -5.188838149069471174E-16, 1.699382548006136313E-16, 1.000000000000000000 ) ) ;
#5623=CARTESIAN_POINT ( 'NONE',  ( -58.40930376703802551, 1.028767233150276628, -0.4283228411258474533 ) ) ;
#5624=ORIENTED_EDGE ( 'NONE', *, *, #2230, .F. ) ;
#5632=CARTESIAN_POINT ( 'NONE',  ( -58.17229861323505702, 0.6892682111524470745, -1.169530247053243821 ) ) ;
#5633=EDGE_CURVE ( 'NONE', #2940, #2461, #33618, .T. ) ;
#5636=DIRECTION ( 'NONE',  ( -0.8745520943968243532, 0.4849315768086547296, -6.829619984160642269E-16 ) ) ;
#5638=CARTESIAN_POINT ( 'NONE',  ( -54.63495462180135576, 7.558260771377723231, -3.173136904912474243 ) ) ;
#5641=CARTESIAN_POINT ( 'NONE',  ( -56.34046819891496938, 4.202508019718290022, -2.501728563949862760 ) ) ;
#5645=ORIENTED_EDGE ( 'NONE', *, *, #34502, .T. ) ;
#5650=CARTESIAN_POINT ( 'NONE',  ( -57.15088083682995546, 2.378576142695001838, -1.865916551128065981 ) ) ;
#5651=AXIS2_PLACEMENT_3D ( 'NONE', #21369, #34196, #5655 ) ;
#5652=EDGE_CURVE ( 'NONE', #31966, #35910, #20082, .T. ) ;
#5655=DIRECTION ( 'NONE',  ( -0.8745520943968230210, 0.4849315768086570611, -6.829619984160674809E-16 ) ) ;
#5658=DIRECTION ( 'NONE',  ( -0.01731298258489111577, 0.9998501190848634312, 2.778415991487939406E-15 ) ) ;
#5659=CARTESIAN_POINT ( 'NONE',  ( -6.096037513970406607, 78.08166987308820239, -1.269999999999996243 ) ) ;
#5662=CARTESIAN_POINT ( 'NONE',  ( -36.98328822617348521, 27.82293856516311692, 1.269999999999995577 ) ) ;
#5663=DIRECTION ( 'NONE',  ( 0.3582377630123966261, -0.9336303900108832154, 0.000000000000000000 ) ) ;
#5664=CIRCLE ( 'NONE', #40359, 0.3810000000000000053 ) ;
#5666=CARTESIAN_POINT ( 'NONE',  ( -50.19988854512629217, 18.36332526648348917, 3.854797337117271017 ) ) ;
#5669=CARTESIAN_POINT ( 'NONE',  ( -49.65119436432973998, 19.91503915004672720, -3.137105223390908471 ) ) ;
#5671=LINE ( 'NONE', #31633, #35316 ) ;
#5672=ORIENTED_EDGE ( 'NONE', *, *, #29504, .F. ) ;
#5683=CARTESIAN_POINT ( 'NONE',  ( -38.65395868481546415, 29.38327706004843876, 1.269999999999994245 ) ) ;
#5684=FACE_OUTER_BOUND ( 'NONE', #13749, .T. ) ;
#5685=VERTEX_POINT ( 'NONE', #26491 ) ;
#5687=DIRECTION ( 'NONE',  ( -0.9998239923360758841, 0.01876124593811817620, 8.953619244849184656E-16 ) ) ;
#5699=CARTESIAN_POINT ( 'NONE',  ( -41.18107378286554621, 22.95619949144852967, -1.523999999999998023 ) ) ;
#5700=CIRCLE ( 'NONE', #14515, 0.2539999999999998925 ) ;
#5711=B_SPLINE_CURVE_WITH_KNOTS ( 'NONE', 3,
 ( #26167, #9976, #2978, #22950, #38751, #10188, #420, #35976, #32782, #26377, #7015, #19983, #3828, #12756, #25541, #16792, #9560, #22319, #32146, #15942, #28937, #10821, #17623, #27432, #30625, #16998, #30209, #40028, #10404, #33632, #8051, #837, #17211, #14425, #36824, #13812, #33838, #37233, #14012, #1049, #26810, #39601, #17417, #36615, #40239, #27019, #24015, #39818, #20812, #4249, #1468, #24222, #20601, #33418, #23804, #13602, #26592, #27226, #23376, #40446, #11238, #10611, #36409, #20392, #632, #4460, #21024, #7642, #7227, #23593, #30414, #11034, #34047, #7851, #37034, #1262, #4877, #20186, #14217, #7434, #29793, #33212, #4666, #4037, #29998, #31835, #25233, #6075, #16048, #18830, #9464, #1677, #8255, #22428, #2674, #25851, #14632, #35047, #15632, #3089, #28636, #41648, #12455, #38656, #38237, #5868, #6279, #25449, #22222, #15427, #35251, #38860, #5086, #35457, #11440, #38447, #34257, #41436, #9263, #41862, #35672, #28428, #12241, #19037, #12865, #18038, #29051, #37433, #27634, #22018, #30830, #40645, #9053, #32043, #31039, #2880, #15842, #28849, #12659, #25649, #19249, #24428, #21227, #32260, #42069, #2464, #9671, #22636, #17832, #109, #13072, #39711, #16895, #26063 ),
 .UNSPECIFIED., .F., .F.,
 ( 4, 2, 2, 2, 1, 2, 2, 1, 2, 2, 1, 2, 2, 2, 1, 2, 2, 2, 1, 2, 2, 2, 1, 1, 2, 2, 2, 2, 1, 1, 2, 2, 2, 2, 1, 1, 1, 2, 2, 2, 2, 2, 1, 1, 1, 1, 2, 2, 2, 2, 2, 1, 1, 1, 2, 2, 2, 2, 2, 1, 1, 1, 1, 1, 2, 2, 2, 1, 1, 1, 2, 2, 2, 1, 1, 1, 1, 1, 1, 2, 2, 2, 2, 2, 1, 1, 1, 1, 2, 2, 2, 1, 1, 1, 2, 2, 4 ),
 ( 0.000000000000000000, 0.001953125000004253542, 0.003906250000008507084, 0.005859375000012760626, 0.006835937500015010562, 0.007324218750016135530, 0.007812500000017260499, 0.008056640625017824284, 0.008178710937518268373, 0.008300781250018712462, 0.008544921875019602375, 0.008666992187520046464, 0.008789062500020490554, 0.009277343750020565147, 0.009521484375020599841, 0.009643554687520533922, 0.009765625000020466268, 0.01074218750001992677, 0.01123046875001975850, 0.01147460937501967523, 0.01171875000001959370, 0.01367187500001920859, 0.01464843750001911492, 0.01513671875001906982, 0.01538085937501904726, 0.01562500000001902645, 0.02343750000001785377, 0.02734375000001739581, 0.02929687500001716682, 0.03027343750001705233, 0.03076171875001698988, 0.03125000000001693090, 0.04687500000001662559, 0.05468750000001662559, 0.05859375000001661865, 0.06054687500001661171, 0.06152343750001676437, 0.06201171875001699335, 0.06250000000001720846, 0.09375000000002055300, 0.1093750000000222322, 0.1171875000000230649, 0.1210937500000234812, 0.1230468750000235784, 0.1240234375000235090, 0.1245117187500235922, 0.1247558593750236478, 0.1250000000000236755, 0.1875000000000396905, 0.2187500000000476563, 0.2343750000000518197, 0.2421875000000539568, 0.2460937500000550116, 0.2480468750000557054, 0.2490234375000561773, 0.2500000000000566769, 0.3750000000001075806, 0.4375000000001327827, 0.4687500000001454947, 0.4843750000001519895, 0.4921875000001553757, 0.4960937500001573186, 0.4980468750001585398, 0.4990234375001590394, 0.4995117187501594280, 0.5000000000001597611, 0.5625000000001978417, 0.5937500000002169376, 0.6093750000002263745, 0.6171875000002311484, 0.6210937500002333689, 0.6250000000002357003, 0.6875000000002793321, 0.7187500000003014256, 0.7343750000003125278, 0.7421875000003183009, 0.7460937500003208545, 0.7480468750003222977, 0.7490234375003230749, 0.7495117187503236300, 0.7500000000003242961, 0.8125000000002705614, 0.8437500000002434719, 0.8593750000002298162, 0.8671875000002228218, 0.8710937500002193801, 0.8730468750002178258, 0.8740234375002170486, 0.8745117187502164935, 0.8750000000002160494, 0.9062500000001612044, 0.9218750000001334488, 0.9296875000001197931, 0.9335937500001127987, 0.9355468750001096900, 0.9375000000001064704, 1.000000000000000000 ),
 .UNSPECIFIED. ) ;
#5712=CARTESIAN_POINT ( 'NONE',  ( -5.639506490940112471, 64.42185452804264401, -1.523999999999993582 ) ) ;
#5713=CARTESIAN_POINT ( 'NONE',  ( -57.93978974282668304, 0.6351742460125603396, 0.9371179993346451242 ) ) ;
#5714=CARTESIAN_POINT ( 'NONE',  ( -8.594951744493888768, 74.76616009375631222, 1.524000000000002464 ) ) ;
#5717=VERTEX_POINT ( 'NONE', #33105 ) ;
#5718=CARTESIAN_POINT ( 'NONE',  ( -47.67648637180144533, 19.71513033058998232, 5.327979952964769339 ) ) ;
#5723=CARTESIAN_POINT ( 'NONE',  ( -29.04966993600562830, 66.62533279660628693, 1.523999999999992916 ) ) ;
#5727=CARTESIAN_POINT ( 'NONE',  ( -29.78720458926533965, 57.91457584465491948, 1.523999999999994026 ) ) ;
#5728=CARTESIAN_POINT ( 'NONE',  ( -41.06680163122255323, 23.07855206975608553, -1.270000052244677269 ) ) ;
#5729=FACE_OUTER_BOUND ( 'NONE', #34176, .T. ) ;
#5730=AXIS2_PLACEMENT_3D ( 'NONE', #23695, #10301, #27331 ) ;
#5731=DIRECTION ( 'NONE',  ( -0.8572391118119460085, -0.5149185422762189157, -3.573031421855289661E-16 ) ) ;
#5743=EDGE_LOOP ( 'NONE', ( #7863, #9841, #15969, #38792 ) ) ;
#5744=CARTESIAN_POINT ( 'NONE',  ( -55.77633192430580777, 4.649224570933515821, 0.8844362032702561827 ) ) ;
#5760=CARTESIAN_POINT ( 'NONE',  ( -46.91715763656851124, 25.27325160652277347, 1.792044074526565778 ) ) ;
#5761=CARTESIAN_POINT ( 'NONE',  ( -46.60530155212501313, 26.17382724835480445, 0.9172222222222133903 ) ) ;
#5763=CARTESIAN_POINT ( 'NONE',  ( -43.83556092231052048, 21.45200552150719631, 2.811646013901242025 ) ) ;
#5766=EDGE_LOOP ( 'NONE', ( #38103, #42066, #18579, #34671 ) ) ;
#5767=CYLINDRICAL_SURFACE ( 'NONE', #41815, 0.2539999999999973390 ) ;
#5771=CARTESIAN_POINT ( 'NONE',  ( -46.60530155212503445, 26.17382724835477958, -1.524000000000008237 ) ) ;
#5783=ORIENTED_EDGE ( 'NONE', *, *, #21007, .T. ) ;
#5789=ORIENTED_EDGE ( 'NONE', *, *, #19811, .F. ) ;
#5791=CARTESIAN_POINT ( 'NONE',  ( -27.10368288468284348, 75.59070314479281194, 1.523999999999992916 ) ) ;
#5800=EDGE_CURVE ( 'NONE', #12982, #7108, #29898, .T. ) ;
#5806=DIRECTION ( 'NONE',  ( 0.3256999990547876367, 0.9454731675810326141, 8.328397965208553695E-18 ) ) ;
#5808=CARTESIAN_POINT ( 'NONE',  ( -58.60951264191312049, -0.2527965749330313150, 0.4344104473664969213 ) ) ;
#5809=ADVANCED_FACE ( 'NONE', ( #33526 ), #41774, .T. ) ;
#5817=AXIS2_PLACEMENT_3D ( 'NONE', #2743, #19107, #29118 ) ;
#5825=CARTESIAN_POINT ( 'NONE',  ( -10.39456080247343905, 81.94606122948148652, 1.524000000000000465 ) ) ;
#5826=LINE ( 'NONE', #27750, #18847 ) ;
#5827=EDGE_CURVE ( 'NONE', #6380, #30889, #15223, .T. ) ;
#5830=ORIENTED_EDGE ( 'NONE', *, *, #2746, .T. ) ;
#5831=CARTESIAN_POINT ( 'NONE',  ( -58.46425016648313999, 0.8496528882456222398, -0.7404953295986963502 ) ) ;
#5834=CARTESIAN_POINT ( 'NONE',  ( -43.11180532272962296, 21.58876176643009615, -2.074236749942713232 ) ) ;
#5838=EDGE_CURVE ( 'NONE', #26546, #20056, #8427, .T. ) ;
#5842=CARTESIAN_POINT ( 'NONE',  ( -55.34422897054474788, 6.609666497766444770, -3.132814435880084680 ) ) ;
#5843=ORIENTED_EDGE ( 'NONE', *, *, #38086, .F. ) ;
#5847=DIRECTION ( 'NONE',  ( -5.188838149069472160E-16, 1.699382548006136559E-16, 1.000000000000000000 ) ) ;
#5850=CARTESIAN_POINT ( 'NONE',  ( -51.58367816905025194, 14.91232437457545146, -4.609044670965841917 ) ) ;
#5853=ORIENTED_EDGE ( 'NONE', *, *, #27124, .F. ) ;
#5857=CARTESIAN_POINT ( 'NONE',  ( -58.60752282809816904, -0.1920500713008393978, -0.6598870774482961110 ) ) ;
#5863=DIRECTION ( 'NONE',  ( 0.6559537821943239866, -0.7548010569845283735, 4.686333752532408853E-16 ) ) ;
#5864=CARTESIAN_POINT ( 'NONE',  ( -47.69647088358534148, 18.57426963660985209, -3.960430087866680271 ) ) ;
#5867=CARTESIAN_POINT ( 'NONE',  ( -58.43690671596436914, -0.4125963578781866037, 0.2423173958219003998 ) ) ;
#5868=CARTESIAN_POINT ( 'NONE',  ( -53.84250820861786480, 9.549132715125418613, 3.786023059759871412 ) ) ;
#5869=CYLINDRICAL_SURFACE ( 'NONE', #6629, 0.5080000000000000071 ) ;
#5871=CARTESIAN_POINT ( 'NONE',  ( -52.70911355518960306, 14.14937146821753444, 3.349573991549116059 ) ) ;
#5874=CARTESIAN_POINT ( 'NONE',  ( -49.10997966587441965, 20.64911895071488956, -3.108984601230539990 ) ) ;
#5887=CARTESIAN_POINT ( 'NONE',  ( -36.65473259702431363, 28.27472347546386544, -1.524000000000003574 ) ) ;
#5906=VECTOR ( 'NONE', #37668, 1000.000000000000114 ) ;
#5909=EDGE_LOOP ( 'NONE', ( #36788, #29258, #23926, #22409 ) ) ;
#5912=CARTESIAN_POINT ( 'NONE',  ( -46.38316532014830784, 26.05065462784526176, -1.524000000000014676 ) ) ;
#5918=CARTESIAN_POINT ( 'NONE',  ( -58.36373456865217690, -0.2788725735744660983, 0.09695730896412824151 ) ) ;
#5919=VECTOR ( 'NONE', #8561, 1000.000000000000000 ) ;
#5921=CARTESIAN_POINT ( 'NONE',  ( -23.14542444889682571, 82.37908244650444090, -1.524000000000005794 ) ) ;
#5926=CIRCLE ( 'NONE', #23587, 0.2540000000000000036 ) ;
#5928=CARTESIAN_POINT ( 'NONE',  ( -41.23752580366542020, 23.26788267949596190, 1.523999999999992916 ) ) ;
#5937=CARTESIAN_POINT ( 'NONE',  ( -6.401666570281891566, 64.12941061790216679, 1.270000000000005125 ) ) ;
#5949=CARTESIAN_POINT ( 'NONE',  ( -57.26476250566310711, 1.946856395439316989, 1.045107959733424074 ) ) ;
#5954=AXIS2_PLACEMENT_3D ( 'NONE', #8859, #15448, #35271 ) ;
#5957=ORIENTED_EDGE ( 'NONE', *, *, #39249, .F. ) ;
#5959=DIRECTION ( 'NONE',  ( 0.9998501190848635423, 0.01731298258488073519, 5.158639060800513087E-16 ) ) ;
#5965=CARTESIAN_POINT ( 'NONE',  ( -46.83932897938335316, 25.61700229504076631, 1.554731942900158259 ) ) ;
#5966=CARTESIAN_POINT ( 'NONE',  ( -46.67361288142431164, 26.04169289900193363, 0.9171659260646253253 ) ) ;
#5968=CARTESIAN_POINT ( 'NONE',  ( -48.21404017327530767, 19.06235592689615288, 5.351320745402585288 ) ) ;
#5971=ORIENTED_EDGE ( 'NONE', *, *, #29037, .F. ) ;
#5981=CARTESIAN_POINT ( 'NONE',  ( -5.591535794131393899, 65.03215273817657760, 1.524000000000005572 ) ) ;
#5996=VERTEX_POINT ( 'NONE', #22994 ) ;
#5997=ORIENTED_EDGE ( 'NONE', *, *, #14599, .T. ) ;
#6010=ORIENTED_EDGE ( 'NONE', *, *, #20468, .F. ) ;
#6020=ADVANCED_FACE ( 'NONE', ( #36021 ), #881, .T. ) ;
#6030=DIRECTION ( 'NONE',  ( -5.188838149069471174E-16, 1.699382548006136313E-16, 1.000000000000000000 ) ) ;
#6033=CARTESIAN_POINT ( 'NONE',  ( -41.25198653392084935, 23.25239942703034046, 1.523999999999994248 ) ) ;
#6035=EDGE_CURVE ( 'NONE', #15131, #15945, #25434, .T. ) ;
#6041=CARTESIAN_POINT ( 'NONE',  ( -41.77909418348673398, 22.73884196981018491, -1.565812447105877192 ) ) ;
#6046=CARTESIAN_POINT ( 'NONE',  ( -57.53431004061603460, 2.062971833132837496, -1.787249339056213637 ) ) ;
#6047=ORIENTED_EDGE ( 'NONE', *, *, #261, .F. ) ;
#6048=CARTESIAN_POINT ( 'NONE',  ( -58.34514637059952236, -0.2398883667948381593, -0.1955437934783339493 ) ) ;
#6055=AXIS2_PLACEMENT_3D ( 'NONE', #41594, #12403, #35614 ) ;
#6057=CARTESIAN_POINT ( 'NONE',  ( -53.17586183559576085, 10.67386474145934372, -4.017225210190888518 ) ) ;
#6063=ADVANCED_FACE ( 'NONE', ( #33296 ), #27098, .T. ) ;
#6064=CARTESIAN_POINT ( 'NONE',  ( -57.60038635073814817, 1.097546858218806376, -1.033898108845213542E-14 ) ) ;
#6067=CARTESIAN_POINT ( 'NONE',  ( -47.10086694477701030, 25.28009754958737787, 1.863548351650762491 ) ) ;
#6070=DIRECTION ( 'NONE',  ( -0.01731298258487873332, 0.9998501190848635423, -9.050832817465997210E-15 ) ) ;
#6072=CARTESIAN_POINT ( 'NONE',  ( -48.84381969468221030, 17.12102923570560975, -3.921819500614954102 ) ) ;
#6074=CARTESIAN_POINT ( 'NONE',  ( -10.57002714855771863, 82.40335727708655611, 1.269999999999999796 ) ) ;
#6075=CARTESIAN_POINT ( 'NONE',  ( -56.45305112249246093, 4.342240606964129945, 2.533486158674154165 ) ) ;
#6076=CARTESIAN_POINT ( 'NONE',  ( -29.88458269586515925, 69.13647124293702007, -1.270000000000007123 ) ) ;
#6078=CARTESIAN_POINT ( 'NONE',  ( -53.73190450750161773, 11.39902669490613896, 3.613030284815563764 ) ) ;
#6080=ORIENTED_EDGE ( 'NONE', *, *, #40749, .T. ) ;
#6081=CARTESIAN_POINT ( 'NONE',  ( -50.19988854512629217, 18.36332526648348917, -3.854797337117289224 ) ) ;
#6095=CARTESIAN_POINT ( 'NONE',  ( -4.085839532347236513, 71.06758511999679229, -1.523999999999994026 ) ) ;
#6096=EDGE_CURVE ( 'NONE', #16976, #21597, #30866, .T. ) ;
#6097=FACE_OUTER_BOUND ( 'NONE', #1294, .T. ) ;
#6101=CARTESIAN_POINT ( 'NONE',  ( -58.36736542105735026, -0.2864936770574270097, -0.06035461783101484651 ) ) ;
#6111=VECTOR ( 'NONE', #27402, 1000.000000000000000 ) ;
#6113=AXIS2_PLACEMENT_3D ( 'NONE', #13664, #37094, #4731 ) ;
#6115=CARTESIAN_POINT ( 'NONE',  ( -47.71508057896579658, 20.49549959222711593, -5.111566084959475731 ) ) ;
#6119=EDGE_CURVE ( 'NONE', #22153, #37301, #40606, .T. ) ;
#6120=CARTESIAN_POINT ( 'NONE',  ( -5.878298779570172883, 78.21245918282636467, 1.270000000000002904 ) ) ;
#6122=ADVANCED_FACE ( 'NONE', ( #13690 ), #25634, .T. ) ;
#6126=LINE ( 'NONE', #19091, #7004 ) ;
#6131=ORIENTED_EDGE ( 'NONE', *, *, #29960, .T. ) ;
#6139=CARTESIAN_POINT ( 'NONE',  ( -30.29872984390849311, 56.23795811431430280, 1.523999999999994026 ) ) ;
#6142=DIRECTION ( 'NONE',  ( 0.4849315768086535638, 0.8745520943968251304, 1.030032898892975065E-16 ) ) ;
#6164=ADVANCED_FACE ( 'NONE', ( #30499, #1130 ), #24312, .T. ) ;
#6165=LINE ( 'NONE', #38330, #749 ) ;
#6168=CARTESIAN_POINT ( 'NONE',  ( -46.82598356868722789, 25.66206020625350348, 1.525368666045084032 ) ) ;
#6169=CARTESIAN_POINT ( 'NONE',  ( -46.72476011081990066, 26.09744872113180847, 0.08471799968938857617 ) ) ;
#6170=AXIS2_PLACEMENT_3D ( 'NONE', #9533, #32536, #19529 ) ;
#6172=CARTESIAN_POINT ( 'NONE',  ( -47.71508057896579658, 20.49549959222711593, 5.111566084959459744 ) ) ;
#6175=ORIENTED_EDGE ( 'NONE', *, *, #15168, .F. ) ;
#6180=AXIS2_PLACEMENT_3D ( 'NONE', #31773, #22156, #31347 ) ;
#6194=VERTEX_POINT ( 'NONE', #39898 ) ;
#6202=DIRECTION ( 'NONE',  ( 0.8745520943968243532, -0.4849315768086547296, 6.829619984160642269E-16 ) ) ;
#6211=CIRCLE ( 'NONE', #29995, 0.3809999999999984510 ) ;
#6216=DIRECTION ( 'NONE',  ( -0.7548010569845180484, -0.6559537821943359770, 0.000000000000000000 ) ) ;
#6217=AXIS2_PLACEMENT_3D ( 'NONE', #41108, #28523, #8303 ) ;
#6224=DIRECTION ( 'NONE',  ( -0.8745520943968235761, 0.4849315768086558398, -4.268512490100410909E-16 ) ) ;
#6234=CIRCLE ( 'NONE', #799, 0.2539999999999932867 ) ;
#6241=VERTEX_POINT ( 'NONE', #7517 ) ;
#6244=CARTESIAN_POINT ( 'NONE',  ( -41.09670346151852982, 23.04688172093031895, -1.270085369932521191 ) ) ;
#6250=CARTESIAN_POINT ( 'NONE',  ( -57.65317970594307440, 1.808445652233532597, -1.687761604364059309 ) ) ;
#6251=ORIENTED_EDGE ( 'NONE', *, *, #32887, .F. ) ;
#6252=CARTESIAN_POINT ( 'NONE',  ( -58.39415239746203667, -0.3126312442486959831, -0.4522786855619334023 ) ) ;
#6258=CARTESIAN_POINT ( 'NONE',  ( -58.11258158571958177, 1.603013069906233934, -1.501710181103033781 ) ) ;
#6259=EDGE_LOOP ( 'NONE', ( #29322, #37213, #8376, #41871, #8928 ) ) ;
#6265=VECTOR ( 'NONE', #18986, 1000.000000000000114 ) ;
#6267=AXIS2_PLACEMENT_3D ( 'NONE', #23486, #17110, #30111 ) ;
#6268=CARTESIAN_POINT ( 'NONE',  ( -56.42856387642239469, 3.193865871111076338, -9.978765949893178940E-15 ) ) ;
#6274=DIRECTION ( 'NONE',  ( -0.3256999990547930768, -0.9454731675810308378, -6.956556933070078754E-15 ) ) ;
#6275=CARTESIAN_POINT ( 'NONE',  ( -47.93564525088159201, 15.36257551998192916, -0.4079155175245698373 ) ) ;
#6278=CARTESIAN_POINT ( 'NONE',  ( -46.73847652112046092, 25.90099053509251092, -1.386667892818581160 ) ) ;
#6279=CARTESIAN_POINT ( 'NONE',  ( -53.84203694985585287, 9.550030682661965642, 3.786207223046024861 ) ) ;
#6281=CARTESIAN_POINT ( 'NONE',  ( -12.79279280188648116, 63.69337819391066091, 1.524000000000002242 ) ) ;
#6283=CARTESIAN_POINT ( 'NONE',  ( -55.74683331106318462, 9.129907917338066170, 0.4890489271862150100 ) ) ;
#6285=EDGE_LOOP ( 'NONE', ( #208, #36050, #31648, #20253 ) ) ;
#6287=CARTESIAN_POINT ( 'NONE',  ( -51.24266872689721453, 19.11669921072455836, -1.581762766848686885 ) ) ;
#6298=CARTESIAN_POINT ( 'NONE',  ( -29.82321757229076908, 71.17901112636586447, -1.524000000000007349 ) ) ;
#6304=ORIENTED_EDGE ( 'NONE', *, *, #33905, .F. ) ;
#6305=CARTESIAN_POINT ( 'NONE',  ( -58.36849006653898897, -0.2888454140588792018, -0.04296944658959341024 ) ) ;
#6316=DIRECTION ( 'NONE',  ( -0.6294287539884059202, -0.7770581983690814099, -1.945484789722797322E-16 ) ) ;
#6318=CARTESIAN_POINT ( 'NONE',  ( -46.82679756180435504, 21.08486709759267086, -4.907624977305287572 ) ) ;
#6322=DIRECTION ( 'NONE',  ( 5.188838149069472160E-16, -1.699382548006136559E-16, -1.000000000000000000 ) ) ;
#6323=CIRCLE ( 'NONE', #23964, 9.048749999999998295 ) ;
#6330=CARTESIAN_POINT ( 'NONE',  ( -58.37002191173434795, -0.2919876190278939410, 0.009343179624763268964 ) ) ;
#6331=AXIS2_PLACEMENT_3D ( 'NONE', #29319, #22690, #19507 ) ;
#6339=DIRECTION ( 'NONE',  ( 0.8745520943968235761, -0.4849315768086558398, 4.268512490100410909E-16 ) ) ;
#6349=EDGE_CURVE ( 'NONE', #32297, #10071, #8639, .T. ) ;
#6356=ADVANCED_FACE ( 'NONE', ( #1342 ), #27310, .T. ) ;
#6360=DIRECTION ( 'NONE',  ( -0.8745520943968235761, 0.4849315768086558953, -5.361993529360570985E-16 ) ) ;
#6370=AXIS2_PLACEMENT_3D ( 'NONE', #32696, #16276, #28864 ) ;
#6371=CARTESIAN_POINT ( 'NONE',  ( -47.96057925449625259, 19.24834700699408074, 5.203605657935928441 ) ) ;
#6372=CARTESIAN_POINT ( 'NONE',  ( -47.29848140234559395, 25.70219632838243484, -8.387873617975133388E-15 ) ) ;
#6374=ORIENTED_EDGE ( 'NONE', *, *, #27979, .F. ) ;
#6375=CARTESIAN_POINT ( 'NONE',  ( -42.34481381083929818, 23.19759442052183473, 1.554397948409609542 ) ) ;
#6376=DIRECTION ( 'NONE',  ( 0.9876665170007969952, -0.1565721916417935344, 5.390917751951444915E-16 ) ) ;
#6380=VERTEX_POINT ( 'NONE', #34554 ) ;
#6386=CARTESIAN_POINT ( 'NONE',  ( -36.79765817521327165, 27.64956762128695900, -1.524000000000003574 ) ) ;
#6388=VECTOR ( 'NONE', #33681, 1000.000000000000000 ) ;
#6391=CARTESIAN_POINT ( 'NONE',  ( -30.15642192025596202, 71.36377005712995469, 1.523999999999991806 ) ) ;
#6395=CARTESIAN_POINT ( 'NONE',  ( -9.795036404550218734, 65.29837086945681790, 1.270000000000003126 ) ) ;
#6398=VERTEX_POINT ( 'NONE', #12170 ) ;
#6399=DIRECTION ( 'NONE',  ( 0.01731298258488073519, -0.9998501190848635423, 1.788962107505278613E-16 ) ) ;
#6401=TOROIDAL_SURFACE ( 'NONE', #18632, 3.111499999999999488, 0.2540000000000000036 ) ;
#6406=ORIENTED_EDGE ( 'NONE', *, *, #20468, .T. ) ;
#6408=CARTESIAN_POINT ( 'NONE',  ( -41.41491986784954804, 22.70581808553406233, -4.778348942345147220E-15 ) ) ;
#6415=DIRECTION ( 'NONE',  ( -0.8745520943968383420, 0.4849315768086291945, -4.268512490100416826E-16 ) ) ;
#6419=ORIENTED_EDGE ( 'NONE', *, *, #34237, .F. ) ;
#6420=DIRECTION ( 'NONE',  ( 0.8745520943968243532, -0.4849315768086547296, 6.829619984160642269E-16 ) ) ;
#6424=CARTESIAN_POINT ( 'NONE',  ( -7.994219716368544226, 68.36415334912796027, 1.524000000000003796 ) ) ;
#6439=CARTESIAN_POINT ( 'NONE',  ( -27.82636559844506152, 59.51700088791086074, 1.523999999999995136 ) ) ;
#6445=CARTESIAN_POINT ( 'NONE',  ( -29.94429436251954613, 71.80236127745905605, -1.270000000000007345 ) ) ;
#6447=ORIENTED_EDGE ( 'NONE', *, *, #27512, .F. ) ;
#6452=EDGE_CURVE ( 'NONE', #36699, #16976, #38569, .T. ) ;
#6454=CARTESIAN_POINT ( 'NONE',  ( -58.17661517772558000, 0.6798812134844969268, -1.164281364473555236 ) ) ;
#6455=VERTEX_POINT ( 'NONE', #34343 ) ;
#6456=CARTESIAN_POINT ( 'NONE',  ( -58.33447198145992729, -0.2173903971933038859, -0.2351149084157238001 ) ) ;
#6460=CARTESIAN_POINT ( 'NONE',  ( -30.75918919842648336, 69.77432548395512413, -1.524000000000007793 ) ) ;
#6463=CARTESIAN_POINT ( 'NONE',  ( -58.37241122568488549, -0.2962816677227753104, -1.034007718770489626E-14 ) ) ;
#6464=VERTEX_POINT ( 'NONE', #40940 ) ;
#6474=CARTESIAN_POINT ( 'NONE',  ( -46.48504882798792437, 25.86691234155606267, 1.523999999999993804 ) ) ;
#6477=CARTESIAN_POINT ( 'NONE',  ( -17.14500000000466784, 71.11999999999886768, 1.269999999999998241 ) ) ;
#6478=CARTESIAN_POINT ( 'NONE',  ( -46.29506748884625011, 20.38262349295737152, -4.279265904994571379 ) ) ;
#6479=ORIENTED_EDGE ( 'NONE', *, *, #11106, .T. ) ;
#6481=CARTESIAN_POINT ( 'NONE',  ( -28.92060043785469503, 77.33101988233063651, -1.270000000000007789 ) ) ;
#6483=DIRECTION ( 'NONE',  ( -0.1565721916417901483, -0.9876665170007974393, 0.000000000000000000 ) ) ;
#6485=CARTESIAN_POINT ( 'NONE',  ( -55.24575511360199442, 11.19612964283759560, -1.042979010729945558E-14 ) ) ;
#6486=CARTESIAN_POINT ( 'NONE',  ( -56.71132732703541990, 3.319205314284062958, 2.191228219141345246 ) ) ;
#6488=ORIENTED_EDGE ( 'NONE', *, *, #35842, .T. ) ;
#6489=CARTESIAN_POINT ( 'NONE',  ( -55.59033409382031721, 8.645621179197947370, -1.431546819705167284 ) ) ;
#6504=DIRECTION ( 'NONE',  ( 0.1565721916418034709, 0.9876665170007954409, -8.659954811667512579E-17 ) ) ;
#6505=ORIENTED_EDGE ( 'NONE', *, *, #37792, .F. ) ;
#6506=AXIS2_PLACEMENT_3D ( 'NONE', #26986, #10788, #3583 ) ;
#6509=CARTESIAN_POINT ( 'NONE',  ( -23.69188486464780752, 78.08202335040543574, -1.270000000000005347 ) ) ;
#6518=VERTEX_POINT ( 'NONE', #38166 ) ;
#6522=CARTESIAN_POINT ( 'NONE',  ( -46.81005371095109524, 25.73327194510133253, -1.583310528698488984 ) ) ;
#6523=ORIENTED_EDGE ( 'NONE', *, *, #27979, .T. ) ;
#6525=DIRECTION ( 'NONE',  ( 0.4849315768086535638, 0.8745520943968251304, 1.030032898892975065E-16 ) ) ;
#6526=CARTESIAN_POINT ( 'NONE',  ( -17.31000046771894318, 62.32679794340116786, -1.523999999999999577 ) ) ;
#6530=AXIS2_PLACEMENT_3D ( 'NONE', #20616, #33647, #30429 ) ;
#6532=EDGE_CURVE ( 'NONE', #27477, #19390, #27672, .T. ) ;
#6534=DIRECTION ( 'NONE',  ( 0.9454731675810360558, -0.3256999990547780888, 5.459396135145339171E-16 ) ) ;
#6543=FACE_OUTER_BOUND ( 'NONE', #11218, .T. ) ;
#6546=VERTEX_POINT ( 'NONE', #2182 ) ;
#6550=DIRECTION ( 'NONE',  ( -5.188838149069472160E-16, 1.699382548006136559E-16, 1.000000000000000000 ) ) ;
#6554=DIRECTION ( 'NONE',  ( -0.8745520943968235761, 0.4849315768086558398, -4.268512490100410909E-16 ) ) ;
#6559=TOROIDAL_SURFACE ( 'NONE', #15395, 0.7620000000000000107, 0.2540000000000000036 ) ;
#6562=EDGE_CURVE ( 'NONE', #13695, #23403, #28570, .T. ) ;
#6567=CARTESIAN_POINT ( 'NONE',  ( -20.21600168833980149, 80.16988503754176065, -1.524000000000003796 ) ) ;
#6571=DIRECTION ( 'NONE',  ( 0.7284927773988482125, 0.6850534820564830873, 0.000000000000000000 ) ) ;
#6572=DIRECTION ( 'NONE',  ( -0.9336303900108808840, -0.3582377630124027879, -2.618564950574899336E-15 ) ) ;
#6574=EDGE_CURVE ( 'NONE', #2316, #35792, #37892, .T. ) ;
#6577=CIRCLE ( 'NONE', #22977, 0.2539999999999942859 ) ;
#6578=CARTESIAN_POINT ( 'NONE',  ( -46.60530155212503445, 26.17382724835477958, 1.269999999999988916 ) ) ;
#6582=CARTESIAN_POINT ( 'NONE',  ( -43.49527490626578441, 22.26612824116996237, 2.150709692269567874 ) ) ;
#6583=CARTESIAN_POINT ( 'NONE',  ( -23.16987411132078378, 77.52691185402750307, -1.270000000000004903 ) ) ;
#6585=CARTESIAN_POINT ( 'NONE',  ( -58.37241122568487128, -0.2962816677227753104, -0.2416009568454013656 ) ) ;
#6587=ORIENTED_EDGE ( 'NONE', *, *, #21078, .F. ) ;
#6604=ORIENTED_EDGE ( 'NONE', *, *, #32666, .F. ) ;
#6609=CIRCLE ( 'NONE', #30402, 0.6350000000000006750 ) ;
#6613=ORIENTED_EDGE ( 'NONE', *, *, #10010, .F. ) ;
#6615=CARTESIAN_POINT ( 'NONE',  ( -42.04356058215219605, 22.06167541775167606, 0.4953331422233907544 ) ) ;
#6623=CARTESIAN_POINT ( 'NONE',  ( -47.87720502863936645, 19.40776447661573911, -5.264800451520500246 ) ) ;
#6628=ADVANCED_FACE ( 'NONE', ( #37949 ), #23580, .T. ) ;
#6629=AXIS2_PLACEMENT_3D ( 'NONE', #28429, #25017, #30985 ) ;
#6630=ORIENTED_EDGE ( 'NONE', *, *, #40223, .F. ) ;
#6633=CARTESIAN_POINT ( 'NONE',  ( -58.65598178207972779, -0.3163282088989305407, 0.3245478190976838206 ) ) ;
#6634=DIRECTION ( 'NONE',  ( 0.9734199927291312671, 0.2290273297124563179, 2.762079339012820083E-15 ) ) ;
#6636=EDGE_CURVE ( 'NONE', #14176, #37301, #34756, .T. ) ;
#6658=EDGE_LOOP ( 'NONE', ( #13680, #4709, #27962, #14755 ) ) ;
#6666=CARTESIAN_POINT ( 'NONE',  ( -58.61347569670156332, -0.2600004252125417414, -0.4230615130465681939 ) ) ;
#6670=CARTESIAN_POINT ( 'NONE',  ( 0.000000000000000000, 0.000000000000000000, 0.000000000000000000 ) ) ;
#6672=CARTESIAN_POINT ( 'NONE',  ( -8.210443557797230341, 69.68696903609419735, 1.270000000000003348 ) ) ;
#6675=CARTESIAN_POINT ( 'NONE',  ( -57.24023649071029496, 3.661034843983918208, -2.195083147259570211 ) ) ;
#6687=EDGE_CURVE ( 'NONE', #34378, #25039, #2607, .T. ) ;
#6690=CARTESIAN_POINT ( 'NONE',  ( -28.69846420587789737, 77.20784726182124302, -1.524000000000007793 ) ) ;
#6691=CARTESIAN_POINT ( 'NONE',  ( -48.74330358230356808, 18.21177412086844072, -5.147861347727202386 ) ) ;
#6694=CARTESIAN_POINT ( 'NONE',  ( -46.75070351170987237, 25.87126803027572564, -1.402526684451548267 ) ) ;
#6699=DIRECTION ( 'NONE',  ( -0.8745520943968240202, 0.4849315768086553402, -5.361993529360572958E-16 ) ) ;
#6700=CARTESIAN_POINT ( 'NONE',  ( -57.73934301000005576, 2.737667398473711433, 1.050169850737047383 ) ) ;
#6701=CARTESIAN_POINT ( 'NONE',  ( -58.23017998949752183, 0.6774554162835566551, 1.209604144815701554 ) ) ;
#6704=CARTESIAN_POINT ( 'NONE',  ( -50.15972161391663064, 17.13814111569222121, -4.955022299345084313 ) ) ;
#6707=ORIENTED_EDGE ( 'NONE', *, *, #20858, .F. ) ;
#6717=CARTESIAN_POINT ( 'NONE',  ( -47.97335965025877869, 19.24887047013930541, -5.222717875959610900 ) ) ;
#6718=CARTESIAN_POINT ( 'NONE',  ( -18.63562586887613648, 79.95981838582228818, 1.269999999999996243 ) ) ;
#6721=ORIENTED_EDGE ( 'NONE', *, *, #27207, .F. ) ;
#6727=VECTOR ( 'NONE', #267, 1000.000000000000000 ) ;
#6733=EDGE_LOOP ( 'NONE', ( #18442, #39213, #1751, #34116 ) ) ;
#6736=DIRECTION ( 'NONE',  ( -0.8572391118119510045, -0.5149185422762100339, -3.573031421855330583E-16 ) ) ;
#6737=CARTESIAN_POINT ( 'NONE',  ( -48.21404017327530767, 19.06235592689615288, -5.351320745402601275 ) ) ;
#6738=VERTEX_POINT ( 'NONE', #26204 ) ;
#6741=AXIS2_PLACEMENT_3D ( 'NONE', #30105, #9873, #39708 ) ;
#6743=DIRECTION ( 'NONE',  ( 0.8572391118119522258, 0.5149185422762083686, -1.192944345661028856E-14 ) ) ;
#6749=FACE_OUTER_BOUND ( 'NONE', #34102, .T. ) ;
#6758=ORIENTED_EDGE ( 'NONE', *, *, #14924, .F. ) ;
#6764=AXIS2_PLACEMENT_3D ( 'NONE', #10714, #27116, #36928 ) ;
#6768=CIRCLE ( 'NONE', #14383, 0.6350000000000006750 ) ;
#6773=ORIENTED_EDGE ( 'NONE', *, *, #6119, .T. ) ;
#6776=DIRECTION ( 'NONE',  ( -5.188838149069471174E-16, 1.699382548006136313E-16, 1.000000000000000000 ) ) ;
#6778=ORIENTED_EDGE ( 'NONE', *, *, #20866, .F. ) ;
#6780=CARTESIAN_POINT ( 'NONE',  ( -8.265412277504241345, 72.86149316418863009, 1.270000000000002682 ) ) ;
#6783=EDGE_CURVE ( 'NONE', #6518, #38326, #6609, .T. ) ;
#6787=AXIS2_PLACEMENT_3D ( 'NONE', #33807, #17591, #20156 ) ;
#6789=CARTESIAN_POINT ( 'NONE',  ( -46.76084739749286712, 25.84593537448104428, 1.416306353842238908 ) ) ;
#6790=CARTESIAN_POINT ( 'NONE',  ( -47.62964748377234514, 25.45032632311202647, 0.1281092358103023410 ) ) ;
#6792=CARTESIAN_POINT ( 'NONE',  ( -56.65231406860745977, 4.194353530936431262, 2.518504496425231221 ) ) ;
#6795=CARTESIAN_POINT ( 'NONE',  ( -58.35029634831491308, -0.2563984898762833309, -0.1830726351724966949 ) ) ;
#6802=CARTESIAN_POINT ( 'NONE',  ( -46.86699512455117400, 25.83114541775341522, -0.4845221143632307825 ) ) ;
#6814=CARTESIAN_POINT ( 'NONE',  ( -17.14500000000466784, 71.11999999999886768, -1.270000000000000684 ) ) ;
#6820=EDGE_CURVE ( 'NONE', #537, #8461, #17478, .T. ) ;
#6821=ORIENTED_EDGE ( 'NONE', *, *, #36185, .F. ) ;
#6823=CARTESIAN_POINT ( 'NONE',  ( -41.40170217118274110, 22.71997040916441080, 0.2118088196526822786 ) ) ;
#6830=DIRECTION ( 'NONE',  ( 5.188838149069472160E-16, -1.699382548006136559E-16, -1.000000000000000000 ) ) ;
#6834=ORIENTED_EDGE ( 'NONE', *, *, #29629, .F. ) ;
#6836=DIRECTION ( 'NONE',  ( 0.8745520943968235761, -0.4849315768086558398, 4.268512490100410909E-16 ) ) ;
#6837=CARTESIAN_POINT ( 'NONE',  ( -11.17805678602830355, 77.92260723867444483, -1.269999999999998685 ) ) ;
#6839=EDGE_CURVE ( 'NONE', #33608, #30025, #13380, .T. ) ;
#6846=LINE ( 'NONE', #30255, #21488 ) ;
#6854=DIRECTION ( 'NONE',  ( -5.188838149069472160E-16, 1.699382548006136559E-16, 1.000000000000000000 ) ) ;
#6855=CARTESIAN_POINT ( 'NONE',  ( -10.18297664959815663, 77.66688486464208552, 1.270000000000000906 ) ) ;
#6858=DIRECTION ( 'NONE',  ( -5.188838149069471174E-16, 1.699382548006136313E-16, 1.000000000000000000 ) ) ;
#6864=ORIENTED_EDGE ( 'NONE', *, *, #39363, .F. ) ;
#6865=CARTESIAN_POINT ( 'NONE',  ( -4.085839532347240066, 71.06758511999679229, 1.270000000000005125 ) ) ;
#6866=EDGE_LOOP ( 'NONE', ( #30246, #2506, #24545, #15629 ) ) ;
#6870=AXIS2_PLACEMENT_3D ( 'NONE', #34227, #5056, #31216 ) ;
#6874=CARTESIAN_POINT ( 'NONE',  ( -58.53126320289103290, -0.08783021930335940808, -0.6231558322867893907 ) ) ;
#6875=ORIENTED_EDGE ( 'NONE', *, *, #3821, .F. ) ;
#6876=CARTESIAN_POINT ( 'NONE',  ( -24.50334120614357047, 81.61487340491997600, -1.270000000000006457 ) ) ;
#6882=EDGE_CURVE ( 'NONE', #21011, #15033, #35167, .T. ) ;
#6884=AXIS2_PLACEMENT_3D ( 'NONE', #29412, #23420, #25789 ) ;
#6886=CARTESIAN_POINT ( 'NONE',  ( -57.85534701229748578, 0.8496279762696679061, -1.203237356453227047 ) ) ;
#6887=EDGE_CURVE ( 'NONE', #16766, #35632, #16600, .T. ) ;
#6895=CARTESIAN_POINT ( 'NONE',  ( -44.40685758373556524, 19.43703734468909516, -6.894256627225939810E-15 ) ) ;
#6899=AXIS2_PLACEMENT_3D ( 'NONE', #27846, #34667, #18457 ) ;
#6902=CARTESIAN_POINT ( 'NONE',  ( -30.37855815223275258, 71.48694267763936239, 1.269999999999992246 ) ) ;
#6903=CARTESIAN_POINT ( 'NONE',  ( -52.42931032121356338, 11.92852722686772005, -4.179465640474091970 ) ) ;
#6908=CARTESIAN_POINT ( 'NONE',  ( -31.37023363772181028, 53.64958092169537451, 1.269999999999992912 ) ) ;
#6913=CARTESIAN_POINT ( 'NONE',  ( -56.26154134542980501, 7.775270144418685803, -1.045335966129298087E-14 ) ) ;
#6914=CARTESIAN_POINT ( 'NONE',  ( -57.52317756609133426, 3.014644041894651405, 1.981665235817938076 ) ) ;
#6916=EDGE_CURVE ( 'NONE', #2842, #35121, #28861, .T. ) ;
#6917=ORIENTED_EDGE ( 'NONE', *, *, #16774, .T. ) ;
#6918=CARTESIAN_POINT ( 'NONE',  ( -51.41777536269126614, 18.15702087101736595, -2.173118852595011141 ) ) ;
#6935=ORIENTED_EDGE ( 'NONE', *, *, #36185, .T. ) ;
#6944=AXIS2_PLACEMENT_3D ( 'NONE', #3299, #13507, #6699 ) ;
#6945=ADVANCED_FACE ( 'NONE', ( #3021 ), #39058, .T. ) ;
#6947=ADVANCED_FACE ( 'NONE', ( #15977 ), #6401, .T. ) ;
#6954=CARTESIAN_POINT ( 'NONE',  ( -43.24646561529713296, 21.63922848039483071, -2.381786957946274264 ) ) ;
#6979=DIRECTION ( 'NONE',  ( 0.6594218222380416883, 0.7517731442105793915, 0.000000000000000000 ) ) ;
#6987=CARTESIAN_POINT ( 'NONE',  ( -23.91048590848665967, 81.84235438443283783, 1.523999999999993138 ) ) ;
#6991=EDGE_CURVE ( 'NONE', #6464, #20372, #38582, .T. ) ;
#6992=EDGE_LOOP ( 'NONE', ( #28561, #6587, #30343, #18853 ) ) ;
#6997=CARTESIAN_POINT ( 'NONE',  ( -47.19240717248583650, 20.04893757306883018, 5.078271723504655277 ) ) ;
#6999=DIRECTION ( 'NONE',  ( -0.8745520943968240202, 0.4849315768086551737, -5.361993529360572958E-16 ) ) ;
#7000=VERTEX_POINT ( 'NONE', #39000 ) ;
#7004=VECTOR ( 'NONE', #9931, 1000.000000000000000 ) ;
#7007=AXIS2_PLACEMENT_3D ( 'NONE', #35820, #30407, #1256 ) ;
#7010=CARTESIAN_POINT ( 'NONE',  ( -46.69016964900118438, 26.00918483878763254, 1.334034565177987242 ) ) ;
#7011=CARTESIAN_POINT ( 'NONE',  ( -47.48049929620759002, 23.18975938597035125, 2.730405167055922178 ) ) ;
#7014=CARTESIAN_POINT ( 'NONE',  ( -51.73272837791831336, 13.19950324185369794, 4.393710239503571202 ) ) ;
#7015=CARTESIAN_POINT ( 'NONE',  ( -58.70326665360445872, -0.3146233719498078840, 0.2858976903834491434 ) ) ;
#7019=CARTESIAN_POINT ( 'NONE',  ( -42.34481381083929818, 23.19759442052183473, 1.554397948409609542 ) ) ;
#7026=CARTESIAN_POINT ( 'NONE',  ( -36.79765817521327165, 27.64956762128695900, -1.270000000000003570 ) ) ;
#7031=CARTESIAN_POINT ( 'NONE',  ( -36.98328822617348521, 27.82293856516311692, -1.524000000000003796 ) ) ;
#7035=CARTESIAN_POINT ( 'NONE',  ( -30.19451713491628198, 70.61549828015995445, 1.523999999999992028 ) ) ;
#7042=ORIENTED_EDGE ( 'NONE', *, *, #39334, .F. ) ;
#7043=CARTESIAN_POINT ( 'NONE',  ( -42.12253153191133492, 21.94389511927448311, -4.944039522370902375E-15 ) ) ;
#7057=AXIS2_PLACEMENT_3D ( 'NONE', #25916, #13141, #22911 ) ;
#7058=CARTESIAN_POINT ( 'NONE',  ( -23.97640303682767993, 76.49434496853974963, 1.523999999999994026 ) ) ;
#7077=CARTESIAN_POINT ( 'NONE',  ( -48.28978369826177186, 19.63653578263564015, -5.206999999995405304 ) ) ;
#7078=FACE_OUTER_BOUND ( 'NONE', #9304, .T. ) ;
#7082=EDGE_CURVE ( 'NONE', #37511, #33280, #21428, .T. ) ;
#7085=CARTESIAN_POINT ( 'NONE',  ( -5.885917553499152355, 77.12042444889114279, -1.269999999999996021 ) ) ;
#7086=ORIENTED_EDGE ( 'NONE', *, *, #1140, .T. ) ;
#7088=TOROIDAL_SURFACE ( 'NONE', #20680, 0.7620000000000000107, 0.2540000000000000036 ) ;
#7094=CARTESIAN_POINT ( 'NONE',  ( -58.58102607532369888, -0.1934477224862401756, -0.5095094156256858575 ) ) ;
#7096=CARTESIAN_POINT ( 'NONE',  ( -58.34682947232719386, -0.2434262655763713701, -0.1887554165967095521 ) ) ;
#7102=CARTESIAN_POINT ( 'NONE',  ( -57.22363667057550884, 2.289652018204080264, -1.875138655370660379 ) ) ;
#7103=CIRCLE ( 'NONE', #26116, 0.2539999999999990599 ) ;
#7106=ADVANCED_FACE ( 'NONE', ( #23412 ), #4705, .T. ) ;
#7108=VERTEX_POINT ( 'NONE', #874 ) ;
#7112=CARTESIAN_POINT ( 'NONE',  ( -58.34556966141487067, -0.2407783058111234720, 0.1938516799453078032 ) ) ;
#7123=CARTESIAN_POINT ( 'NONE',  ( -53.80167111242602118, 9.145755618221249605, -3.362987294923143633 ) ) ;
#7127=CARTESIAN_POINT ( 'NONE',  ( -17.09698261757901960, 84.43312239790384410, -1.524000000000002908 ) ) ;
#7128=CARTESIAN_POINT ( 'NONE',  ( -7.772068811996249771, 69.25462295839062676, 1.270000000000003570 ) ) ;
#7130=DIRECTION ( 'NONE',  ( -0.8745520943968247973, 0.4849315768086537304, -5.361993529360573944E-16 ) ) ;
#7131=CARTESIAN_POINT ( 'NONE',  ( -57.87117896969294861, 2.397448601660856493, 0.9757051360025592590 ) ) ;
#7132=CARTESIAN_POINT ( 'NONE',  ( -57.92346726745822849, 0.7446056814934959300, 1.206286704679851107 ) ) ;
#7135=CARTESIAN_POINT ( 'NONE',  ( -56.90927647567382763, 5.206763508130138440, -0.7605795637955022892 ) ) ;
#7137=EDGE_LOOP ( 'NONE', ( #28874, #22453, #40225, #13213 ) ) ;
#7138=CARTESIAN_POINT ( 'NONE',  ( -14.60888863026623952, 79.54114996201613508, -1.524000000000001132 ) ) ;
#7153=CARTESIAN_POINT ( 'NONE',  ( -57.49410450365485303, 1.597103417522111934, -1.403138785175781944 ) ) ;
#7162=ORIENTED_EDGE ( 'NONE', *, *, #7451, .T. ) ;
#7165=( BOUNDED_SURFACE ( )  B_SPLINE_SURFACE ( 3, 2, ( 
 ( #34066, #14028, #17639 ),
 ( #7450, #17432, #4893 ),
 ( #17848, #5102, #23820 ),
 ( #24240, #30430, #30848 ),
 ( #1484, #10627, #27034 ),
 ( #36629, #40043, #27240 ),
 ( #18054, #27652, #37249 ),
 ( #854, #20407, #10836 ),
 ( #11255, #36840, #7660 ),
 ( #26825, #20618, #40255 ),
 ( #11049, #24035, #40664 ),
 ( #37050, #30641, #40465 ),
 ( #1694, #7868, #20829 ),
 ( #4682, #14440, #27450 ),
 ( #8066, #11455, #24446 ),
 ( #37450, #33437, #34274 ),
 ( #39832, #18683, #22288 ),
 ( #15069, #8696, #41080 ),
 ( #28703, #24658, #15496 ),
 ( #41292, #37872, #15698 ),
 ( #34684, #2741, #14858 ),
 ( #8490, #40870, #28285 ),
 ( #31692, #25298, #31263 ),
 ( #11671, #11888, #27862 ) ),
 .UNSPECIFIED., .F., .F., .F. ) 
 B_SPLINE_SURFACE_WITH_KNOTS ( ( 4, 2, 2, 2, 2, 2, 2, 2, 2, 2, 2, 4 ),
 ( 3, 3 ),
 ( 0.000000000000000000, 0.0005614604826171184235, 0.001122920965234236847, 0.001684381447851355379, 0.002245841930468473694, 0.003368762895702710758, 0.004491683860936947388, 0.005614604826171184018, 0.006737525791405421516, 0.007298986274022539397, 0.007860446756639657279, 0.008983367721873894776 ),
 ( 0.000000000000000000, 1.000000000000000000 ),
 .UNSPECIFIED. ) 
 GEOMETRIC_REPRESENTATION_ITEM ( )  RATIONAL_B_SPLINE_SURFACE ( (
 ( 1.000000000000000000, 0.9987193938133381854, 1.000000000000000000),
 ( 1.000000000000000000, 0.9982000373937082172, 1.000000000000000000),
 ( 1.000000000000000000, 0.9975619604998443579, 1.000000000000000000),
 ( 1.000000000000000000, 0.9916939477420071425, 1.000000000000000000),
 ( 1.000000000000000000, 0.9861209039942885335, 1.000000000000000000),
 ( 1.000000000000000000, 0.9617740169773764114, 1.000000000000000000),
 ( 1.000000000000000000, 0.9448443023870999324, 1.000000000000000000),
 ( 1.000000000000000000, 0.9146158020826528068, 1.000000000000000000),
 ( 1.000000000000000000, 0.9004045293498704750, 1.000000000000000000),
 ( 1.000000000000000000, 0.8619933248295105210, 1.000000000000000000),
 ( 1.000000000000000000, 0.8427343359447093674, 1.000000000000000000),
 ( 1.000000000000000000, 0.8121850874613311122, 1.000000000000000000),
 ( 1.000000000000000000, 0.8005416906224276374, 1.000000000000000000),
 ( 1.000000000000000000, 0.7821458849522040513, 1.000000000000000000),
 ( 1.000000000000000000, 0.7751654015739020132, 1.000000000000000000),
 ( 1.000000000000000000, 0.7626205617125327851, 1.000000000000000000),
 ( 1.000000000000000000, 0.7574054414875175389, 1.000000000000000000),
 ( 1.000000000000000000, 0.7453179101210614110, 1.000000000000000000),
 ( 1.000000000000000000, 0.7405197175301533319, 1.000000000000000000),
 ( 1.000000000000000000, 0.7299770405535720430, 1.000000000000000000),
 ( 1.000000000000000000, 0.7243132446550970549, 1.000000000000000000),
 ( 1.000000000000000000, 0.7087302219116619062, 1.000000000000000000),
 ( 1.000000000000000000, 0.7007553748513319913, 1.000000000000000000),
 ( 1.000000000000000000, 0.7072256012392703628, 1.000000000000000000) ) ) 
 REPRESENTATION_ITEM ( '' )  SURFACE ( )  );
#7168=CARTESIAN_POINT ( 'NONE',  ( -51.54051843738712080, 14.84038450301108192, -4.692172599169433411 ) ) ;
#7178=EDGE_CURVE ( 'NONE', #4929, #26503, #978, .T. ) ;
#7179=CARTESIAN_POINT ( 'NONE',  ( -43.06611735332000279, 21.60822042109159824, -2.043235477782531007 ) ) ;
#7182=LINE ( 'NONE', #11185, #2505 ) ;
#7183=EDGE_CURVE ( 'NONE', #38737, #32933, #35658, .T. ) ;
#7187=CARTESIAN_POINT ( 'NONE',  ( -46.60530155212504155, 26.17382724835477958, -1.270000000000008455 ) ) ;
#7190=EDGE_CURVE ( 'NONE', #22599, #25412, #11165, .T. ) ;
#7202=CARTESIAN_POINT ( 'NONE',  ( -58.60951264191635346, -0.2527965749311716914, -0.4344104473673510713 ) ) ;
#7207=EDGE_LOOP ( 'NONE', ( #14436, #2489, #22808, #3113 ) ) ;
#7210=DIRECTION ( 'NONE',  ( -0.8745520943968253524, 0.4849315768086530087, -8.537024980200771528E-16 ) ) ;
#7211=CARTESIAN_POINT ( 'NONE',  ( -10.84307050033138431, 78.30450799593342026, -1.269999999999998685 ) ) ;
#7212=CIRCLE ( 'NONE', #6530, 0.5080000000000000071 ) ;
#7213=EDGE_LOOP ( 'NONE', ( #16501, #27693, #30758, #5843 ) ) ;
#7216=CARTESIAN_POINT ( 'NONE',  ( -46.78618054628500289, 25.31127283853226828, -1.744542934675088919 ) ) ;
#7222=CARTESIAN_POINT ( 'NONE',  ( -57.91918631225849623, 0.6797522236637953963, 0.9623354101195258359 ) ) ;
#7223=CARTESIAN_POINT ( 'NONE',  ( -47.07934102874912696, 22.98505637820354153, 3.579966862081923828 ) ) ;
#7226=CARTESIAN_POINT ( 'NONE',  ( -55.65298819915649631, 5.540485941798511504, 2.823722248809245272 ) ) ;
#7227=CARTESIAN_POINT ( 'NONE',  ( -57.86763781102449400, 1.347252755066737473, 1.494140885802228924 ) ) ;
#7229=CARTESIAN_POINT ( 'NONE',  ( -58.37241122568488549, -0.2962816677227753104, -1.028586707908062104E-14 ) ) ;
#7231=CARTESIAN_POINT ( 'NONE',  ( -24.23745918283205114, 82.38670122043342303, -1.270000000000006457 ) ) ;
#7241=CARTESIAN_POINT ( 'NONE',  ( -13.99440778436217592, 79.95103047660883533, 1.269999999999998241 ) ) ;
#7242=VECTOR ( 'NONE', #37795, 1000.000000000000000 ) ;
#7253=VERTEX_POINT ( 'NONE', #39155 ) ;
#7254=CARTESIAN_POINT ( 'NONE',  ( -41.35393432493753352, 22.77111593294431913, 0.9171044195162014745 ) ) ;
#7264=EDGE_LOOP ( 'NONE', ( #36160, #19631, #15253, #31115 ) ) ;
#7269=VECTOR ( 'NONE', #22840, 1000.000000000000000 ) ;
#7273=CARTESIAN_POINT ( 'NONE',  ( -17.65389921742010060, 84.42347906515803402, -1.270000000000003348 ) ) ;
#7281=DIRECTION ( 'NONE',  ( -5.188838149069472160E-16, 1.699382548006136559E-16, 1.000000000000000000 ) ) ;
#7283=AXIS2_PLACEMENT_3D ( 'NONE', #39689, #10902, #4124 ) ;
#7289=DIRECTION ( 'NONE',  ( 5.188838149069472160E-16, -1.699382548006136559E-16, -1.000000000000000000 ) ) ;
#7290=DIRECTION ( 'NONE',  ( 0.3256999990547897461, 0.9454731675810318370, 0.000000000000000000 ) ) ;
#7292=ORIENTED_EDGE ( 'NONE', *, *, #14987, .F. ) ;
#7298=CARTESIAN_POINT ( 'NONE',  ( -58.61721026093515263, -0.2672633658392670197, -0.4124697875294594529 ) ) ;
#7299=EDGE_LOOP ( 'NONE', ( #2818, #30961, #41985, #9159 ) ) ;
#7300=DIRECTION ( 'NONE',  ( 0.000000000000000000, 0.000000000000000000, 1.000000000000000000 ) ) ;
#7301=CIRCLE ( 'NONE', #36553, 0.6349999999999970113 ) ;
#7303=PRESENTATION_STYLE_ASSIGNMENT (( #36482 ) ) ;
#7308=DIRECTION ( 'NONE',  ( 0.9816537812491092918, 0.1906721105965052399, 1.574460549389967402E-15 ) ) ;
#7311=ORIENTED_EDGE ( 'NONE', *, *, #23787, .T. ) ;
#7315=CARTESIAN_POINT ( 'NONE',  ( -47.84756666395260538, 19.38928433903618043, 5.209054514891976240 ) ) ;
#7324=CARTESIAN_POINT ( 'NONE',  ( -53.87733401397680666, 8.744676589845553849, -2.811092830483142180 ) ) ;
#7326=DIRECTION ( 'NONE',  ( -0.5149185422762221354, 0.8572391118119438991, -4.128606161907600514E-16 ) ) ;
#7327=FACE_OUTER_BOUND ( 'NONE', #15408, .T. ) ;
#7328=DIRECTION ( 'NONE',  ( -5.188838149069472160E-16, 1.699382548006136559E-16, 1.000000000000000000 ) ) ;
#7329=CARTESIAN_POINT ( 'NONE',  ( -29.24397885281356224, 65.27318422236749029, -1.270000000000006013 ) ) ;
#7332=LINE ( 'NONE', #39715, #26654 ) ;
#7333=CARTESIAN_POINT ( 'NONE',  ( -58.33482727260580702, 1.278009831241974759, -1.064229179957365390E-14 ) ) ;
#7337=CARTESIAN_POINT ( 'NONE',  ( -57.80399136194962040, 2.779771081967835400, -0.2452555687351754832 ) ) ;
#7339=ORIENTED_EDGE ( 'NONE', *, *, #9157, .F. ) ;
#7340=CARTESIAN_POINT ( 'NONE',  ( -14.21338345945963688, 79.68069512491149453, -1.524000000000000909 ) ) ;
#7346=TOROIDAL_SURFACE ( 'NONE', #24999, 0.3810000000000001719, 0.2540000000000000036 ) ;
#7348=CARTESIAN_POINT ( 'NONE',  ( -33.42971872652992005, 49.93539301574497102, 1.269999999999992690 ) ) ;
#7355=CARTESIAN_POINT ( 'NONE',  ( -57.78008333914727501, 0.9803893178324115665, -1.120514846177007584 ) ) ;
#7361=CARTESIAN_POINT ( 'NONE',  ( -48.21404017327530767, 19.06235592689615288, -5.351320745402601275 ) ) ;
#7363=ADVANCED_FACE ( 'NONE', ( #38944 ), #4391, .T. ) ;
#7369=CARTESIAN_POINT ( 'NONE',  ( -24.32950799593924884, 77.42192949967211746, 1.269999999999993578 ) ) ;
#7371=CARTESIAN_POINT ( 'NONE',  ( -50.11792632901008915, 17.09067799859288783, -5.048577231237582730 ) ) ;
#7374=DIRECTION ( 'NONE',  ( -0.5149185422762221354, 0.8572391118119438991, -4.128606161907600514E-16 ) ) ;
#7379=CARTESIAN_POINT ( 'NONE',  ( -45.05484530740422144, 21.03919035317145259, -3.644944174416286042 ) ) ;
#7381=PRODUCT_DEFINITION_CONTEXT ( 'detailed design', #9918, 'design' ) ;
#7382=EDGE_CURVE ( 'NONE', #13050, #8692, #22932, .T. ) ;
#7386=CARTESIAN_POINT ( 'NONE',  ( -46.84426172109978381, 25.74287342672571910, -1.326046531036418452 ) ) ;
#7387=DIRECTION ( 'NONE',  ( -0.8745520943968243532, 0.4849315768086547296, -5.361993529360573944E-16 ) ) ;
#7397=DIRECTION ( 'NONE',  ( 0.8745520943968235761, -0.4849315768086558398, 4.268512490100410909E-16 ) ) ;
#7404=CARTESIAN_POINT ( 'NONE',  ( -50.01754050906186677, 16.20622680599536025, -4.878148848507119162 ) ) ;
#7405=FACE_OUTER_BOUND ( 'NONE', #32257, .T. ) ;
#7410=ORIENTED_EDGE ( 'NONE', *, *, #13888, .T. ) ;
#7412=EDGE_CURVE ( 'NONE', #41143, #4125, #35328, .T. ) ;
#7427=EDGE_CURVE ( 'NONE', #24767, #30889, #9795, .T. ) ;
#7429=DIRECTION ( 'NONE',  ( -0.1906721105965055174, 0.9816537812491091808, 0.000000000000000000 ) ) ;
#7430=CARTESIAN_POINT ( 'NONE',  ( -53.60911972597136810, 9.592866957671235539, 3.621504120778383129 ) ) ;
#7431=CARTESIAN_POINT ( 'NONE',  ( -47.36975192132250356, 22.26287704218617236, 3.814390537888098009 ) ) ;
#7433=CARTESIAN_POINT ( 'NONE',  ( -49.93490050754573417, 16.96705409125581099, 5.170188367178237598 ) ) ;
#7434=CARTESIAN_POINT ( 'NONE',  ( -57.44836869838920279, 2.247189469432294473, 1.860557060983530686 ) ) ;
#7438=CARTESIAN_POINT ( 'NONE',  ( -46.20552558087364758, 24.41938074005533466, 2.020549794458497139 ) ) ;
#7447=ADVANCED_FACE ( 'NONE', ( #29130 ), #22031, .T. ) ;
#7450=CARTESIAN_POINT ( 'NONE',  ( -47.72307967018315367, 19.52623448395708294, 5.191226814324476635 ) ) ;
#7451=EDGE_CURVE ( 'NONE', #28646, #27727, #17968, .T. ) ;
#7454=CARTESIAN_POINT ( 'NONE',  ( -10.00099186598785472, 77.19260062651656540, -1.269999999999998019 ) ) ;
#7463=CARTESIAN_POINT ( 'NONE',  ( -52.48304539424793091, 11.63526101311008354, 3.802211793135424678 ) ) ;
#7473=FACE_OUTER_BOUND ( 'NONE', #25080, .T. ) ;
#7475=TOROIDAL_SURFACE ( 'NONE', #1356, 0.3810000000000001719, 0.2540000000000000036 ) ;
#7476=ORIENTED_EDGE ( 'NONE', *, *, #20344, .F. ) ;
#7481=DIRECTION ( 'NONE',  ( 0.8745520943968235761, -0.4849315768086558398, 0.000000000000000000 ) ) ;
#7483=CARTESIAN_POINT ( 'NONE',  ( -20.21600168833980149, 80.16988503754176065, -1.270000000000003793 ) ) ;
#7488=ORIENTED_EDGE ( 'NONE', *, *, #11387, .F. ) ;
#7492=CARTESIAN_POINT ( 'NONE',  ( -14.01601067707388992, 79.52082022139843787, 1.269999999999998463 ) ) ;
#7494=DIRECTION ( 'NONE',  ( -0.6294287539883864913, -0.7770581983690970640, 0.000000000000000000 ) ) ;
#7503=CARTESIAN_POINT ( 'NONE',  ( -9.712308604790303335, 65.53852105402241079, 1.270000000000003126 ) ) ;
#7510=CYLINDRICAL_SURFACE ( 'NONE', #32775, 0.2539999999999998925 ) ;
#7512=( LENGTH_UNIT ( ) NAMED_UNIT ( * ) SI_UNIT ( .MILLI., .METRE. ) );
#7514=DIRECTION ( 'NONE',  ( -5.188838149069471174E-16, 1.699382548006136313E-16, 1.000000000000000000 ) ) ;
#7517=CARTESIAN_POINT ( 'NONE',  ( -19.21741104974024594, 79.92823415920659613, 1.269999999999994911 ) ) ;
#7520=ORIENTED_EDGE ( 'NONE', *, *, #24095, .F. ) ;
#7524=CARTESIAN_POINT ( 'NONE',  ( -54.51629495445180140, 7.799846118209302404, 3.232377281230888855 ) ) ;
#7531=DIRECTION ( 'NONE',  ( -0.3582377630123915746, 0.9336303900108851028, -3.445432962228667069E-16 ) ) ;
#7532=CARTESIAN_POINT ( 'NONE',  ( -55.81215269371604393, 4.390389611868092068, -0.4227292597524531792 ) ) ;
#7534=CARTESIAN_POINT ( 'NONE',  ( -15.42835734045148577, 79.74558783746837776, 1.269999999999998019 ) ) ;
#7538=CARTESIAN_POINT ( 'NONE',  ( -29.81988630912367455, 58.80898419537163591, -1.523999999998479460 ) ) ;
#7542=CARTESIAN_POINT ( 'NONE',  ( -14.64596739026573857, 69.73430801926814127, -1.523999999999999355 ) ) ;
#7543=CARTESIAN_POINT ( 'NONE',  ( -58.39046968809522298, 1.092456688167306567, 0.3056578461530140567 ) ) ;
#7547=CARTESIAN_POINT ( 'NONE',  ( -57.97744691355249813, 2.174673694799844625, -0.6577596567056189780 ) ) ;
#7549=ORIENTED_EDGE ( 'NONE', *, *, #28197, .T. ) ;
#7550=FACE_OUTER_BOUND ( 'NONE', #18933, .T. ) ;
#7551=VECTOR ( 'NONE', #32398, 1000.000000000000114 ) ;
#7558=DIRECTION ( 'NONE',  ( -0.8745520943968250194, 0.4849315768086532863, -5.361993529360574930E-16 ) ) ;
#7561=CARTESIAN_POINT ( 'NONE',  ( -29.91360363449003756, 70.04874496952835727, -1.524000000000007349 ) ) ;
#7565=CARTESIAN_POINT ( 'NONE',  ( -57.44712170204855539, 1.698054324899128220, -1.444792672776622267 ) ) ;
#7570=CARTESIAN_POINT ( 'NONE',  ( -45.68084146533627177, 21.25878370237693815, -4.188014402015116211 ) ) ;
#7574=ORIENTED_EDGE ( 'NONE', *, *, #36259, .F. ) ;
#7579=CARTESIAN_POINT ( 'NONE',  ( -54.39768377094780760, 8.094885465611476150, -3.421923752996840928 ) ) ;
#7581=PRODUCT_DEFINITION_SHAPE ( 'NONE', 'NONE',  #10216 ) ;
#7590=CARTESIAN_POINT ( 'NONE',  ( -58.37241122568487128, -0.2962816677227614326, -1.047861413196692856E-14 ) ) ;
#7592=ORIENTED_EDGE ( 'NONE', *, *, #18795, .F. ) ;
#7593=CARTESIAN_POINT ( 'NONE',  ( -48.05879467440716013, 25.10120116127142964, -0.1605504162684674441 ) ) ;
#7595=CARTESIAN_POINT ( 'NONE',  ( -46.87302333144432254, 25.14943835890254675, -1.855287453902875416 ) ) ;
#7600=AXIS2_PLACEMENT_3D ( 'NONE', #25079, #38085, #27645 ) ;
#7603=VECTOR ( 'NONE', #28270, 1000.000000000000114 ) ;
#7605=ORIENTED_EDGE ( 'NONE', *, *, #39968, .F. ) ;
#7610=DIRECTION ( 'NONE',  ( -5.188838149069471174E-16, 1.699382548006136313E-16, 1.000000000000000000 ) ) ;
#7611=ORIENTED_EDGE ( 'NONE', *, *, #21370, .F. ) ;
#7615=CARTESIAN_POINT ( 'NONE',  ( -57.70126415073581683, 1.705439686540813238, -1.647193596428901285 ) ) ;
#7616=CARTESIAN_POINT ( 'NONE',  ( -46.60530155212502024, 26.17382724835479735, -8.515758108943001820E-15 ) ) ;
#7625=CARTESIAN_POINT ( 'NONE',  ( -45.05484530740381643, 21.03919035317155206, 3.644944174415911675 ) ) ;
#7627=EDGE_CURVE ( 'NONE', #8692, #25310, #20004, .T. ) ;
#7628=ORIENTED_EDGE ( 'NONE', *, *, #8361, .F. ) ;
#7632=AXIS2_PLACEMENT_3D ( 'NONE', #31582, #15166, #28595 ) ;
#7636=CARTESIAN_POINT ( 'NONE',  ( -24.49496359545907609, 76.94162913054094588, -1.524000000000005572 ) ) ;
#7639=CARTESIAN_POINT ( 'NONE',  ( -53.27040232883901183, 10.25240396212598348, 3.758512621827925226 ) ) ;
#7640=CARTESIAN_POINT ( 'NONE',  ( -47.59483747600737047, 24.73124547893296921, 0.7500189231788738642 ) ) ;
#7641=CARTESIAN_POINT ( 'NONE',  ( -49.66210360255988832, 16.76989353321783227, 4.946330335750482199 ) ) ;
#7642=CARTESIAN_POINT ( 'NONE',  ( -57.92211639876096996, 1.229603953560909124, 1.440092494702427617 ) ) ;
#7643=EDGE_CURVE ( 'NONE', #19349, #11005, #30893, .T. ) ;
#7647=CARTESIAN_POINT ( 'NONE',  ( -46.68395179480138779, 26.03198510454123848, 1.523999999999991140 ) ) ;
#7648=TOROIDAL_SURFACE ( 'NONE', #25996, 0.3809999999999997278, 0.2540000000000000036 ) ;
#7654=FILL_AREA_STYLE_COLOUR ( '', #1589 ) ;
#7655=EDGE_CURVE ( 'NONE', #4128, #40015, #16773, .T. ) ;
#7660=CARTESIAN_POINT ( 'NONE',  ( -46.39387867998472359, 20.78226312411871035, 4.747706454273270538 ) ) ;
#7670=AXIS2_PLACEMENT_3D ( 'NONE', #959, #26077, #39936 ) ;
#7673=CARTESIAN_POINT ( 'NONE',  ( -50.43530108972998960, 14.71354995532366594, 3.653486772774918734 ) ) ;
#7684=AXIS2_PLACEMENT_3D ( 'NONE', #1406, #40384, #24371 ) ;
#7689=DIRECTION ( 'NONE',  ( 5.188838149069472160E-16, -1.699382548006136559E-16, -1.000000000000000000 ) ) ;
#7690=EDGE_CURVE ( 'NONE', #16059, #702, #5027, .T. ) ;
#7693=DIRECTION ( 'NONE',  ( 5.188838149069472160E-16, -1.699382548006136559E-16, -1.000000000000000000 ) ) ;
#7694=TOROIDAL_SURFACE ( 'NONE', #25385, 0.7620000000000000107, 0.2540000000000000036 ) ;
#7696=CARTESIAN_POINT ( 'NONE',  ( -28.76494711669534610, 76.52965637509277030, -1.270000000000007567 ) ) ;
#7699=ORIENTED_EDGE ( 'NONE', *, *, #36327, .T. ) ;
#7708=DIRECTION ( 'NONE',  ( -0.8745520943968843053, 0.4849315768085461498, -4.268512490100407458E-16 ) ) ;
#7715=ORIENTED_EDGE ( 'NONE', *, *, #3453, .F. ) ;
#7720=VERTEX_POINT ( 'NONE', #13586 ) ;
#7721=DIRECTION ( 'NONE',  ( 5.188838149069471174E-16, -1.699382548006136313E-16, -1.000000000000000000 ) ) ;
#7724=CARTESIAN_POINT ( 'NONE',  ( -47.23734577298776571, 20.07943201422508395, 5.152903770775020931 ) ) ;
#7729=VECTOR ( 'NONE', #19966, 1000.000000000000114 ) ;
#7735=CARTESIAN_POINT ( 'NONE',  ( -57.69387532515970918, 1.166760082113277308, 1.211409762388486300 ) ) ;
#7742=DIRECTION ( 'NONE',  ( 5.188838149069472160E-16, -1.699382548006136559E-16, -1.000000000000000000 ) ) ;
#7743=ADVANCED_FACE ( 'NONE', ( #13793 ), #13996, .F. ) ;
#7744=CARTESIAN_POINT ( 'NONE',  ( -52.57757236033170045, 11.11936768914174145, -3.180765541460440105 ) ) ;
#7746=FACE_OUTER_BOUND ( 'NONE', #37834, .T. ) ;
#7747=CIRCLE ( 'NONE', #30838, 0.2540000000000000591 ) ;
#7750=CARTESIAN_POINT ( 'NONE',  ( -29.43804252120325415, 67.00854438735211716, -1.523999999998907784 ) ) ;
#7752=EDGE_CURVE ( 'NONE', #11776, #27053, #27493, .T. ) ;
#7754=FACE_OUTER_BOUND ( 'NONE', #6733, .T. ) ;
#7755=CARTESIAN_POINT ( 'NONE',  ( -58.03428750496623678, 2.144022121626051991, 0.09394692876219323807 ) ) ;
#7756=DIRECTION ( 'NONE',  ( -0.8572391118119481179, -0.5149185422762151410, 0.000000000000000000 ) ) ;
#7759=ORIENTED_EDGE ( 'NONE', *, *, #20338, .T. ) ;
#7760=CARTESIAN_POINT ( 'NONE',  ( -58.16317756775203662, 1.603007233358586081, -1.028822313162498947 ) ) ;
#7762=EDGE_LOOP ( 'NONE', ( #22981, #21952, #19465, #17069 ) ) ;
#7763=CARTESIAN_POINT ( 'NONE',  ( -47.35734194463830704, 19.95394279970460971, -5.176037500948948100 ) ) ;
#7772=CARTESIAN_POINT ( 'NONE',  ( -49.88865472065932494, 16.47292688720559539, -4.948449357369904433 ) ) ;
#7773=DIRECTION ( 'NONE',  ( -0.9454731675810332803, 0.3256999990547855828, -8.537024980200802097E-16 ) ) ;
#7777=CARTESIAN_POINT ( 'NONE',  ( -57.84388493117042174, 0.8425746053944089820, -1.050754030429361885 ) ) ;
#7780=AXIS2_PLACEMENT_3D ( 'NONE', #9542, #38321, #16127 ) ;
#7783=CARTESIAN_POINT ( 'NONE',  ( -48.04822308881582416, 19.89521662531995005, -5.294633059834412236 ) ) ;
#7787=EDGE_LOOP ( 'NONE', ( #37073, #12701, #228, #40316, #26252 ) ) ;
#7790=TOROIDAL_SURFACE ( 'NONE', #3019, 0.7620000000000000107, 0.2540000000000000036 ) ;
#7791=CARTESIAN_POINT ( 'NONE',  ( -15.96130909653717111, 80.00612572611477447, 1.269999999999997575 ) ) ;
#7793=CARTESIAN_POINT ( 'NONE',  ( -52.06546789126484498, 13.38259882428268632, -4.575081192416392106 ) ) ;
#7803=CARTESIAN_POINT ( 'NONE',  ( -57.51979792895002674, 1.380172231454854348, 0.6550001595469883142 ) ) ;
#7804=EDGE_CURVE ( 'NONE', #35632, #34680, #20796, .T. ) ;
#7807=CARTESIAN_POINT ( 'NONE',  ( -46.60530155212501313, 26.17382724835480445, -0.08466666666667589658 ) ) ;
#7809=LINE ( 'NONE', #40398, #17604 ) ;
#7817=EDGE_LOOP ( 'NONE', ( #17794, #40352, #13993, #5202 ) ) ;
#7821=LINE ( 'NONE', #27192, #6111 ) ;
#7822=ORIENTED_EDGE ( 'NONE', *, *, #35344, .F. ) ;
#7826=CARTESIAN_POINT ( 'NONE',  ( -58.62613161865938594, -0.2841797903866821740, -0.3870556671703427321 ) ) ;
#7833=DIRECTION ( 'NONE',  ( 0.8745520943968235761, -0.4849315768086558398, 4.268512490100410909E-16 ) ) ;
#7835=ORIENTED_EDGE ( 'NONE', *, *, #9252, .F. ) ;
#7839=CARTESIAN_POINT ( 'NONE',  ( -10.15441061790785682, 81.86333342972157823, -1.523999999999999133 ) ) ;
#7843=CARTESIAN_POINT ( 'NONE',  ( -6.559134203278482289, 78.24119908707510263, -1.523999999999996469 ) ) ;
#7844=EDGE_CURVE ( 'NONE', #6518, #16326, #28820, .T. ) ;
#7845=VECTOR ( 'NONE', #10626, 1000.000000000000000 ) ;
#7848=CARTESIAN_POINT ( 'NONE',  ( -57.35194221082588939, 1.902352115738135119, 1.527398156819058661 ) ) ;
#7849=LINE ( 'NONE', #34045, #15996 ) ;
#7850=CARTESIAN_POINT ( 'NONE',  ( -57.64973313486724038, 1.352533784701764885, 1.499908592384902706 ) ) ;
#7851=CARTESIAN_POINT ( 'NONE',  ( -57.63560179895036129, 1.846074579945612637, 1.702420071201910412 ) ) ;
#7852=ADVANCED_FACE ( 'NONE', ( #8665 ), #31511, .T. ) ;
#7856=CARTESIAN_POINT ( 'NONE',  ( -46.40591231939538375, 23.70796668624020853, 2.618124260499386402 ) ) ;
#7863=ORIENTED_EDGE ( 'NONE', *, *, #13113, .T. ) ;
#7866=ADVANCED_FACE ( 'NONE', ( #27619 ), #4859, .F. ) ;
#7868=CARTESIAN_POINT ( 'NONE',  ( -44.75127360237820540, 21.22985803517970638, 3.557274316435921513 ) ) ;
#7869=DIRECTION ( 'NONE',  ( 5.188838149069472160E-16, -1.699382548006136559E-16, -1.000000000000000000 ) ) ;
#7880=CARTESIAN_POINT ( 'NONE',  ( -50.67046617086457161, 13.01238886216411039, 1.492009926703871336 ) ) ;
#7882=CIRCLE ( 'NONE', #30989, 0.2540000000000010583 ) ;
#7886=ORIENTED_EDGE ( 'NONE', *, *, #31245, .F. ) ;
#7895=CARTESIAN_POINT ( 'NONE',  ( -8.723850037987370243, 68.58388863026053173, 1.524000000000003352 ) ) ;
#7899=CARTESIAN_POINT ( 'NONE',  ( -17.08598887363762131, 83.79821757228496892, -1.524000000000002908 ) ) ;
#7904=ORIENTED_EDGE ( 'NONE', *, *, #40026, .F. ) ;
#7912=CARTESIAN_POINT ( 'NONE',  ( -20.59944062528794362, 79.83666051618703818, -1.524000000000004018 ) ) ;
#7933=AXIS2_PLACEMENT_3D ( 'NONE', #35526, #21873, #28495 ) ;
#7936=AXIS2_PLACEMENT_3D ( 'NONE', #38854, #6070, #100 ) ;
#7941=EDGE_CURVE ( 'NONE', #15033, #26127, #14615, .T. ) ;
#7942=CARTESIAN_POINT ( 'NONE',  ( -48.15691857872906922, 19.01861963076551021, 5.213839621080547992 ) ) ;
#7950=CARTESIAN_POINT ( 'NONE',  ( -57.71946847630993460, 1.146847591362354368, -1.351507486235954403 ) ) ;
#7954=DIRECTION ( 'NONE',  ( 0.1906721105965186736, -0.9816537812491066273, 0.000000000000000000 ) ) ;
#7960=CARTESIAN_POINT ( 'NONE',  ( -58.20820809768405013, 1.420579653404072218, 1.355822160094593887 ) ) ;
#7964=ORIENTED_EDGE ( 'NONE', *, *, #10499, .T. ) ;
#7965=CARTESIAN_POINT ( 'NONE',  ( -55.64884842185075087, 8.819639511685364752, -1.021878145082219635 ) ) ;
#7967=CARTESIAN_POINT ( 'NONE',  ( -45.96492958221768532, 21.02066589182467382, -4.445716362542115441 ) ) ;
#7972=CARTESIAN_POINT ( 'NONE',  ( -29.20503723471917823, 64.36951892211030213, 1.269999999999993356 ) ) ;
#7974=EDGE_CURVE ( 'NONE', #2461, #537, #5700, .T. ) ;
#7975=CARTESIAN_POINT ( 'NONE',  ( -49.99298857535946894, 16.30720399940068788, -4.926441425282844122 ) ) ;
#7979=CARTESIAN_POINT ( 'NONE',  ( -49.99139319293801975, 16.20859854215753515, -4.826775924100495274 ) ) ;
#7982=CARTESIAN_POINT ( 'NONE',  ( -48.65005484009959957, 18.46594748123760965, -5.297328305960443018 ) ) ;
#7983=CIRCLE ( 'NONE', #35195, 0.2540000000000000036 ) ;
#7990=FACE_OUTER_BOUND ( 'NONE', #19499, .T. ) ;
#7993=CARTESIAN_POINT ( 'NONE',  ( -55.60486134785667645, 7.243031971518515633, -3.140198620020504094 ) ) ;
#7994=CIRCLE ( 'NONE', #31797, 0.6350000000000014522 ) ;
#8003=AXIS2_PLACEMENT_3D ( 'NONE', #17963, #4014, #35955 ) ;
#8004=CARTESIAN_POINT ( 'NONE',  ( -58.35029634831491308, -0.2563984898762833309, 0.1830726351724760170 ) ) ;
#8006=ORIENTED_EDGE ( 'NONE', *, *, #2504, .T. ) ;
#8007=CARTESIAN_POINT ( 'NONE',  ( -47.62967605938791849, 25.45029596856965171, -9.729597958152646858E-15 ) ) ;
#8010=ORIENTED_EDGE ( 'NONE', *, *, #35498, .T. ) ;
#8011=DIRECTION ( 'NONE',  ( -0.8745520943968249084, 0.4849315768086533418, -5.271987356194193006E-16 ) ) ;
#8018=ORIENTED_EDGE ( 'NONE', *, *, #15372, .T. ) ;
#8028=CARTESIAN_POINT ( 'NONE',  ( -56.42349525705788693, 3.945591430473524230, -2.427201670071943429 ) ) ;
#8038=EDGE_LOOP ( 'NONE', ( #21208, #34655, #29672, #34261 ) ) ;
#8040=DIRECTION ( 'NONE',  ( 5.188838149069472160E-16, -1.699382548006136559E-16, -1.000000000000000000 ) ) ;
#8041=CARTESIAN_POINT ( 'NONE',  ( -20.37123700195715870, 79.57406833244878896, -1.524000000000003796 ) ) ;
#8048=CARTESIAN_POINT ( 'NONE',  ( -55.27300860040548258, 6.262530169634048072, 2.859796270508659255 ) ) ;
#8050=CARTESIAN_POINT ( 'NONE',  ( -58.83227707057486811, -0.08366279997995551554, 0.2458995907044889129 ) ) ;
#8051=CARTESIAN_POINT ( 'NONE',  ( -58.63368340525728684, -0.2968340078074506727, 0.3659978923735402456 ) ) ;
#8052=LINE ( 'NONE', #28053, #30693 ) ;
#8056=CARTESIAN_POINT ( 'NONE',  ( -53.83456308493991571, 9.379524109395250164, 3.755176697756422044 ) ) ;
#8062=ORIENTED_EDGE ( 'NONE', *, *, #41616, .F. ) ;
#8066=CARTESIAN_POINT ( 'NONE',  ( -43.98070909377825899, 21.30087824702203037, 2.736222515986834747 ) ) ;
#8067=DIRECTION ( 'NONE',  ( -0.8745520943968235761, 0.4849315768086558953, -5.361993529360570985E-16 ) ) ;
#8069=AXIS2_PLACEMENT_3D ( 'NONE', #10510, #17317, #20921 ) ;
#8072=DIRECTION ( 'NONE',  ( -0.9816537812491077375, -0.1906721105965138996, -4.769617732184456426E-16 ) ) ;
#8080=EDGE_LOOP ( 'NONE', ( #15022, #41657, #10257, #2611 ) ) ;
#8081=CARTESIAN_POINT ( 'NONE',  ( -52.67395729902614221, 10.59333423579336753, 2.513629069394781368 ) ) ;
#8088=DIRECTION ( 'NONE',  ( -5.188838149069471174E-16, 1.699382548006136313E-16, 1.000000000000000000 ) ) ;
#8091=ORIENTED_EDGE ( 'NONE', *, *, #38040, .F. ) ;
#8095=DIRECTION ( 'NONE',  ( -5.188838149069471174E-16, 1.699382548006136313E-16, 1.000000000000000000 ) ) ;
#8103=EDGE_LOOP ( 'NONE', ( #30874, #33955, #14459, #18374 ) ) ;
#8114=EDGE_CURVE ( 'NONE', #2780, #27477, #5479, .T. ) ;
#8118=ORIENTED_EDGE ( 'NONE', *, *, #12274, .T. ) ;
#8124=ORIENTED_EDGE ( 'NONE', *, *, #37081, .F. ) ;
#8125=FACE_OUTER_BOUND ( 'NONE', #3961, .T. ) ;
#8129=AXIS2_PLACEMENT_3D ( 'NONE', #12932, #41923, #390 ) ;
#8135=EDGE_CURVE ( 'NONE', #9063, #19512, #11119, .T. ) ;
#8142=CARTESIAN_POINT ( 'NONE',  ( -56.62423581747135160, 3.520748359633372182, 2.300294558594641714 ) ) ;
#8143=ADVANCED_FACE ( 'NONE', ( #17607 ), #34940, .T. ) ;
#8150=CARTESIAN_POINT ( 'NONE',  ( -46.95911617132934879, 24.98948415085533270, 1.986615011824473864 ) ) ;
#8151=CIRCLE ( 'NONE', #4081, 8.794749999999993406 ) ;
#8153=CARTESIAN_POINT ( 'NONE',  ( -58.02159823468433331, 0.4660483771539991604, -0.8824573672536869529 ) ) ;
#8156=CARTESIAN_POINT ( 'NONE',  ( -31.59722765895411101, 71.22255575826451945, -1.270000000000008233 ) ) ;
#8158=DIRECTION ( 'NONE',  ( 5.188838149069472160E-16, -1.699382548006136559E-16, -1.000000000000000000 ) ) ;
#8160=CARTESIAN_POINT ( 'NONE',  ( -46.59067040677711447, 25.67275826535883709, 1.583530073016286899 ) ) ;
#8161=DIRECTION ( 'NONE',  ( -0.8745520943968240202, 0.4849315768086551737, -5.361993529360572958E-16 ) ) ;
#8166=ORIENTED_EDGE ( 'NONE', *, *, #34061, .T. ) ;
#8167=CYLINDRICAL_SURFACE ( 'NONE', #1882, 0.2539999999999986158 ) ;
#8169=EDGE_LOOP ( 'NONE', ( #23862, #23704, #7339, #19890 ) ) ;
#8170=CARTESIAN_POINT ( 'NONE',  ( -46.78477525497644507, 20.40172935491330719, -4.969468548368532801 ) ) ;
#8178=CARTESIAN_POINT ( 'NONE',  ( -49.52577634351906966, 17.04162928648567288, -5.022404464390935352 ) ) ;
#8180=CYLINDRICAL_SURFACE ( 'NONE', #27485, 0.6350000000000014522 ) ;
#8182=CARTESIAN_POINT ( 'NONE',  ( -56.47502814425232742, 3.765754792631150760, -2.169991423106563566 ) ) ;
#8185=CARTESIAN_POINT ( 'NONE',  ( -41.88683177698051452, 22.33947639032530219, -1.656270940288501636 ) ) ;
#8191=CARTESIAN_POINT ( 'NONE',  ( -58.37934292759150168, 0.9822739792931106662, -1.208960021102219340 ) ) ;
#8199=EDGE_CURVE ( 'NONE', #11267, #1003, #40388, .T. ) ;
#8200=CARTESIAN_POINT ( 'NONE',  ( -41.40170217118274110, 22.71997040916441080, -0.2118088196526931866 ) ) ;
#8202=CIRCLE ( 'NONE', #34074, 0.2540000000000010583 ) ;
#8203=CARTESIAN_POINT ( 'NONE',  ( -8.539387426415398608, 74.43734692935288422, -1.269999999999996909 ) ) ;
#8204=CARTESIAN_POINT ( 'NONE',  ( -58.37241122568488549, -0.2962816677227891882, -1.032426590602281809E-14 ) ) ;
#8205=CARTESIAN_POINT ( 'NONE',  ( -53.84631020977099780, 15.55534180641097386, 0.3033304672099269017 ) ) ;
#8208=CARTESIAN_POINT ( 'NONE',  ( -47.91671457320775573, 24.98613645765719582, -0.3547230740385284853 ) ) ;
#8219=DIRECTION ( 'NONE',  ( -0.8745520943968240202, 0.4849315768086553402, -5.361993529360572958E-16 ) ) ;
#8223=ORIENTED_EDGE ( 'NONE', *, *, #15865, .T. ) ;
#8228=LINE ( 'NONE', #5262, #35447 ) ;
#8230=CARTESIAN_POINT ( 'NONE',  ( -58.47668496617176004, -0.4796687618251362917, -0.2989310191338567235 ) ) ;
#8244=DIRECTION ( 'NONE',  ( -5.188838149069472160E-16, 1.699382548006136559E-16, 1.000000000000000000 ) ) ;
#8251=CARTESIAN_POINT ( 'NONE',  ( -17.64290547347870941, 83.78857423953914463, 1.523999999999996247 ) ) ;
#8252=CARTESIAN_POINT ( 'NONE',  ( -58.36745437842773754, -0.2866796535172885796, 0.05885235802170251523 ) ) ;
#8253=CARTESIAN_POINT ( 'NONE',  ( -30.60466991270287807, 55.37784481733978481, -1.524000000000004462 ) ) ;
#8254=AXIS2_PLACEMENT_3D ( 'NONE', #33501, #7514, #20264 ) ;
#8255=CARTESIAN_POINT ( 'NONE',  ( -55.83113473690871587, 5.632394305663344092, 2.901290885506219386 ) ) ;
#8260=CARTESIAN_POINT ( 'NONE',  ( -53.68435271313694557, 11.12367579685427721, 3.945100831076007619 ) ) ;
#8263=CYLINDRICAL_SURFACE ( 'NONE', #11489, 0.5080000000000000071 ) ;
#8273=CARTESIAN_POINT ( 'NONE',  ( -6.422645615570758970, 77.88548590848095898, -1.523999999999996469 ) ) ;
#8275=DIRECTION ( 'NONE',  ( -0.8745520943968249084, 0.4849315768086536194, -5.575199987069925217E-16 ) ) ;
#8277=CARTESIAN_POINT ( 'NONE',  ( -5.861642722916909243, 64.54502714855203749, -1.523999999999993804 ) ) ;
#8283=TOROIDAL_SURFACE ( 'NONE', #11680, 0.3810000000000014486, 0.2540000000000000036 ) ;
#8288=CARTESIAN_POINT ( 'NONE',  ( -48.25086062633821626, 17.91646674446130305, 3.976701633436060757 ) ) ;
#8303=DIRECTION ( 'NONE',  ( 0.8745520943968235761, -0.4849315768086558398, 0.000000000000000000 ) ) ;
#8306=DIRECTION ( 'NONE',  ( -0.8745520943968235761, 0.4849315768086558953, -5.361993529360570985E-16 ) ) ;
#8312=CARTESIAN_POINT ( 'NONE',  ( -23.97640303682767993, 76.49434496853974963, -1.270000000000005347 ) ) ;
#8315=B_SPLINE_CURVE_WITH_KNOTS ( 'NONE', 3,
 ( #19356, #9165, #2785, #12560 ),
 .UNSPECIFIED., .F., .F.,
 ( 4, 4 ),
 ( 0.000000000000000000, 0.9566564897266378598 ),
 .UNSPECIFIED. ) ;
#8319=AXIS2_PLACEMENT_3D ( 'NONE', #18104, #38141, #15746 ) ;
#8321=CARTESIAN_POINT ( 'NONE',  ( -48.56815661899839398, 19.24492339269599839, 5.224590812749970503 ) ) ;
#8325=EDGE_CURVE ( 'NONE', #31622, #24097, #15185, .T. ) ;
#8329=ORIENTED_EDGE ( 'NONE', *, *, #34821, .F. ) ;
#8341=CARTESIAN_POINT ( 'NONE',  ( -42.82337740149211669, 22.05454911558773645, 2.000910913296384930 ) ) ;
#8345=DIRECTION ( 'NONE',  ( -5.188838149069471174E-16, 1.699382548006136313E-16, 1.000000000000000000 ) ) ;
#8353=CARTESIAN_POINT ( 'NONE',  ( -57.94306413390888366, 1.184802614102420382, 1.419326152558788134 ) ) ;
#8358=CIRCLE ( 'NONE', #11094, 0.6350000000000014522 ) ;
#8361=EDGE_CURVE ( 'NONE', #2275, #13951, #19496, .T. ) ;
#8363=CARTESIAN_POINT ( 'NONE',  ( -57.78284603921808582, 0.8603191986865516006, -0.5272538806337706552 ) ) ;
#8365=CARTESIAN_POINT ( 'NONE',  ( -10.34239276132902319, 65.15305678602257444, -1.269999999999996243 ) ) ;
#8368=CARTESIAN_POINT ( 'NONE',  ( -17.08598887363762131, 83.79821757228496892, -1.270000000000002904 ) ) ;
#8376=ORIENTED_EDGE ( 'NONE', *, *, #17204, .F. ) ;
#8378=ORIENTED_EDGE ( 'NONE', *, *, #37282, .F. ) ;
#8379=CARTESIAN_POINT ( 'NONE',  ( -47.84756666395252722, 19.38928433903621240, -5.209054514891962917 ) ) ;
#8380=CIRCLE ( 'NONE', #18583, 0.2539999999999986158 ) ;
#8384=AXIS2_PLACEMENT_3D ( 'NONE', #36428, #10209, #38984 ) ;
#8388=CARTESIAN_POINT ( 'NONE',  ( -48.68735867619428603, 18.29031291928623659, -5.164865279787345997 ) ) ;
#8390=ORIENTED_EDGE ( 'NONE', *, *, #31314, .T. ) ;
#8394=CARTESIAN_POINT ( 'NONE',  ( -52.83837246138028831, 11.08843963240696517, -3.928308309794706688 ) ) ;
#8397=CARTESIAN_POINT ( 'NONE',  ( -56.22331024217277928, 5.808995339285999648, -2.850545730341259798 ) ) ;
#8400=EDGE_CURVE ( 'NONE', #19740, #9063, #8151, .T. ) ;
#8401=ORIENTED_EDGE ( 'NONE', *, *, #34821, .T. ) ;
#8405=EDGE_CURVE ( 'NONE', #1192, #30178, #11546, .T. ) ;
#8406=CARTESIAN_POINT ( 'NONE',  ( -58.07447437077728125, 1.735896131820596766, -1.499107834811110429 ) ) ;
#8409=CARTESIAN_POINT ( 'NONE',  ( -17.14500000000466784, 71.11999999999886768, -1.524000000000000909 ) ) ;
#8414=DIRECTION ( 'NONE',  ( -0.1906721105965055174, 0.9816537812491091808, 0.000000000000000000 ) ) ;
#8416=CARTESIAN_POINT ( 'NONE',  ( -44.35420297070785978, 19.68308750433651966, -0.4327882352162440438 ) ) ;
#8419=TOROIDAL_SURFACE ( 'NONE', #37018, 0.7620000000000000107, 0.2540000000000000036 ) ;
#8420=CARTESIAN_POINT ( 'NONE',  ( -57.78284603921808582, 0.8603191986865516006, 0.5272538806337502271 ) ) ;
#8421=CARTESIAN_POINT ( 'NONE',  ( -49.23607562092252721, 19.66429951101446960, 3.974467759520285082 ) ) ;
#8423=EDGE_LOOP ( 'NONE', ( #2573, #33924, #21553, #29564 ) ) ;
#8424=CARTESIAN_POINT ( 'NONE',  ( -48.74997074597248314, 21.16799237019927205, -3.036721307642072265 ) ) ;
#8427=CIRCLE ( 'NONE', #2339, 0.2540000000000018909 ) ;
#8439=CARTESIAN_POINT ( 'NONE',  ( -41.05189575270519242, 23.09451173561982529, -1.269999999999997797 ) ) ;
#8440=DIRECTION ( 'NONE',  ( -5.188838149069472160E-16, 1.699382548006136559E-16, 1.000000000000000000 ) ) ;
#8441=VERTEX_POINT ( 'NONE', #26952 ) ;
#8445=CARTESIAN_POINT ( 'NONE',  ( -47.84356795211455449, 19.38525671449502852, -5.197506975155119058 ) ) ;
#8447=AXIS2_PLACEMENT_3D ( 'NONE', #34224, #11839, #38259 ) ;
#8457=EDGE_CURVE ( 'NONE', #18705, #21597, #23768, .T. ) ;
#8458=DIRECTION ( 'NONE',  ( -5.188838149069472160E-16, 1.699382548006136559E-16, 1.000000000000000000 ) ) ;
#8459=CIRCLE ( 'NONE', #15918, 0.6349999999999977884 ) ;
#8461=VERTEX_POINT ( 'NONE', #775 ) ;
#8463=CARTESIAN_POINT ( 'NONE',  ( -6.318938770521977055, 64.36956080246774548, -1.269999999999994023 ) ) ;
#8466=B_SPLINE_CURVE_WITH_KNOTS ( 'NONE', 3,
 ( #14956, #35006, #6033, #21758 ),
 .UNSPECIFIED., .F., .F.,
 ( 4, 4 ),
 ( 9.335326988569945976E-17, 6.355780391037319497E-05 ),
 .UNSPECIFIED. ) ;
#8468=ADVANCED_FACE ( 'NONE', ( #36135 ), #18325, .T. ) ;
#8473=LINE ( 'NONE', #24637, #26739 ) ;
#8474=CARTESIAN_POINT ( 'NONE',  ( -58.34697146883529228, -0.2437238978784766197, 0.1881573647123204462 ) ) ;
#8476=CARTESIAN_POINT ( 'NONE',  ( -28.65049350906917880, 77.81814547195517662, -1.524000000000008015 ) ) ;
#8479=ORIENTED_EDGE ( 'NONE', *, *, #38421, .T. ) ;
#8480=CARTESIAN_POINT ( 'NONE',  ( -49.19743978460682143, 17.65503563884207594, 5.190924102448284394 ) ) ;
#8489=DIRECTION ( 'NONE',  ( 5.188838149069472160E-16, -1.699382548006136559E-16, -1.000000000000000000 ) ) ;
#8490=CARTESIAN_POINT ( 'NONE',  ( -41.63373767251881929, 22.51256436878201939, 1.325597493787631587 ) ) ;
#8495=CYLINDRICAL_SURFACE ( 'NONE', #25200, 0.2539999999999986158 ) ;
#8502=VERTEX_POINT ( 'NONE', #32723 ) ;
#8503=CARTESIAN_POINT ( 'NONE',  ( -56.39145920764457287, 3.696195836928164891, 1.449839391286695589 ) ) ;
#8525=B_SPLINE_SURFACE_WITH_KNOTS ( 'NONE', 3, 1, ( 
 ( #29478, #29262 ),
 ( #4143, #6908 ),
 ( #32466, #13287 ),
 ( #19878, #13916 ),
 ( #23061, #32892 ) ),
 .UNSPECIFIED., .F., .F., .F.,
 ( 4, 1, 4 ),
 ( 2, 2 ),
 ( 0.000000000000000000, 0.4760613254002281081, 0.9521226508004562161 ),
 ( 0.000000000000000000, 1.000000000000000000 ),
 .UNSPECIFIED. ) ;
#8526=EDGE_LOOP ( 'NONE', ( #40626, #25995, #152, #26633 ) ) ;
#8527=ORIENTED_EDGE ( 'NONE', *, *, #13418, .T. ) ;
#8528=CARTESIAN_POINT ( 'NONE',  ( -5.369399562154598904, 64.90898011766716991, -1.269999999999993578 ) ) ;
#8535=CARTESIAN_POINT ( 'NONE',  ( -57.80205714066466527, 2.371715784325115095, 1.753227392946289154 ) ) ;
#8553=DIRECTION ( 'NONE',  ( 0.9336303900108928744, 0.3582377630123714241, 0.000000000000000000 ) ) ;
#8561=DIRECTION ( 'NONE',  ( 6.104810211199659290E-14, 1.534542364845396606E-13, 1.000000000000000000 ) ) ;
#8564=ORIENTED_EDGE ( 'NONE', *, *, #37299, .F. ) ;
#8566=DIRECTION ( 'NONE',  ( 0.4849315768086534528, 0.8745520943968249084, 1.030032898892974818E-16 ) ) ;
#8567=CARTESIAN_POINT ( 'NONE',  ( -57.60629982073535871, 1.412843483088787044, 1.546595473637959239 ) ) ;
#8568=CIRCLE ( 'NONE', #32370, 0.5080000000000000071 ) ;
#8576=CARTESIAN_POINT ( 'NONE',  ( -56.88731995051697510, 2.378615435641926013, -1.029510524999914353E-14 ) ) ;
#8579=PLANE ( 'NONE',  #24623 ) ;
#8580=CARTESIAN_POINT ( 'NONE',  ( -10.55305098051677248, 77.31887769575739355, -1.523999999999998467 ) ) ;
#8588=CARTESIAN_POINT ( 'NONE',  ( -58.33482727260580702, 1.278009831241974759, -1.053392386569325874E-14 ) ) ;
#8596=CIRCLE ( 'NONE', #7933, 0.2539999999999990599 ) ;
#8598=CARTESIAN_POINT ( 'NONE',  ( -51.53167472531687565, 13.74790139509799936, -4.551524594881854568 ) ) ;
#8599=AXIS2_PLACEMENT_3D ( 'NONE', #41224, #2676, #35459 ) ;
#8601=CARTESIAN_POINT ( 'NONE',  ( -38.65395868481546415, 29.38327706004843876, -1.524000000000004906 ) ) ;
#8603=CIRCLE ( 'NONE', #32404, 0.6350000000000014522 ) ;
#8604=CARTESIAN_POINT ( 'NONE',  ( -56.22633580991770685, 4.287755688858543301, -2.325607019181227475 ) ) ;
#8607=CARTESIAN_POINT ( 'NONE',  ( -50.15972161391664486, 17.13814111569220699, -4.955022299345085202 ) ) ;
#8613=EDGE_CURVE ( 'NONE', #38737, #41570, #14919, .T. ) ;
#8614=EDGE_CURVE ( 'NONE', #41032, #28056, #9727, .T. ) ;
#8615=CARTESIAN_POINT ( 'NONE',  ( -58.40597088826705630, 0.2738206778524349128, -0.9753506901443967925 ) ) ;
#8621=DIRECTION ( 'NONE',  ( -0.9816537812491094028, -0.1906721105965052399, 6.949828216605158287E-15 ) ) ;
#8627=CARTESIAN_POINT ( 'NONE',  ( -50.94572941386617515, 18.90544291192138004, 2.223209376321575004 ) ) ;
#8630=ORIENTED_EDGE ( 'NONE', *, *, #28953, .F. ) ;
#8631=CARTESIAN_POINT ( 'NONE',  ( -50.95401363114979176, 21.69085172357045010, -1.082912443856812391E-14 ) ) ;
#8635=CARTESIAN_POINT ( 'NONE',  ( -47.84356795211458291, 19.38525671449504983, 5.197506975155153697 ) ) ;
#8639=CIRCLE ( 'NONE', #36541, 0.2539999999999931202 ) ;
#8646=ADVANCED_FACE ( 'NONE', ( #3977 ), #3385, .T. ) ;
#8648=CARTESIAN_POINT ( 'NONE',  ( -41.08173151913536003, 23.06272320883578075, -1.524000000017811773 ) ) ;
#8661=AXIS2_PLACEMENT_3D ( 'NONE', #36672, #17275, #33691 ) ;
#8665=FACE_OUTER_BOUND ( 'NONE', #7137, .T. ) ;
#8667=ORIENTED_EDGE ( 'NONE', *, *, #1928, .F. ) ;
#8671=CIRCLE ( 'NONE', #18874, 0.3810000000000015041 ) ;
#8678=DIRECTION ( 'NONE',  ( 0.8745520943968235761, -0.4849315768086558398, 0.000000000000000000 ) ) ;
#8679=CARTESIAN_POINT ( 'NONE',  ( -58.28980089130899245, -0.1221305639422176070, 0.3636100989710047693 ) ) ;
#8683=CIRCLE ( 'NONE', #23532, 0.5079999999999968985 ) ;
#8684=ORIENTED_EDGE ( 'NONE', *, *, #28211, .F. ) ;
#8686=CARTESIAN_POINT ( 'NONE',  ( -51.09990735641632398, 14.52648110433587370, 4.713018929684107405 ) ) ;
#8690=DIRECTION ( 'NONE',  ( -0.6559537821943236535, 0.7548010569845287066, 2.445308717870848367E-15 ) ) ;
#8692=VERTEX_POINT ( 'NONE', #4402 ) ;
#8694=CARTESIAN_POINT ( 'NONE',  ( -33.42971872652991294, 49.93539301574497813, 1.523999999999990917 ) ) ;
#8696=CARTESIAN_POINT ( 'NONE',  ( -42.61647787783788743, 21.91010357080768856, 1.992259954793912158 ) ) ;
#8709=EDGE_CURVE ( 'NONE', #30779, #6194, #35926, .T. ) ;
#8711=ORIENTED_EDGE ( 'NONE', *, *, #5335, .T. ) ;
#8712=CARTESIAN_POINT ( 'NONE',  ( -55.14069116334859189, 5.401725095812784261, -9.468868952413029037E-15 ) ) ;
#8716=ORIENTED_EDGE ( 'NONE', *, *, #25566, .T. ) ;
#8730=CARTESIAN_POINT ( 'NONE',  ( -4.095482865093060809, 71.62450171983788039, 1.524000000000005350 ) ) ;
#8743=DIRECTION ( 'NONE',  ( 0.8745520943968249084, -0.4849315768086533418, 5.271987356194193006E-16 ) ) ;
#8745=DIRECTION ( 'NONE',  ( -0.8745520943968243532, 0.4849315768086547296, -5.361993529360573944E-16 ) ) ;
#8763=EDGE_CURVE ( 'NONE', #35910, #14467, #2024, .T. ) ;
#8774=CARTESIAN_POINT ( 'NONE',  ( -18.01920641645601151, 83.84822824455466161, 1.269999999999995799 ) ) ;
#8780=FACE_OUTER_BOUND ( 'NONE', #37266, .T. ) ;
#8781=AXIS2_PLACEMENT_3D ( 'NONE', #15840, #25230, #38654 ) ;
#8784=CARTESIAN_POINT ( 'NONE',  ( -56.60409974985236659, 4.028981045520047211, 2.444348447023971804 ) ) ;
#8792=CARTESIAN_POINT ( 'NONE',  ( -57.22211421646275653, 1.778355698664441098, -1.009576694067165286E-14 ) ) ;
#8799=DIRECTION ( 'NONE',  ( -0.8745520943968243532, 0.4849315768086547296, -5.361993529360573944E-16 ) ) ;
#8804=CIRCLE ( 'NONE', #37349, 0.6350000000000014522 ) ;
#8805=AXIS2_PLACEMENT_3D ( 'NONE', #41342, #25348, #28544 ) ;
#8807=CARTESIAN_POINT ( 'NONE',  ( -41.52577271625990818, 22.97115911878781702, -1.524000000000015564 ) ) ;
#8814=CARTESIAN_POINT ( 'NONE',  ( -56.33726422335487172, 4.582392934301856791, -2.601884677528782497 ) ) ;
#8815=EDGE_LOOP ( 'NONE', ( #17494, #40207, #15298, #31342 ) ) ;
#8817=LINE ( 'NONE', #28612, #15472 ) ;
#8819=CARTESIAN_POINT ( 'NONE',  ( -48.37723337351298625, 18.71554189175216010, -5.186504670261411043 ) ) ;
#8822=CARTESIAN_POINT ( 'NONE',  ( -56.21344593158320180, 5.939860726778031896, -2.828251681716873911 ) ) ;
#8824=ORIENTED_EDGE ( 'NONE', *, *, #5103, .F. ) ;
#8828=CARTESIAN_POINT ( 'NONE',  ( -58.83227707057486811, -0.08366279997995551554, -0.2458995907045101459 ) ) ;
#8829=CIRCLE ( 'NONE', #16297, 0.2539999999999992819 ) ;
#8835=CARTESIAN_POINT ( 'NONE',  ( -57.24023649071029496, 3.661034843983918208, -2.195083147259570211 ) ) ;
#8836=LINE ( 'NONE', #30982, #35612 ) ;
#8837=ORIENTED_EDGE ( 'NONE', *, *, #5633, .T. ) ;
#8839=CARTESIAN_POINT ( 'NONE',  ( -57.83637253161431602, 2.237724655402451024, 1.757929103219288747 ) ) ;
#8842=CARTESIAN_POINT ( 'NONE',  ( -49.72500615219620101, 20.62299186128851858, 2.281585690523495025 ) ) ;
#8845=CARTESIAN_POINT ( 'NONE',  ( -48.56815661899839398, 19.24492339269599839, -5.224590812749988267 ) ) ;
#8859=CARTESIAN_POINT ( 'NONE',  ( -23.91048590848665967, 81.84235438443283783, 1.269999999999992912 ) ) ;
#8861=FACE_OUTER_BOUND ( 'NONE', #30503, .T. ) ;
#8874=CARTESIAN_POINT ( 'NONE',  ( -10.57002714855771508, 82.40335727708655611, -1.269999999999999130 ) ) ;
#8875=AXIS2_PLACEMENT_3D ( 'NONE', #4745, #1753, #8553 ) ;
#8876=CARTESIAN_POINT ( 'NONE',  ( -45.67973391888839529, 25.66060799623228661, -1.524000000000008237 ) ) ;
#8879=DIRECTION ( 'NONE',  ( -5.188838149069472160E-16, 1.699382548006136559E-16, 1.000000000000000000 ) ) ;
#8887=CARTESIAN_POINT ( 'NONE',  ( -58.05778227315403228, 0.3792031317013907499, 0.7797940327017545137 ) ) ;
#8890=FACE_OUTER_BOUND ( 'NONE', #13042, .T. ) ;
#8891=DIRECTION ( 'NONE',  ( 5.188838149069472160E-16, -1.699382548006136559E-16, -1.000000000000000000 ) ) ;
#8892=DIRECTION ( 'NONE',  ( 5.188838149069472160E-16, -1.699382548006136559E-16, -1.000000000000000000 ) ) ;
#8894=CARTESIAN_POINT ( 'NONE',  ( -48.16508968810062896, 19.01313136326716347, 5.219744232931976313 ) ) ;
#8898=DIRECTION ( 'NONE',  ( 0.7548010569845180484, 0.6559537821943359770, 0.000000000000000000 ) ) ;
#8899=CIRCLE ( 'NONE', #1443, 8.794749999999996959 ) ;
#8905=DIRECTION ( 'NONE',  ( 0.8745520943968240202, -0.4849315768086553402, 6.829619984160650158E-16 ) ) ;
#8907=DIRECTION ( 'NONE',  ( -0.8745520943968245753, 0.4849315768086539524, -5.691349986800526185E-16 ) ) ;
#8911=DIRECTION ( 'NONE',  ( -0.8745520943968361216, 0.4849315768086333023, -6.829619984160648185E-16 ) ) ;
#8918=ORIENTED_EDGE ( 'NONE', *, *, #1409, .T. ) ;
#8919=EDGE_CURVE ( 'NONE', #1690, #24097, #8829, .T. ) ;
#8920=CARTESIAN_POINT ( 'NONE',  ( -55.00324375927522169, 6.200002331679180578, 1.420877854375688587 ) ) ;
#8928=ORIENTED_EDGE ( 'NONE', *, *, #27889, .F. ) ;
#8931=DIRECTION ( 'NONE',  ( -0.8745520943968240202, 0.4849315768086553402, -5.361993529360572958E-16 ) ) ;
#8935=ADVANCED_FACE ( 'NONE', ( #8780 ), #28367, .T. ) ;
#8938=CARTESIAN_POINT ( 'NONE',  ( -46.94614764229907422, 25.08748753966319001, 1.921268435158901999 ) ) ;
#8939=CARTESIAN_POINT ( 'NONE',  ( -46.81215924274956564, 25.79096025118141711, 0.6894041771338947910 ) ) ;
#8942=CARTESIAN_POINT ( 'NONE',  ( -46.91604881613255174, 25.30076613767161220, 1.786867259277511666 ) ) ;
#8945=VERTEX_POINT ( 'NONE', #25381 ) ;
#8950=AXIS2_PLACEMENT_3D ( 'NONE', #24794, #21578, #14780 ) ;
#8954=CARTESIAN_POINT ( 'NONE',  ( -50.15972161391663064, 17.13814111569222121, 4.955022299345066550 ) ) ;
#8955=CARTESIAN_POINT ( 'NONE',  ( -29.82321757229076908, 71.17901112636586447, -1.270000000000007123 ) ) ;
#8968=AXIS2_PLACEMENT_3D ( 'NONE', #3517, #25855, #3728 ) ;
#8970=VERTEX_POINT ( 'NONE', #11963 ) ;
#8971=CIRCLE ( 'NONE', #10903, 0.5080000000000000071 ) ;
#8973=CARTESIAN_POINT ( 'NONE',  ( -8.095114962461808616, 74.19100168833409725, 1.270000000000002460 ) ) ;
#8976=CARTESIAN_POINT ( 'NONE',  ( -6.559134203278485842, 78.24119908707510263, -1.523999999999996469 ) ) ;
#8986=CARTESIAN_POINT ( 'NONE',  ( -10.53334313995851801, 65.32054992887103140, -1.523999999999996469 ) ) ;
#8987=FACE_OUTER_BOUND ( 'NONE', #37407, .T. ) ;
#8988=ADVANCED_FACE ( 'NONE', ( #7990 ), #31981, .T. ) ;
#8990=CARTESIAN_POINT ( 'NONE',  ( -58.82991071597915322, -0.2577532384647474029, -1.205395329641216235E-14 ) ) ;
#8997=AXIS2_PLACEMENT_3D ( 'NONE', #11352, #37342, #8161 ) ;
#9004=CARTESIAN_POINT ( 'NONE',  ( -36.98328822617348521, 27.82293856516311692, -1.270000000000003793 ) ) ;
#9005=EDGE_CURVE ( 'NONE', #37389, #41900, #39453, .T. ) ;
#9006=DIRECTION ( 'NONE',  ( 0.6878275643682715268, 0.7258741224862691466, 2.626171355423258178E-14 ) ) ;
#9009=CARTESIAN_POINT ( 'NONE',  ( -10.34239276132902674, 65.15305678602257444, 1.270000000000002016 ) ) ;
#9014=ORIENTED_EDGE ( 'NONE', *, *, #28731, .F. ) ;
#9015=CARTESIAN_POINT ( 'NONE',  ( -58.57480556029605623, 0.6052348492003173375, -0.1017111358178830471 ) ) ;
#9018=CARTESIAN_POINT ( 'NONE',  ( -42.60041433329272564, 22.17261999083454072, -1.881317670890401361 ) ) ;
#9025=CARTESIAN_POINT ( 'NONE',  ( -58.16583728925170504, 0.7033174012466524294, -1.177358567970812508 ) ) ;
#9033=CARTESIAN_POINT ( 'NONE',  ( -57.09878488423309051, 3.216020309495956742, -2.217633722229552351 ) ) ;
#9040=CARTESIAN_POINT ( 'NONE',  ( -58.73801720703743001, -0.4998429216807459552, -1.049519136981926467E-14 ) ) ;
#9043=CARTESIAN_POINT ( 'NONE',  ( -47.26619606798132622, 24.98193397792429593, 1.785901896324509019 ) ) ;
#9044=ADVANCED_FACE ( 'NONE', ( #35187 ), #7475, .T. ) ;
#9047=CARTESIAN_POINT ( 'NONE',  ( -32.51099854767154085, 68.28336360077705081, -1.270000000000008233 ) ) ;
#9048=ADVANCED_FACE ( 'NONE', ( #8987 ), #30561, .T. ) ;
#9049=CARTESIAN_POINT ( 'NONE',  ( -41.33672448130794663, 22.78954268934618810, -1.170983984347497842 ) ) ;
#9052=CARTESIAN_POINT ( 'NONE',  ( -58.70413935429054675, 0.2332485698458008905, 0.6626129746612759996 ) ) ;
#9053=CARTESIAN_POINT ( 'NONE',  ( -49.98362463941607814, 16.32256260904422618, 4.928702286786347919 ) ) ;
#9057=CARTESIAN_POINT ( 'NONE',  ( -52.41299847468118855, 17.00754718993399095, 1.481513115354232024 ) ) ;
#9060=CARTESIAN_POINT ( 'NONE',  ( -51.38196307026375820, 20.99359797579823805, -1.083509735914620812E-14 ) ) ;
#9063=VERTEX_POINT ( 'NONE', #15778 ) ;
#9069=VECTOR ( 'NONE', #12504, 1000.000000000000000 ) ;
#9072=CARTESIAN_POINT ( 'NONE',  ( -10.18297664959815663, 77.66688486464208552, -1.269999999999998019 ) ) ;
#9077=ORIENTED_EDGE ( 'NONE', *, *, #15470, .T. ) ;
#9079=DIRECTION ( 'NONE',  ( 0.7517731442105912709, -0.6594218222380281436, 8.537024980200781389E-16 ) ) ;
#9089=AXIS2_PLACEMENT_3D ( 'NONE', #37920, #21494, #8743 ) ;
#9101=EDGE_CURVE ( 'NONE', #514, #25107, #41489, .T. ) ;
#9104=AXIS2_PLACEMENT_3D ( 'NONE', #6583, #13390, #36194 ) ;
#9105=CARTESIAN_POINT ( 'NONE',  ( -58.29828225616458326, -0.1403253391138825912, 0.3417568066585683906 ) ) ;
#9106=CARTESIAN_POINT ( 'NONE',  ( -19.33375693323417011, 80.42273151551299293, -1.270000000000003570 ) ) ;
#9109=VERTEX_POINT ( 'NONE', #16405 ) ;
#9115=CARTESIAN_POINT ( 'NONE',  ( -28.99017888265885645, 62.64366196043476265, 1.523999999999993138 ) ) ;
#9119=CARTESIAN_POINT ( 'NONE',  ( -30.15519950990045217, 69.97033940222175374, 1.523999999999994914 ) ) ;
#9122=AXIS2_PLACEMENT_3D ( 'NONE', #4776, #33945, #14534 ) ;
#9135=ORIENTED_EDGE ( 'NONE', *, *, #37081, .T. ) ;
#9136=CARTESIAN_POINT ( 'NONE',  ( -55.14069116334857767, 5.401725095812811794, 0.2259897844577825055 ) ) ;
#9147=DIRECTION ( 'NONE',  ( -0.7548010569845216011, -0.6559537821943317581, -2.801824109679580762E-16 ) ) ;
#9148=EDGE_CURVE ( 'NONE', #27418, #36699, #22389, .T. ) ;
#9152=CARTESIAN_POINT ( 'NONE',  ( -46.85193236286590945, 25.57103397218990182, 1.585296040148151286 ) ) ;
#9153=CARTESIAN_POINT ( 'NONE',  ( -46.72388148998840762, 26.09838203902186393, -8.130785423271672580E-15 ) ) ;
#9155=CARTESIAN_POINT ( 'NONE',  ( -43.24646561529713296, 21.63922848039483071, 2.381786957946262273 ) ) ;
#9157=EDGE_CURVE ( 'NONE', #31300, #18130, #25811, .T. ) ;
#9159=ORIENTED_EDGE ( 'NONE', *, *, #20134, .F. ) ;
#9165=CARTESIAN_POINT ( 'NONE',  ( -54.78025980062105305, 10.68576047822487141, -1.034243702897348038E-14 ) ) ;
#9169=DIRECTION ( 'NONE',  ( 5.188838149069472160E-16, -1.699382548006136559E-16, -1.000000000000000000 ) ) ;
#9183=EDGE_LOOP ( 'NONE', ( #17530, #5853, #23490, #30392 ) ) ;
#9184=ORIENTED_EDGE ( 'NONE', *, *, #15618, .T. ) ;
#9188=LINE ( 'NONE', #12166, #36822 ) ;
#9196=ORIENTED_EDGE ( 'NONE', *, *, #40122, .T. ) ;
#9199=CYLINDRICAL_SURFACE ( 'NONE', #26574, 0.2539999999999998925 ) ;
#9216=DIRECTION ( 'NONE',  ( 5.188838149069472160E-16, -1.699382548006136559E-16, -1.000000000000000000 ) ) ;
#9232=CARTESIAN_POINT ( 'NONE',  ( -55.72094646625244252, 5.847107909200485842, -2.941330550160955681 ) ) ;
#9234=CARTESIAN_POINT ( 'NONE',  ( -58.31893842775842529, -0.1844529990628340776, -0.2851935484599126269 ) ) ;
#9240=ADVANCED_FACE ( 'NONE', ( #3869 ), #38589, .F. ) ;
#9243=CARTESIAN_POINT ( 'NONE',  ( -52.30895062419047292, 13.66434875625866674, -4.401212925246500873 ) ) ;
#9244=ADVANCED_FACE ( 'NONE', ( #19187 ), #22782, .T. ) ;
#9246=AXIS2_PLACEMENT_3D ( 'NONE', #32531, #28702, #15495 ) ;
#9252=EDGE_CURVE ( 'NONE', #36653, #5054, #9496, .T. ) ;
#9255=DIRECTION ( 'NONE',  ( -0.6294287539883980376, -0.7770581983690878491, -1.945484789722745799E-16 ) ) ;
#9258=CARTESIAN_POINT ( 'NONE',  ( -53.00789483126595769, 12.40033530745290236, -4.180047681284821515 ) ) ;
#9259=CARTESIAN_POINT ( 'NONE',  ( -49.58053446479453186, 16.59387910164543456, -4.528212452174721570 ) ) ;
#9261=CARTESIAN_POINT ( 'NONE',  ( -5.809227842914837403, 77.60418761620948658, -1.523999999999996025 ) ) ;
#9262=CARTESIAN_POINT ( 'NONE',  ( -56.78650302187183740, 3.241477563879227475, 2.205756828360251109 ) ) ;
#9263=CARTESIAN_POINT ( 'NONE',  ( -51.64658268050072820, 13.54811038370313447, 4.518953239828090496 ) ) ;
#9266=CARTESIAN_POINT ( 'NONE',  ( -56.10358335640970751, 6.949471795635917104, 1.762666882438575611 ) ) ;
#9269=CIRCLE ( 'NONE', #33088, 0.2539999999999989488 ) ;
#9270=EDGE_LOOP ( 'NONE', ( #84, #8091, #6251, #5672 ) ) ;
#9271=CARTESIAN_POINT ( 'NONE',  ( -54.91040913962392978, 10.45702928859090086, -1.592171597931419491 ) ) ;
#9279=CARTESIAN_POINT ( 'NONE',  ( -6.559134203278485842, 78.24119908707510263, -1.269999999999996465 ) ) ;
#9285=DIRECTION ( 'NONE',  ( 5.188838149069472160E-16, -1.699382548006136559E-16, -1.000000000000000000 ) ) ;
#9286=CYLINDRICAL_SURFACE ( 'NONE', #32960, 0.2540000000000000036 ) ;
#9289=CARTESIAN_POINT ( 'NONE',  ( -58.36875020124374913, -0.2893854339803315634, -0.03832961079136332910 ) ) ;
#9300=DIRECTION ( 'NONE',  ( 5.188838149069472160E-16, -1.699382548006136559E-16, -1.000000000000000000 ) ) ;
#9302=CARTESIAN_POINT ( 'NONE',  ( -47.11704014324645584, 20.18577099567727373, -5.127035723291441194 ) ) ;
#9303=AXIS2_PLACEMENT_3D ( 'NONE', #1146, #7742, #314 ) ;
#9304=EDGE_LOOP ( 'NONE', ( #12848, #8918, #14565, #2645 ) ) ;
#9307=CARTESIAN_POINT ( 'NONE',  ( -46.38316532014824389, 26.05065462784537900, -1.270000000000008233 ) ) ;
#9313=AXIS2_PLACEMENT_3D ( 'NONE', #23460, #36487, #21521 ) ;
#9317=DIRECTION ( 'NONE',  ( 0.8745520943968235761, -0.4849315768086558398, 4.268512490100410909E-16 ) ) ;
#9321=ORIENTED_EDGE ( 'NONE', *, *, #3768, .T. ) ;
#9323=CARTESIAN_POINT ( 'NONE',  ( -28.96638701337642985, 63.08302880242272437, 1.523999999999993582 ) ) ;
#9325=DIRECTION ( 'NONE',  ( -5.188838149069471174E-16, 1.699382548006136313E-16, 1.000000000000000000 ) ) ;
#9326=CIRCLE ( 'NONE', #9979, 0.2540000000000052771 ) ;
#9327=CARTESIAN_POINT ( 'NONE',  ( -8.584014518950162653, 73.13423810798758495, 1.524000000000002686 ) ) ;
#9331=CARTESIAN_POINT ( 'NONE',  ( -50.55264109713811393, 15.40887103989715889, -4.805487048246964932 ) ) ;
#9337=ORIENTED_EDGE ( 'NONE', *, *, #34423, .T. ) ;
#9340=DIRECTION ( 'NONE',  ( -5.188838149069472160E-16, 1.699382548006136559E-16, 1.000000000000000000 ) ) ;
#9344=ORIENTED_EDGE ( 'NONE', *, *, #7412, .F. ) ;
#9350=VECTOR ( 'NONE', #25753, 1000.000000000000000 ) ;
#9352=CARTESIAN_POINT ( 'NONE',  ( -29.91360363449004822, 70.04874496952839991, 1.523999999999992250 ) ) ;
#9354=CARTESIAN_POINT ( 'NONE',  ( -46.69554899239189183, 26.06112269829689865, 0.4657571695567544467 ) ) ;
#9356=CARTESIAN_POINT ( 'NONE',  ( -47.67648637180144533, 19.71513033058998232, 5.327979952964769339 ) ) ;
#9383=ORIENTED_EDGE ( 'NONE', *, *, #25098, .T. ) ;
#9385=LINE ( 'NONE', #5791, #39904 ) ;
#9397=CARTESIAN_POINT ( 'NONE',  ( -17.64290547347870941, 83.78857423953914463, -1.524000000000003130 ) ) ;
#9412=CARTESIAN_POINT ( 'NONE',  ( -7.842268484490568348, 73.30875693322846587, 1.270000000000002904 ) ) ;
#9413=DIRECTION ( 'NONE',  ( -0.6294287539884013682, -0.7770581983690854067, 6.679558114607144468E-15 ) ) ;
#9421=ORIENTED_EDGE ( 'NONE', *, *, #33484, .T. ) ;
#9424=CARTESIAN_POINT ( 'NONE',  ( -41.63373767251972168, 22.51256436878228939, -1.325597493795125370 ) ) ;
#9430=CARTESIAN_POINT ( 'NONE',  ( -58.44674015341568918, 0.09518567107959752249, -0.7847720614711276577 ) ) ;
#9432=CARTESIAN_POINT ( 'NONE',  ( -58.62884620442462591, -0.7615560826026042118, -0.07633319197460453065 ) ) ;
#9436=FACE_OUTER_BOUND ( 'NONE', #30737, .T. ) ;
#9437=CIRCLE ( 'NONE', #8069, 0.5080000000000000071 ) ;
#9439=CIRCLE ( 'NONE', #38699, 0.3810000000000015041 ) ;
#9441=CARTESIAN_POINT ( 'NONE',  ( -58.73801720703743001, -0.4998429216807459552, -1.049519136981926467E-14 ) ) ;
#9442=ORIENTED_EDGE ( 'NONE', *, *, #3453, .T. ) ;
#9445=ORIENTED_EDGE ( 'NONE', *, *, #20644, .T. ) ;
#9449=CARTESIAN_POINT ( 'NONE',  ( -48.50421218116025557, 14.67712143704001626, -8.170758227952415863E-15 ) ) ;
#9456=LINE ( 'NONE', #13066, #14029 ) ;
#9460=CARTESIAN_POINT ( 'NONE',  ( -45.37978287637889707, 19.43610829578849675, -1.699483007375131249 ) ) ;
#9461=ORIENTED_EDGE ( 'NONE', *, *, #42058, .T. ) ;
#9463=CARTESIAN_POINT ( 'NONE',  ( -47.01877684503696742, 24.36789988528162354, 2.430126310640454257 ) ) ;
#9464=CARTESIAN_POINT ( 'NONE',  ( -56.40692165385873125, 4.437999542203786341, 2.560908555091980787 ) ) ;
#9466=EDGE_CURVE ( 'NONE', #30610, #40365, #36081, .T. ) ;
#9467=FACE_OUTER_BOUND ( 'NONE', #32191, .T. ) ;
#9468=CARTESIAN_POINT ( 'NONE',  ( -53.89938688035451975, 11.68864614896874343, 3.017114338529855111 ) ) ;
#9470=ORIENTED_EDGE ( 'NONE', *, *, #5123, .F. ) ;
#9471=CARTESIAN_POINT ( 'NONE',  ( -55.45615287082594591, 8.171946630687445534, -2.478682617993501758 ) ) ;
#9478=CYLINDRICAL_SURFACE ( 'NONE', #17257, 0.6350000000000006750 ) ;
#9484=DIRECTION ( 'NONE',  ( 5.188838149069472160E-16, -1.699382548006136559E-16, -1.000000000000000000 ) ) ;
#9486=ORIENTED_EDGE ( 'NONE', *, *, #20344, .T. ) ;
#9489=CARTESIAN_POINT ( 'NONE',  ( -58.34965918702084764, -0.2493686153283701523, -0.1767538080080786056 ) ) ;
#9496=CIRCLE ( 'NONE', #33348, 3.111499999999999932 ) ;
#9499=CIRCLE ( 'NONE', #29223, 9.048749999999994742 ) ;
#9501=DIRECTION ( 'NONE',  ( -0.8745520943968250194, 0.4849315768086535083, -5.424246918827963022E-16 ) ) ;
#9502=CARTESIAN_POINT ( 'NONE',  ( -42.79661761208809168, 21.81806929429799879, -2.089873509012822428 ) ) ;
#9504=ORIENTED_EDGE ( 'NONE', *, *, #14506, .T. ) ;
#9507=LINE ( 'NONE', #9718, #35961 ) ;
#9515=AXIS2_PLACEMENT_3D ( 'NONE', #11913, #24901, #2131 ) ;
#9525=ORIENTED_EDGE ( 'NONE', *, *, #7643, .F. ) ;
#9528=CARTESIAN_POINT ( 'NONE',  ( -16.46263872254443683, 83.91929436251373886, -1.270000000000002460 ) ) ;
#9533=CARTESIAN_POINT ( 'NONE',  ( -7.772068811996249771, 69.25462295839062676, -1.269999999999995577 ) ) ;
#9541=AXIS2_PLACEMENT_3D ( 'NONE', #36874, #13440, #32828 ) ;
#9542=CARTESIAN_POINT ( 'NONE',  ( -46.38316532014824389, 26.05065462784537900, 1.269999999999990914 ) ) ;
#9547=CARTESIAN_POINT ( 'NONE',  ( -29.91139568370676116, 83.95719535527391031, -1.270000000000009566 ) ) ;
#9550=DIRECTION ( 'NONE',  ( -0.9454731675810359448, 0.3256999990547780333, -5.459396135145339171E-16 ) ) ;
#9554=CARTESIAN_POINT ( 'NONE',  ( -50.94359596358804509, 14.56251409809150132, 4.558007702229759595 ) ) ;
#9555=CARTESIAN_POINT ( 'NONE',  ( -46.93986413309943373, 25.37947832266650039, 1.074976477481959902 ) ) ;
#9556=CIRCLE ( 'NONE', #39540, 0.2540000000000012248 ) ;
#9557=DIRECTION ( 'NONE',  ( 5.188838149069472160E-16, -1.699382548006136559E-16, -1.000000000000000000 ) ) ;
#9559=CARTESIAN_POINT ( 'NONE',  ( -48.56815661899837977, 19.24492339269602681, 5.224590812749973168 ) ) ;
#9560=CARTESIAN_POINT ( 'NONE',  ( -58.67901903226392335, -0.3139884119181903799, 0.3104539207526157418 ) ) ;
#9562=CARTESIAN_POINT ( 'NONE',  ( -58.16721443865020547, 0.09938604254088045931, -0.2878065994480087375 ) ) ;
#9564=ORIENTED_EDGE ( 'NONE', *, *, #32332, .T. ) ;
#9565=ORIENTED_EDGE ( 'NONE', *, *, #19873, .F. ) ;
#9575=DIRECTION ( 'NONE',  ( 0.3256999990547876367, 0.9454731675810326141, 8.328397965208553695E-18 ) ) ;
#9583=ORIENTED_EDGE ( 'NONE', *, *, #37125, .F. ) ;
#9584=DIRECTION ( 'NONE',  ( -0.8745520943968249084, 0.4849315768086533418, -5.271987356194193006E-16 ) ) ;
#9598=CARTESIAN_POINT ( 'NONE',  ( -26.51793118801306548, 72.98537704160715123, 1.269999999999993134 ) ) ;
#9599=VECTOR ( 'NONE', #713, 1000.000000000000227 ) ;
#9603=ORIENTED_EDGE ( 'NONE', *, *, #22178, .T. ) ;
#9624=AXIS2_PLACEMENT_3D ( 'NONE', #33950, #14748, #20719 ) ;
#9626=DIRECTION ( 'NONE',  ( 0.8745520943968249084, -0.4849315768086533418, 5.271987356194193006E-16 ) ) ;
#9632=DIRECTION ( 'NONE',  ( -0.7517731442105912709, 0.6594218222380281436, -8.537024980200781389E-16 ) ) ;
#9634=CARTESIAN_POINT ( 'NONE',  ( -30.75918919842648336, 69.77432548395512413, 1.269999999999991358 ) ) ;
#9639=CARTESIAN_POINT ( 'NONE',  ( -58.35071543880859934, 0.3020958082991723748, -0.9346586068229112421 ) ) ;
#9640=B_SPLINE_CURVE_WITH_KNOTS ( 'NONE', 3,
 ( #10086, #32259, #3294, #3088, #3723, #38655, #38859, #9874, #9463, #35884, #32465, #16258 ),
 .UNSPECIFIED., .F., .F.,
 ( 4, 1, 1, 1, 1, 1, 1, 1, 1, 4 ),
 ( 0.7354344192538688763, 0.7500000000000001110, 0.7685053377236187311, 0.8015760037631017854, 0.8346466698025848396, 0.8677173358420678939, 0.9007880018815509482, 0.9338586679210340025, 0.9503940009407755296, 0.9543042185119943177 ),
 .UNSPECIFIED. ) ;
#9641=ORIENTED_EDGE ( 'NONE', *, *, #633, .T. ) ;
#9642=CARTESIAN_POINT ( 'NONE',  ( -54.09072575249082604, 8.649776409409795974, -3.422340198163621228 ) ) ;
#9645=DIRECTION ( 'NONE',  ( -0.7770581983690852956, 0.6294287539884014793, -4.360450048231382406E-16 ) ) ;
#9648=CARTESIAN_POINT ( 'NONE',  ( -58.55221842960730783, 0.5754175076986972615, -0.9757793345693789311 ) ) ;
#9649=EDGE_LOOP ( 'NONE', ( #39084, #24342, #23298, #9525 ) ) ;
#9652=ORIENTED_EDGE ( 'NONE', *, *, #22054, .F. ) ;
#9657=DIRECTION ( 'NONE',  ( 0.8745520943968243532, -0.4849315768086547296, 6.829619984160642269E-16 ) ) ;
#9658=ADVANCED_FACE ( 'NONE', ( #37475 ), #11699, .T. ) ;
#9662=EDGE_CURVE ( 'NONE', #32297, #10127, #31717, .T. ) ;
#9666=AXIS2_PLACEMENT_3D ( 'NONE', #34154, #1781, #21333 ) ;
#9667=CARTESIAN_POINT ( 'NONE',  ( -48.90916507497669841, 16.41193755240580288, -3.099911505780766685 ) ) ;
#9668=ORIENTED_EDGE ( 'NONE', *, *, #14971, .T. ) ;
#9669=CARTESIAN_POINT ( 'NONE',  ( -4.476425760464393555, 71.61790547347303004, 1.270000000000005791 ) ) ;
#9671=CARTESIAN_POINT ( 'NONE',  ( -48.84267179513337709, 18.06759678302662309, 5.143183091231904314 ) ) ;
#9674=CARTESIAN_POINT ( 'NONE',  ( -17.65389921742009705, 84.42347906515803402, -1.270000000000003348 ) ) ;
#9675=CARTESIAN_POINT ( 'NONE',  ( -55.24575511360421842, 11.19612964283526324, 0.2458718103055573534 ) ) ;
#9676=CARTESIAN_POINT ( 'NONE',  ( -57.78858274104275949, 1.044662872677112997, 1.355440516197746303 ) ) ;
#9679=EDGE_LOOP ( 'NONE', ( #14141, #9486, #6864, #39199 ) ) ;
#9680=CARTESIAN_POINT ( 'NONE',  ( -54.68578128245503223, 13.03233524004687638, -1.089573673074214656E-14 ) ) ;
#9687=DIRECTION ( 'NONE',  ( -0.8745520943968249084, 0.4849315768086533418, -5.271987356194193006E-16 ) ) ;
#9690=CARTESIAN_POINT ( 'NONE',  ( -20.05275907367747124, 79.68882802557934042, -1.270000000000003793 ) ) ;
#9693=DIRECTION ( 'NONE',  ( 0.3086833358529555982, -0.9511648638205112416, 1.501066210750423308E-13 ) ) ;
#9698=ADVANCED_FACE ( 'NONE', ( #12123 ), #21272, .T. ) ;
#9699=CARTESIAN_POINT ( 'NONE',  ( -58.34883683990797465, -0.2476419964839868537, -0.1803091383267578784 ) ) ;
#9705=DIRECTION ( 'NONE',  ( -0.1565721916417968096, -0.9876665170007964401, 0.000000000000000000 ) ) ;
#9707=AXIS2_PLACEMENT_3D ( 'NONE', #35392, #22162, #19191 ) ;
#9709=ORIENTED_EDGE ( 'NONE', *, *, #17586, .T. ) ;
#9714=CARTESIAN_POINT ( 'NONE',  ( -41.88683177698051452, 22.33947639032530219, -1.656270940288501636 ) ) ;
#9718=CARTESIAN_POINT ( 'NONE',  ( -30.45812239790965492, 71.16801738242446618, 1.269999999999991358 ) ) ;
#9719=AXIS2_PLACEMENT_3D ( 'NONE', #20299, #16486, #13928 ) ;
#9727=B_SPLINE_CURVE_WITH_KNOTS ( 'NONE', 3,
 ( #989, #17147, #32937, #36352 ),
 .UNSPECIFIED., .F., .F.,
 ( 4, 4 ),
 ( 0.7699389564571422762, 1.000000000000000000 ),
 .UNSPECIFIED. ) ;
#9729=ORIENTED_EDGE ( 'NONE', *, *, #3047, .T. ) ;
#9731=CARTESIAN_POINT ( 'NONE',  ( -8.270297712355500153, 69.35377921309405735, -1.269999999999995799 ) ) ;
#9736=ORIENTED_EDGE ( 'NONE', *, *, #36593, .T. ) ;
#9739=FACE_OUTER_BOUND ( 'NONE', #32309, .T. ) ;
#9740=CARTESIAN_POINT ( 'NONE',  ( -3.911441847776591096, 70.75305732235845824, -1.523999999999993804 ) ) ;
#9758=ADVANCED_FACE ( 'NONE', ( #2765 ), #15720, .T. ) ;
#9762=CARTESIAN_POINT ( 'NONE',  ( -4.476425760464393555, 71.61790547347303004, -1.523999999999994248 ) ) ;
#9766=AXIS2_PLACEMENT_3D ( 'NONE', #33440, #27454, #1697 ) ;
#9768=CARTESIAN_POINT ( 'NONE',  ( -47.05348687143031583, 24.98710001375500056, 1.566218509541806636 ) ) ;
#9770=CARTESIAN_POINT ( 'NONE',  ( -47.35944255389382818, 21.37623662739424191, 4.722871667523163453 ) ) ;
#9774=ORIENTED_EDGE ( 'NONE', *, *, #37346, .T. ) ;
#9781=CARTESIAN_POINT ( 'NONE',  ( -8.594951744493888768, 74.76616009375631222, -1.269999999999996909 ) ) ;
#9782=CARTESIAN_POINT ( 'NONE',  ( -7.921807157844599878, 72.80702234259206307, 1.270000000000002682 ) ) ;
#9793=AXIS2_PLACEMENT_3D ( 'NONE', #35885, #10512, #39073 ) ;
#9795=CIRCLE ( 'NONE', #15227, 8.794749999999996959 ) ;
#9802=CARTESIAN_POINT ( 'NONE',  ( -47.74911022259793469, 17.86741523025699152, 3.129844374475859947 ) ) ;
#9818=CARTESIAN_POINT ( 'NONE',  ( -58.82782897837036984, -0.2608788304230558186, 0.04583423360467810820 ) ) ;
#9830=FACE_OUTER_BOUND ( 'NONE', #4547, .T. ) ;
#9831=DIRECTION ( 'NONE',  ( 5.188838149069472160E-16, -1.699382548006136559E-16, -1.000000000000000000 ) ) ;
#9839=ORIENTED_EDGE ( 'NONE', *, *, #18824, .F. ) ;
#9841=ORIENTED_EDGE ( 'NONE', *, *, #2962, .F. ) ;
#9842=DIRECTION ( 'NONE',  ( 0.1565721916418019999, 0.9876665170007956629, -8.659954811667593930E-17 ) ) ;
#9847=CARTESIAN_POINT ( 'NONE',  ( -58.77082881926929048, -0.3034670599615398867, -0.1967669022685080149 ) ) ;
#9852=DIRECTION ( 'NONE',  ( 0.6294287539883844929, 0.7770581983690987293, 0.000000000000000000 ) ) ;
#9855=CARTESIAN_POINT ( 'NONE',  ( -58.10099831372669854, 0.3475205698689753930, -0.9728495803591354907 ) ) ;
#9856=ORIENTED_EDGE ( 'NONE', *, *, #10274, .T. ) ;
#9859=ORIENTED_EDGE ( 'NONE', *, *, #28255, .F. ) ;
#9863=CARTESIAN_POINT ( 'NONE',  ( -57.89731077922513691, 0.5615449381113218896, -1.034775302914740585E-14 ) ) ;
#9867=DIRECTION ( 'NONE',  ( -0.7445787077807538568, -0.6675346791886865860, 0.000000000000000000 ) ) ;
#9870=CARTESIAN_POINT ( 'NONE',  ( -49.01671973967521012, 18.67808020721676954, -5.174630477995056488 ) ) ;
#9871=CARTESIAN_POINT ( 'NONE',  ( -48.96835380800505533, 15.76965437727898056, -2.261121166259650650 ) ) ;
#9872=DIRECTION ( 'NONE',  ( 5.188838149069472160E-16, -1.699382548006136559E-16, -1.000000000000000000 ) ) ;
#9873=DIRECTION ( 'NONE',  ( 5.188838149069472160E-16, -1.699382548006136559E-16, -1.000000000000000000 ) ) ;
#9874=CARTESIAN_POINT ( 'NONE',  ( -47.04217617083259029, 23.73857702128102076, 2.948847133965281309 ) ) ;
#9875=FACE_OUTER_BOUND ( 'NONE', #13763, .T. ) ;
#9879=CARTESIAN_POINT ( 'NONE',  ( -17.14500000000466784, 71.11999999999886768, -1.270000000000000684 ) ) ;
#9880=CARTESIAN_POINT ( 'NONE',  ( -55.59033409382031721, 8.645621179197947370, 1.431546819705146634 ) ) ;
#9881=CARTESIAN_POINT ( 'NONE',  ( -55.60486134785667645, 7.243031971518515633, 3.140198620020484110 ) ) ;
#9884=CARTESIAN_POINT ( 'NONE',  ( -53.04800011021367112, 17.61732480354184815, -1.091987273408484482E-14 ) ) ;
#9886=ORIENTED_EDGE ( 'NONE', *, *, #4338, .T. ) ;
#9894=DIRECTION ( 'NONE',  ( -0.7258741224889101451, 0.6878275643654844229, -8.537024980200846470E-16 ) ) ;
#9897=CARTESIAN_POINT ( 'NONE',  ( -17.14500000000466784, 71.11999999999886768, 1.269999999999998241 ) ) ;
#9898=FACE_OUTER_BOUND ( 'NONE', #29952, .T. ) ;
#9900=AXIS2_PLACEMENT_3D ( 'NONE', #27812, #40820, #5463 ) ;
#9902=ORIENTED_EDGE ( 'NONE', *, *, #41610, .T. ) ;
#9903=DIRECTION ( 'NONE',  ( 5.188838149069472160E-16, -1.699382548006136559E-16, -1.000000000000000000 ) ) ;
#9918=APPLICATION_CONTEXT ( 'automotive_design' ) ;
#9920=CARTESIAN_POINT ( 'NONE',  ( -47.87216941255763203, 19.82042534259524658, -5.426529464407940928 ) ) ;
#9921=ORIENTED_EDGE ( 'NONE', *, *, #15276, .T. ) ;
#9929=CIRCLE ( 'NONE', #5212, 0.2539999999999998925 ) ;
#9931=DIRECTION ( 'NONE',  ( -5.188838149069471174E-16, 1.699382548006136313E-16, 1.000000000000000000 ) ) ;
#9942=ORIENTED_EDGE ( 'NONE', *, *, #9157, .T. ) ;
#9955=VECTOR ( 'NONE', #16115, 1000.000000000000114 ) ;
#9957=EDGE_LOOP ( 'NONE', ( #35939, #10268, #5428, #18809 ) ) ;
#9963=EDGE_CURVE ( 'NONE', #30709, #27023, #13378, .T. ) ;
#9964=VERTEX_POINT ( 'NONE', #41736 ) ;
#9966=DIRECTION ( 'NONE',  ( 0.9876665170007969952, -0.1565721916417935344, 5.390917751951444915E-16 ) ) ;
#9967=CARTESIAN_POINT ( 'NONE',  ( -9.909999474182706436, 76.95545850745379823, -1.269999999999998019 ) ) ;
#9972=CARTESIAN_POINT ( 'NONE',  ( -48.37037162488499575, 18.71529471574935499, 5.180666589218357210 ) ) ;
#9973=CARTESIAN_POINT ( 'NONE',  ( -47.22545206610593027, 24.52529105818055655, 1.461865184087808966 ) ) ;
#9975=CARTESIAN_POINT ( 'NONE',  ( -50.58884987432006852, 15.93229845861179861, 5.010371253631904942 ) ) ;
#9976=CARTESIAN_POINT ( 'NONE',  ( -58.82993613934316812, -0.2576853927351192564, 0.02220333243337114723 ) ) ;
#9978=DIRECTION ( 'NONE',  ( -0.5149185422762269093, 0.8572391118119411235, 5.959261578127985974E-15 ) ) ;
#9979=AXIS2_PLACEMENT_3D ( 'NONE', #18191, #2036, #5663 ) ;
#9980=ORIENTED_EDGE ( 'NONE', *, *, #21698, .T. ) ;
#9986=CARTESIAN_POINT ( 'NONE',  ( -46.69554899239189183, 26.06112269829689865, -0.4657571695567720438 ) ) ;
#9989=EDGE_CURVE ( 'NONE', #25607, #6738, #13491, .T. ) ;
#9990=DIRECTION ( 'NONE',  ( 5.188838149069472160E-16, -1.699382548006136559E-16, -1.000000000000000000 ) ) ;
#9993=DIRECTION ( 'NONE',  ( 0.9336303900108808840, 0.3582377630124027879, -6.739313779395947471E-16 ) ) ;
#10007=EDGE_LOOP ( 'NONE', ( #15754, #10890, #18680, #17695 ) ) ;
#10008=ORIENTED_EDGE ( 'NONE', *, *, #22058, .F. ) ;
#10009=CARTESIAN_POINT ( 'NONE',  ( -45.15528325240633478, 20.88806775524793125, 3.529375091719462176 ) ) ;
#10010=EDGE_CURVE ( 'NONE', #5685, #24684, #2526, .T. ) ;
#10021=AXIS2_PLACEMENT_3D ( 'NONE', #4108, #39883, #36471 ) ;
#10025=DIRECTION ( 'NONE',  ( -0.8745520943968236871, 0.4849315768086559508, -6.829619984160659032E-16 ) ) ;
#10044=DIRECTION ( 'NONE',  ( 0.9876665170007953298, -0.1565721916418034432, 5.390917751951452804E-16 ) ) ;
#10048=ADVANCED_FACE ( 'NONE', ( #29574 ), #26366, .F. ) ;
#10058=CARTESIAN_POINT ( 'NONE',  ( -58.63621593477581229, -0.3005977173826933635, -0.3593407213355099827 ) ) ;
#10064=CARTESIAN_POINT ( 'NONE',  ( -46.85406979095059654, 20.44882429329730655, 5.016006923199691769 ) ) ;
#10067=CARTESIAN_POINT ( 'NONE',  ( -57.97566020452313040, 1.918554019021911916, -1.632400077439718933 ) ) ;
#10068=VERTEX_POINT ( 'NONE', #10809 ) ;
#10071=VERTEX_POINT ( 'NONE', #23791 ) ;
#10076=DIRECTION ( 'NONE',  ( -5.188838149069471174E-16, 1.699382548006136313E-16, 1.000000000000000000 ) ) ;
#10083=CARTESIAN_POINT ( 'NONE',  ( -48.35712625370394591, 16.55775765112550602, -2.292466156223463614 ) ) ;
#10084=DIRECTION ( 'NONE',  ( -0.8745520943968235761, 0.4849315768086558398, -4.268512490100410909E-16 ) ) ;
#10086=CARTESIAN_POINT ( 'NONE',  ( -48.28978369826177186, 19.63653578263565436, 5.206999999995388428 ) ) ;
#10087=CARTESIAN_POINT ( 'NONE',  ( -7.772068811996249771, 69.25462295839062676, -1.523999999999995580 ) ) ;
#10088=CARTESIAN_POINT ( 'NONE',  ( -58.32289719230551839, -0.2069853552843642364, -0.1059582036190383214 ) ) ;
#10091=CARTESIAN_POINT ( 'NONE',  ( -15.27962295839633811, 80.49293118800726177, -1.270000000000001350 ) ) ;
#10092=CARTESIAN_POINT ( 'NONE',  ( -28.42835727709238114, 77.69497285144578314, -1.524000000000007793 ) ) ;
#10093=CARTESIAN_POINT ( 'NONE',  ( -55.15137202863810728, 10.98262019425784430, 0.5441000652715827224 ) ) ;
#10094=CARTESIAN_POINT ( 'NONE',  ( -55.65298819915649631, 5.540485941798511504, 2.823722248809245272 ) ) ;
#10096=ORIENTED_EDGE ( 'NONE', *, *, #23687, .F. ) ;
#10097=CARTESIAN_POINT ( 'NONE',  ( -52.06588384925056801, 19.72955628943436679, -1.090601490622711080E-14 ) ) ;
#10099=AXIS2_PLACEMENT_3D ( 'NONE', #10299, #29475, #23059 ) ;
#10101=CARTESIAN_POINT ( 'NONE',  ( -26.51793118801306548, 72.98537704160715123, -1.270000000000006013 ) ) ;
#10113=CYLINDRICAL_SURFACE ( 'NONE', #39757, 0.2539999999999997260 ) ;
#10114=ORIENTED_EDGE ( 'NONE', *, *, #24172, .T. ) ;
#10118=DIRECTION ( 'NONE',  ( -0.6559537821943240976, 0.7548010569845284845, -4.686333752532409839E-16 ) ) ;
#10124=DIRECTION ( 'NONE',  ( -0.6294287539884068083, -0.7770581983690809658, -9.357678942267682069E-16 ) ) ;
#10127=VERTEX_POINT ( 'NONE', #4448 ) ;
#10131=CARTESIAN_POINT ( 'NONE',  ( -47.02779878473986486, 24.11651466984139702, -2.637840241488492943 ) ) ;
#10134=AXIS2_PLACEMENT_3D ( 'NONE', #4561, #5191, #4356 ) ;
#10135=DIRECTION ( 'NONE',  ( 0.5149185422762211362, -0.8572391118119444542, 0.000000000000000000 ) ) ;
#10137=B_SPLINE_CURVE_WITH_KNOTS ( 'NONE', 3,
 ( #7077, #10251, #16426, #23224, #15796, #2837, #29214, #36256, #19414, #13025, #41821, #19616 ),
 .UNSPECIFIED., .F., .F.,
 ( 4, 1, 1, 1, 1, 1, 1, 1, 1, 4 ),
 ( 0.7354344192538665448, 0.7685053377236187311, 0.8015760037631016743, 0.8346466698025848396, 0.8677173358420678939, 0.9007880018815508372, 0.9173233349012923643, 0.9338586679210338914, 0.9503940009407754186, 0.9543042185119922083 ),
 .UNSPECIFIED. ) ;
#10142=DIRECTION ( 'NONE',  ( 0.000000000000000000, 0.000000000000000000, 1.000000000000000000 ) ) ;
#10145=ORIENTED_EDGE ( 'NONE', *, *, #9005, .T. ) ;
#10152=ORIENTED_EDGE ( 'NONE', *, *, #3924, .T. ) ;
#10158=AXIS2_PLACEMENT_3D ( 'NONE', #23127, #36164, #38930 ) ;
#10162=CIRCLE ( 'NONE', #39429, 0.6350000000000014522 ) ;
#10163=CARTESIAN_POINT ( 'NONE',  ( -28.36525985791271154, 77.02308833105713859, 1.269999999999992468 ) ) ;
#10172=CARTESIAN_POINT ( 'NONE',  ( -41.62422838180557960, 22.52195256220192832, 1.324149224697090954 ) ) ;
#10184=CARTESIAN_POINT ( 'NONE',  ( -49.73866923540565210, 16.61554395881175594, 4.889435247958469510 ) ) ;
#10185=CARTESIAN_POINT ( 'NONE',  ( -50.57586884603683330, 21.47051451305503988, 0.7809936997224511401 ) ) ;
#10187=CARTESIAN_POINT ( 'NONE',  ( -54.32300027520380326, 9.724537220608771904, 3.743864951777626349 ) ) ;
#10188=CARTESIAN_POINT ( 'NONE',  ( -58.78603281983694018, -0.2970393704508183519, 0.1722180483736777401 ) ) ;
#10192=VERTEX_POINT ( 'NONE', #27420 ) ;
#10209=DIRECTION ( 'NONE',  ( -5.188838149069471174E-16, 1.699382548006136313E-16, 1.000000000000000000 ) ) ;
#10216=PRODUCT_DEFINITION ( 'UNKNOWN', '', #37986, #7381 ) ;
#10217=CARTESIAN_POINT ( 'NONE',  ( -47.20049172920048619, 19.11349993950443249, 3.907078929042784310 ) ) ;
#10225=DIRECTION ( 'NONE',  ( 0.7308269722843274696, -0.6825627711659368879, 8.537024980200725183E-16 ) ) ;
#10230=EDGE_LOOP ( 'NONE', ( #24208, #38414, #30695, #18629 ) ) ;
#10231=CARTESIAN_POINT ( 'NONE',  ( -9.960492004070040650, 64.81807050032566053, -1.523999999999996025 ) ) ;
#10232=ADVANCED_FACE ( 'NONE', ( #4235 ), #16984, .F. ) ;
#10235=AXIS2_PLACEMENT_3D ( 'NONE', #13151, #3368, #6554 ) ;
#10251=CARTESIAN_POINT ( 'NONE',  ( -48.08949201794742123, 19.91830422262442468, -5.194343260851647770 ) ) ;
#10257=ORIENTED_EDGE ( 'NONE', *, *, #102, .F. ) ;
#10258=DIRECTION ( 'NONE',  ( 0.3256999990547876367, 0.9454731675810326141, 8.328397965208553695E-18 ) ) ;
#10263=VECTOR ( 'NONE', #39835, 1000.000000000000227 ) ;
#10266=CARTESIAN_POINT ( 'NONE',  ( -58.81729092949609594, -0.2729283875645143742, -0.09353142974602446369 ) ) ;
#10268=ORIENTED_EDGE ( 'NONE', *, *, #8709, .F. ) ;
#10274=EDGE_CURVE ( 'NONE', #17215, #30025, #11021, .T. ) ;
#10278=CARTESIAN_POINT ( 'NONE',  ( -57.50953982388014651, 1.662011999372992044, -1.631050346940590812 ) ) ;
#10282=ORIENTED_EDGE ( 'NONE', *, *, #25832, .T. ) ;
#10288=CARTESIAN_POINT ( 'NONE',  ( -58.10259267898809554, 0.2821446311938036189, 0.7168088428568702986 ) ) ;
#10292=EDGE_CURVE ( 'NONE', #514, #32447, #26316, .T. ) ;
#10296=CARTESIAN_POINT ( 'NONE',  ( -19.97113776634630611, 79.44829951959813741, 1.269999999999995799 ) ) ;
#10297=CARTESIAN_POINT ( 'NONE',  ( -50.67046617086457161, 13.01238886216411039, -1.492009926703888656 ) ) ;
#10299=CARTESIAN_POINT ( 'NONE',  ( -36.65473259702432074, 28.27472347546385834, 1.269999999999995577 ) ) ;
#10301=DIRECTION ( 'NONE',  ( 5.188838149069472160E-16, -1.699382548006136559E-16, -1.000000000000000000 ) ) ;
#10303=DIRECTION ( 'NONE',  ( -0.8745520943968235761, 0.4849315768086558398, -4.268512490100410909E-16 ) ) ;
#10306=LINE ( 'NONE', #10092, #1506 ) ;
#10307=CARTESIAN_POINT ( 'NONE',  ( -58.00234944525002589, 2.059104932340308114, 0.8980956459801138214 ) ) ;
#10308=CARTESIAN_POINT ( 'NONE',  ( -58.24807683554808335, 1.288543178753334573, 1.357556113208942428 ) ) ;
#10311=CARTESIAN_POINT ( 'NONE',  ( -57.76461416131697746, 2.594137363129217277, -1.330350326707380626 ) ) ;
#10313=EDGE_LOOP ( 'NONE', ( #24145, #3318, #36897, #11171, #18412 ) ) ;
#10322=CARTESIAN_POINT ( 'NONE',  ( -31.84560491834792373, 53.04492649710044816, 1.269999999999993578 ) ) ;
#10330=CARTESIAN_POINT ( 'NONE',  ( -57.60360693722056169, 1.361403835229456849, -1.300536957989121500 ) ) ;
#10347=CARTESIAN_POINT ( 'NONE',  ( -56.71132732703541990, 3.319205314284062958, -2.191228219141365230 ) ) ;
#10348=DIRECTION ( 'NONE',  ( -0.8745520943968126959, 0.4849315768086755463, -5.691349986800565628E-16 ) ) ;
#10350=CARTESIAN_POINT ( 'NONE',  ( -30.01829664378881901, 60.43850663962886216, -1.270000000000005569 ) ) ;
#10355=CARTESIAN_POINT ( 'NONE',  ( -41.62422838180499696, 22.52195256220245057, -1.324149224696933747 ) ) ;
#10363=CARTESIAN_POINT ( 'NONE',  ( -47.26619606798129070, 24.98193397792426751, -1.785901896324533222 ) ) ;
#10379=CARTESIAN_POINT ( 'NONE',  ( -57.02215525307828159, 2.672977372696112575, -2.026151568886790599 ) ) ;
#10380=DIRECTION ( 'NONE',  ( -0.8745520943968243532, 0.4849315768086547296, -5.361993529360573944E-16 ) ) ;
#10388=VECTOR ( 'NONE', #36781, 1000.000000000000114 ) ;
#10394=CIRCLE ( 'NONE', #40373, 0.5080000000000000071 ) ;
#10398=AXIS2_PLACEMENT_3D ( 'NONE', #4869, #32613, #4242 ) ;
#10400=CARTESIAN_POINT ( 'NONE',  ( -46.77033296427473630, 25.82163574504403059, 1.429790282917978939 ) ) ;
#10401=CARTESIAN_POINT ( 'NONE',  ( -48.75318004186330967, 22.89261100037833785, 1.301163434177643241 ) ) ;
#10403=CARTESIAN_POINT ( 'NONE',  ( -54.34142964503966056, 9.837102586603037935, 3.694930414371496052 ) ) ;
#10404=CARTESIAN_POINT ( 'NONE',  ( -58.63886446992002988, -0.3042812601921741078, 0.3526691660533222694 ) ) ;
#10407=ORIENTED_EDGE ( 'NONE', *, *, #3748, .T. ) ;
#10408=CARTESIAN_POINT ( 'NONE',  ( -44.36446822842629700, 21.81554158013422651, 2.896954608336737014 ) ) ;
#10411=VECTOR ( 'NONE', #38924, 1000.000000000000000 ) ;
#10414=AXIS2_PLACEMENT_3D ( 'NONE', #32006, #37982, #12207 ) ;
#10416=CARTESIAN_POINT ( 'NONE',  ( -5.924740142096584172, 65.21691166894066782, 1.270000000000006013 ) ) ;
#10423=EDGE_CURVE ( 'NONE', #915, #10519, #6577, .T. ) ;
#10426=CARTESIAN_POINT ( 'NONE',  ( -14.60888863026623952, 79.54114996201613508, 1.269999999999998019 ) ) ;
#10434=CARTESIAN_POINT ( 'NONE',  ( -47.44699234454015624, 15.94620872345377904, 0.4021177788561363098 ) ) ;
#10443=DIRECTION ( 'NONE',  ( 0.8745520943968243532, -0.4849315768086547296, 6.829619984160642269E-16 ) ) ;
#10467=CYLINDRICAL_SURFACE ( 'NONE', #40107, 0.6350000000000014522 ) ;
#10468=DIRECTION ( 'NONE',  ( -5.188838149069471174E-16, 1.699382548006136313E-16, 1.000000000000000000 ) ) ;
#10474=DIRECTION ( 'NONE',  ( -0.8745520943968235761, 0.4849315768086558398, -5.691349986800547879E-16 ) ) ;
#10476=DIRECTION ( 'NONE',  ( 0.9998501190848636533, 0.01731298258487296016, -2.441448296158449905E-15 ) ) ;
#10481=CARTESIAN_POINT ( 'NONE',  ( -58.64197075571546947, -0.3086314946795363223, -0.3446796491146816854 ) ) ;
#10483=DIRECTION ( 'NONE',  ( -0.4849315768086534528, -0.8745520943968249084, -1.030032898892974818E-16 ) ) ;
#10495=ORIENTED_EDGE ( 'NONE', *, *, #356, .T. ) ;
#10497=CARTESIAN_POINT ( 'NONE',  ( -14.42383115828894447, 69.61113539875873357, 1.524000000000000243 ) ) ;
#10498=CARTESIAN_POINT ( 'NONE',  ( -48.98643424071138952, 17.83616253325477174, 5.099923142907145213 ) ) ;
#10499=EDGE_CURVE ( 'NONE', #32297, #33608, #4656, .T. ) ;
#10503=AXIS2_PLACEMENT_3D ( 'NONE', #2983, #25340, #3186 ) ;
#10507=EDGE_CURVE ( 'NONE', #30484, #15671, #12016, .T. ) ;
#10508=CARTESIAN_POINT ( 'NONE',  ( -51.86985193027736329, 10.34936321858908492, -9.208787596046330052E-15 ) ) ;
#10510=CARTESIAN_POINT ( 'NONE',  ( -24.32950799593924884, 77.42192949967211746, -1.270000000000005569 ) ) ;
#10511=CARTESIAN_POINT ( 'NONE',  ( -46.91105319604628932, 25.30766295409365441, -1.767504291099697866 ) ) ;
#10512=DIRECTION ( 'NONE',  ( 5.188838149069472160E-16, -1.699382548006136559E-16, -1.000000000000000000 ) ) ;
#10513=CARTESIAN_POINT ( 'NONE',  ( -29.37490963521362275, 66.57792725179282911, -1.524000000000867994 ) ) ;
#10515=CARTESIAN_POINT ( 'NONE',  ( -46.87324200585490530, 25.14909121271579195, 1.861784591013474266 ) ) ;
#10516=CARTESIAN_POINT ( 'NONE',  ( -58.03112897257378933, 1.932186039288422030, 1.137512825365907254 ) ) ;
#10517=CARTESIAN_POINT ( 'NONE',  ( -55.60508136934060275, 7.116827924314645060, 3.170888472016278214 ) ) ;
#10519=VERTEX_POINT ( 'NONE', #28472 ) ;
#10520=CARTESIAN_POINT ( 'NONE',  ( -56.91719228404756592, 5.442273006173628858, -0.3640331681397807606 ) ) ;
#10522=ADVANCED_FACE ( 'NONE', ( #11645 ), #22888, .T. ) ;
#10524=PLANE ( 'NONE',  #15822 ) ;
#10530=EDGE_CURVE ( 'NONE', #27874, #25310, #5926, .T. ) ;
#10540=CARTESIAN_POINT ( 'NONE',  ( -58.16081875750722219, 0.1563330388574495078, -0.6246648654044505422 ) ) ;
#10546=CARTESIAN_POINT ( 'NONE',  ( -48.82738941085167284, 18.57305038084609095, -5.399437279161923620 ) ) ;
#10555=CARTESIAN_POINT ( 'NONE',  ( -49.72660956849071567, 16.83360665160238412, -5.072308565479707099 ) ) ;
#10562=EDGE_CURVE ( 'NONE', #12982, #1192, #39242, .T. ) ;
#10564=CARTESIAN_POINT ( 'NONE',  ( -7.772068811996249771, 69.25462295839062676, 1.524000000000003796 ) ) ;
#10568=ORIENTED_EDGE ( 'NONE', *, *, #15865, .F. ) ;
#10575=DIRECTION ( 'NONE',  ( -0.9807655518882848478, 0.1951894777626808908, -8.537024980200819846E-16 ) ) ;
#10577=EDGE_CURVE ( 'NONE', #26127, #14331, #2621, .T. ) ;
#10581=CARTESIAN_POINT ( 'NONE',  ( -18.88948446928058900, 80.17638627449419175, 1.269999999999995799 ) ) ;
#10582=FACE_OUTER_BOUND ( 'NONE', #7787, .T. ) ;
#10586=CARTESIAN_POINT ( 'NONE',  ( -58.76944392236582360, -0.3049061203676955989, -0.2000781065760083854 ) ) ;
#10587=CARTESIAN_POINT ( 'NONE',  ( -5.861642722916909243, 64.54502714855203749, -1.269999999999993801 ) ) ;
#10594=DIRECTION ( 'NONE',  ( -5.188838149069471174E-16, 1.699382548006136313E-16, 1.000000000000000000 ) ) ;
#10596=AXIS2_PLACEMENT_3D ( 'NONE', #34273, #11670, #14648 ) ;
#10599=DIRECTION ( 'NONE',  ( -5.188838149069471174E-16, 1.699382548006136313E-16, 1.000000000000000000 ) ) ;
#10607=CARTESIAN_POINT ( 'NONE',  ( -57.61251194202308312, 1.342215824410947222, 1.291938351770520077 ) ) ;
#10608=CARTESIAN_POINT ( 'NONE',  ( -48.74997074597248314, 21.16799237019927205, 3.036721307642054946 ) ) ;
#10610=CARTESIAN_POINT ( 'NONE',  ( -49.72660956849071567, 16.83360665160238412, 5.072308565479690223 ) ) ;
#10611=CARTESIAN_POINT ( 'NONE',  ( -58.19146433326328349, 0.6478084378821518108, 1.146157376894137325 ) ) ;
#10616=CARTESIAN_POINT ( 'NONE',  ( -41.05189575270516400, 23.09451173561986081, 1.523999999999992472 ) ) ;
#10623=AXIS2_PLACEMENT_3D ( 'NONE', #30431, #23175, #30224 ) ;
#10626=DIRECTION ( 'NONE',  ( -0.9336303900108815501, -0.3582377630124009560, -4.235673982319039874E-16 ) ) ;
#10627=CARTESIAN_POINT ( 'NONE',  ( -47.20932677516402975, 20.06242161047454076, 5.120036295479145849 ) ) ;
#10631=CIRCLE ( 'NONE', #23537, 0.2539999999999998925 ) ;
#10632=CARTESIAN_POINT ( 'NONE',  ( -17.14500000000466784, 71.11999999999886768, 1.269999999999998241 ) ) ;
#10634=DIRECTION ( 'NONE',  ( -5.188838149069471174E-16, 1.699382548006136313E-16, 1.000000000000000000 ) ) ;
#10640=ORIENTED_EDGE ( 'NONE', *, *, #38131, .F. ) ;
#10641=CARTESIAN_POINT ( 'NONE',  ( -53.75865956017525349, 9.373754164828760338, 3.697140908559925165 ) ) ;
#10646=ORIENTED_EDGE ( 'NONE', *, *, #36018, .T. ) ;
#10652=VERTEX_POINT ( 'NONE', #28042 ) ;
#10657=AXIS2_PLACEMENT_3D ( 'NONE', #5444, #5237, #18404 ) ;
#10662=CARTESIAN_POINT ( 'NONE',  ( -17.14500000000466784, 71.11999999999886768, -1.270000000000000684 ) ) ;
#10679=DIRECTION ( 'NONE',  ( 5.188838149069472160E-16, -1.699382548006136559E-16, -1.000000000000000000 ) ) ;
#10688=CIRCLE ( 'NONE', #33818, 9.048749999999998295 ) ;
#10692=CARTESIAN_POINT ( 'NONE',  ( -47.36402082484878662, 19.94680553081675356, 5.177108632069717942 ) ) ;
#10695=DIRECTION ( 'NONE',  ( -0.7284927773988482125, -0.6850534820564830873, 0.000000000000000000 ) ) ;
#10703=CARTESIAN_POINT ( 'NONE',  ( -58.36992421181236068, -0.2917964073288620286, -5.103743859794852046E-13 ) ) ;
#10711=TOROIDAL_SURFACE ( 'NONE', #40650, 8.794749999999998735, 0.2540000000000000036 ) ;
#10712=CARTESIAN_POINT ( 'NONE',  ( -54.07635852566403400, 7.689673991023174615, -1.154061576158815550 ) ) ;
#10714=CARTESIAN_POINT ( 'NONE',  ( -17.32429653712378936, 61.56493206124108042, -1.269999999999999130 ) ) ;
#10715=DIRECTION ( 'NONE',  ( 0.01731298258488772612, -0.9998501190848633202, 1.788962107505314604E-16 ) ) ;
#10716=CARTESIAN_POINT ( 'NONE',  ( -32.57812072184745489, 51.47121137486388420, -1.270000000000005569 ) ) ;
#10718=CARTESIAN_POINT ( 'NONE',  ( -46.38316532014830074, 26.05065462784526176, 1.523999999999997357 ) ) ;
#10720=CARTESIAN_POINT ( 'NONE',  ( -58.05887703936295452, 1.806656698574160558, 1.362798277128383972 ) ) ;
#10722=LINE ( 'NONE', #11144, #24024 ) ;
#10725=CARTESIAN_POINT ( 'NONE',  ( -55.80532936045926107, 9.325833942460080905, -1.087685647686953452E-14 ) ) ;
#10734=CARTESIAN_POINT ( 'NONE',  ( -8.473844426907703564, 67.77203500197072117, 1.524000000000003574 ) ) ;
#10738=CARTESIAN_POINT ( 'NONE',  ( -15.71196903609989981, 80.05455644220629097, 1.269999999999997575 ) ) ;
#10744=CARTESIAN_POINT ( 'NONE',  ( -57.61623536216810493, 1.334194615165582576, -1.288300599212580888 ) ) ;
#10749=CARTESIAN_POINT ( 'NONE',  ( -44.96292901393739072, 21.56701576681934540, -3.486870777078513228 ) ) ;
#10753=ORIENTED_EDGE ( 'NONE', *, *, #39902, .F. ) ;
#10756=DIRECTION ( 'NONE',  ( 0.8745520943968235761, -0.4849315768086558398, 0.000000000000000000 ) ) ;
#10758=EDGE_CURVE ( 'NONE', #13951, #22153, #41478, .T. ) ;
#10759=CARTESIAN_POINT ( 'NONE',  ( -53.45432727069204759, 10.77832982246877691, -4.078803160923793136 ) ) ;
#10763=EDGE_CURVE ( 'NONE', #22953, #14753, #31763, .T. ) ;
#10770=CARTESIAN_POINT ( 'NONE',  ( -17.09258512000246100, 84.17916046765628835, 1.523999999999996469 ) ) ;
#10774=CARTESIAN_POINT ( 'NONE',  ( -46.60530155212499892, 26.17382724835484709, -0.6632222222222314834 ) ) ;
#10777=DIRECTION ( 'NONE',  ( 5.188838149069472160E-16, -1.699382548006136559E-16, -1.000000000000000000 ) ) ;
#10780=VECTOR ( 'NONE', #26225, 1000.000000000000000 ) ;
#10782=CARTESIAN_POINT ( 'NONE',  ( -41.08173151913482002, 23.06272320883524785, 1.524000000019140932 ) ) ;
#10788=DIRECTION ( 'NONE',  ( -5.188838149069472160E-16, 1.699382548006136559E-16, 1.000000000000000000 ) ) ;
#10794=CARTESIAN_POINT ( 'NONE',  ( -55.40724689661794855, 6.067898552060245088, -3.000206617153963418 ) ) ;
#10802=CIRCLE ( 'NONE', #41413, 9.048749999999998295 ) ;
#10807=EDGE_LOOP ( 'NONE', ( #32374, #9668 ) ) ;
#10809=CARTESIAN_POINT ( 'NONE',  ( -29.89586364642803318, 71.55302121702176521, -1.524000000000007571 ) ) ;
#10810=CARTESIAN_POINT ( 'NONE',  ( -30.02342128825639023, 69.55262966049605211, -1.270000000000007123 ) ) ;
#10817=CARTESIAN_POINT ( 'NONE',  ( -16.46263872254443683, 83.91929436251373886, 1.269999999999996687 ) ) ;
#10818=CARTESIAN_POINT ( 'NONE',  ( -53.56064905838539403, 9.687610447046496986, 3.641404713838447105 ) ) ;
#10819=CARTESIAN_POINT ( 'NONE',  ( -49.15418727280429323, 24.05022843951647715, -9.137385882761073034E-15 ) ) ;
#10820=CARTESIAN_POINT ( 'NONE',  ( -50.29507671575587580, 15.72791930032350827, 4.796563717952097683 ) ) ;
#10821=CARTESIAN_POINT ( 'NONE',  ( -58.65389498535380852, -0.3158197163193834367, 0.3266806156710039266 ) ) ;
#10823=DIRECTION ( 'NONE',  ( -5.188838149069472160E-16, 1.699382548006136559E-16, 1.000000000000000000 ) ) ;
#10825=CARTESIAN_POINT ( 'NONE',  ( -45.82931853585290582, 22.14969803457954356, 3.600065900675641029 ) ) ;
#10826=AXIS2_PLACEMENT_3D ( 'NONE', #30070, #41656, #33277 ) ;
#10835=DIRECTION ( 'NONE',  ( -0.8745520943968245753, 0.4849315768086539524, -5.691349986800526185E-16 ) ) ;
#10836=CARTESIAN_POINT ( 'NONE',  ( -46.53702275532343435, 20.69065974945542763, 4.840627275220680481 ) ) ;
#10837=CARTESIAN_POINT ( 'NONE',  ( -25.80936006922821591, 73.72935646344811289, 1.269999999999992468 ) ) ;
#10839=DIRECTION ( 'NONE',  ( -0.8745520943968250194, 0.4849315768086532863, -5.361993529360574930E-16 ) ) ;
#10847=EDGE_LOOP ( 'NONE', ( #28065, #40856, #9196, #9902 ) ) ;
#10848=CARTESIAN_POINT ( 'NONE',  ( -49.86808358410245745, 14.13890166617936472, 1.547476669397152671 ) ) ;
#10857=CYLINDRICAL_SURFACE ( 'NONE', #14979, 0.2540000000000015024 ) ;
#10859=AXIS2_PLACEMENT_3D ( 'NONE', #18341, #22155, #2401 ) ;
#10867=FACE_OUTER_BOUND ( 'NONE', #35013, .T. ) ;
#10869=DIRECTION ( 'NONE',  ( 0.3582377630124009560, -0.9336303900108815501, 3.445432962228709470E-16 ) ) ;
#10874=ORIENTED_EDGE ( 'NONE', *, *, #34502, .F. ) ;
#10890=ORIENTED_EDGE ( 'NONE', *, *, #31808, .T. ) ;
#10891=CYLINDRICAL_SURFACE ( 'NONE', #216, 0.2540000000000005032 ) ;
#10902=DIRECTION ( 'NONE',  ( 5.188838149069472160E-16, -1.699382548006136559E-16, -1.000000000000000000 ) ) ;
#10903=AXIS2_PLACEMENT_3D ( 'NONE', #36480, #23668, #16870 ) ;
#10908=AXIS2_PLACEMENT_3D ( 'NONE', #39481, #39697, #33092 ) ;
#10910=CARTESIAN_POINT ( 'NONE',  ( -58.36222274556690337, -0.2757005147488722496, 0.1096927518865258300 ) ) ;
#10916=VECTOR ( 'NONE', #36355, 1000.000000000000114 ) ;
#10919=DIRECTION ( 'NONE',  ( 0.9469626219732538708, 0.3213437296502617002, 6.686393187109395313E-16 ) ) ;
#10920=CARTESIAN_POINT ( 'NONE',  ( -56.42856387642236626, 3.193865871111118082, -0.1553879740656047281 ) ) ;
#10922=DIRECTION ( 'NONE',  ( -0.8745520943968240202, 0.4849315768086553402, -5.361993529360572958E-16 ) ) ;
#10925=CARTESIAN_POINT ( 'NONE',  ( -29.18709815851897815, 67.04824513550720155, -1.524000000000006461 ) ) ;
#10930=CARTESIAN_POINT ( 'NONE',  ( -58.10740272659374739, 1.828491270143103975, 0.5949618876680204949 ) ) ;
#10931=DIRECTION ( 'NONE',  ( -5.188838149069471174E-16, 1.699382548006136313E-16, 1.000000000000000000 ) ) ;
#10934=CARTESIAN_POINT ( 'NONE',  ( -58.19197273006702886, 1.486408586729007109, -1.232490673556632332 ) ) ;
#10937=CARTESIAN_POINT ( 'NONE',  ( -47.60342124590309254, 19.66962190513607212, -5.193532021806997356 ) ) ;
#10938=AXIS2_PLACEMENT_3D ( 'NONE', #31718, #21475, #8931 ) ;
#10944=DIRECTION ( 'NONE',  ( 5.188838149069472160E-16, -1.699382548006136559E-16, -1.000000000000000000 ) ) ;
#10946=CARTESIAN_POINT ( 'NONE',  ( -52.88939467130921912, 11.33278677544117841, -4.135169601362077785 ) ) ;
#10947=DIRECTION ( 'NONE',  ( -0.8745520943968236871, 0.4849315768086558953, -5.361993529360571971E-16 ) ) ;
#10951=CARTESIAN_POINT ( 'NONE',  ( -58.19487492224605774, 0.08271841185791539708, -0.5637723373511558389 ) ) ;
#10952=EDGE_CURVE ( 'NONE', #4427, #29032, #31786, .T. ) ;
#10956=CARTESIAN_POINT ( 'NONE',  ( -46.30033180095409051, 21.65562830348028456, -4.292083522273610008 ) ) ;
#10968=CARTESIAN_POINT ( 'NONE',  ( -50.36516092884956208, 15.79195539882771726, -4.916963016749614113 ) ) ;
#10972=DIRECTION ( 'NONE',  ( 0.8745520943968235761, -0.4849315768086558398, 4.268512490100410909E-16 ) ) ;
#10980=TOROIDAL_SURFACE ( 'NONE', #36849, 0.7620000000000000107, 0.2540000000000000036 ) ;
#10982=CARTESIAN_POINT ( 'NONE',  ( -57.65203525413342334, 1.118929822212927361, 0.5921937322712250706 ) ) ;
#10984=ORIENTED_EDGE ( 'NONE', *, *, #5353, .F. ) ;
#10986=CARTESIAN_POINT ( 'NONE',  ( -47.01877684503696742, 24.36789988528162354, -2.430126310640470688 ) ) ;
#10988=CARTESIAN_POINT ( 'NONE',  ( -47.10086694478710712, 25.28009754960136490, -1.863548351662550617 ) ) ;
#10989=ORIENTED_EDGE ( 'NONE', *, *, #28206, .F. ) ;
#10993=CIRCLE ( 'NONE', #140, 2.857500000000000817 ) ;
#11002=AXIS2_PLACEMENT_3D ( 'NONE', #40725, #24506, #21512 ) ;
#11004=DIRECTION ( 'NONE',  ( -5.188838149069471174E-16, 1.699382548006136313E-16, 1.000000000000000000 ) ) ;
#11005=VERTEX_POINT ( 'NONE', #22062 ) ;
#11009=CARTESIAN_POINT ( 'NONE',  ( -48.44329217233745055, 18.62907245612683838, -5.187175938578627132 ) ) ;
#11017=CARTESIAN_POINT ( 'NONE',  ( -47.84356795211458291, 19.38525671449504983, 5.197506975155153697 ) ) ;
#11019=ORIENTED_EDGE ( 'NONE', *, *, #6783, .T. ) ;
#11021=LINE ( 'NONE', #27005, #14740 ) ;
#11023=AXIS2_PLACEMENT_3D ( 'NONE', #2208, #12616, #8799 ) ;
#11030=DIRECTION ( 'NONE',  ( 5.188838149069472160E-16, -1.699382548006136559E-16, -1.000000000000000000 ) ) ;
#11031=CARTESIAN_POINT ( 'NONE',  ( -54.64736747358799818, 7.536306771770948210, 3.171698711319464792 ) ) ;
#11032=CARTESIAN_POINT ( 'NONE',  ( -29.79391970787719757, 57.88946435418900194, -1.524000000000005128 ) ) ;
#11033=CARTESIAN_POINT ( 'NONE',  ( -57.93941708942283952, 2.052042089854988483, 1.628789306319508245 ) ) ;
#11034=CARTESIAN_POINT ( 'NONE',  ( -57.69320192990073082, 1.722488987974756025, 1.652538576205534460 ) ) ;
#11038=CARTESIAN_POINT ( 'NONE',  ( -44.55074271434504851, 21.27721161058206789, 3.389857510897057224 ) ) ;
#11043=SURFACE_STYLE_FILL_AREA ( #4469 ) ;
#11045=ORIENTED_EDGE ( 'NONE', *, *, #40493, .F. ) ;
#11049=CARTESIAN_POINT ( 'NONE',  ( -45.65533061069353238, 20.86966646997320396, 4.138311239626682791 ) ) ;
#11052=EDGE_CURVE ( 'NONE', #30132, #30491, #37901, .T. ) ;
#11053=LINE ( 'NONE', #13830, #34757 ) ;
#11055=LINE ( 'NONE', #4688, #40280 ) ;
#11065=CARTESIAN_POINT ( 'NONE',  ( -49.09053848811835508, 14.44377425990215436, 0.7907028275641450055 ) ) ;
#11075=EDGE_LOOP ( 'NONE', ( #12438, #3792, #18892, #31958 ) ) ;
#11081=DIRECTION ( 'NONE',  ( -5.188838149069471174E-16, 1.699382548006136313E-16, 1.000000000000000000 ) ) ;
#11084=CARTESIAN_POINT ( 'NONE',  ( -11.05715273818225164, 82.67346420587206524, -1.269999999999999352 ) ) ;
#11087=EDGE_LOOP ( 'NONE', ( #32434, #28676, #17887, #386 ) ) ;
#11091=CARTESIAN_POINT ( 'NONE',  ( -5.885917553499150578, 77.12042444889114279, -1.523999999999996025 ) ) ;
#11094=AXIS2_PLACEMENT_3D ( 'NONE', #23371, #11030, #39813 ) ;
#11096=CYLINDRICAL_SURFACE ( 'NONE', #6113, 0.2539999999999998925 ) ;
#11101=CARTESIAN_POINT ( 'NONE',  ( -25.77058783747419213, 72.83664265955201245, -1.524000000000005572 ) ) ;
#11102=ORIENTED_EDGE ( 'NONE', *, *, #34542, .F. ) ;
#11106=EDGE_CURVE ( 'NONE', #39412, #41136, #23320, .T. ) ;
#11110=LINE ( 'NONE', #4328, #38123 ) ;
#11113=CARTESIAN_POINT ( 'NONE',  ( -41.80860202649011370, 22.71167205159044045, 1.570694036847530173 ) ) ;
#11119=CIRCLE ( 'NONE', #26788, 0.7620000000000015650 ) ;
#11125=CARTESIAN_POINT ( 'NONE',  ( -50.47813777548210368, 15.38220854283604133, 4.696510882197381775 ) ) ;
#11133=CARTESIAN_POINT ( 'NONE',  ( -55.72901529264892417, 4.991126730481368234, -1.691135755076719649 ) ) ;
#11136=CIRCLE ( 'NONE', #39709, 9.048749999999998295 ) ;
#11139=DIRECTION ( 'NONE',  ( 0.1906721105965065721, -0.9816537812491090698, 2.657572025465716008E-16 ) ) ;
#11142=DIRECTION ( 'NONE',  ( -0.8745520943968240202, 0.4849315768086551737, -5.361993529360572958E-16 ) ) ;
#11143=CARTESIAN_POINT ( 'NONE',  ( -58.32144855246983184, 1.173557705256414341, 1.098103182355992136 ) ) ;
#11144=CARTESIAN_POINT ( 'NONE',  ( -3.831877602099685198, 71.07198261757335445, -1.523999999999993804 ) ) ;
#11146=AXIS2_PLACEMENT_3D ( 'NONE', #13915, #23269, #23481 ) ;
#11147=ORIENTED_EDGE ( 'NONE', *, *, #25126, .T. ) ;
#11148=CARTESIAN_POINT ( 'NONE',  ( -56.26154134543016738, 7.775270144418325202, -0.1976385065555597287 ) ) ;
#11150=CARTESIAN_POINT ( 'NONE',  ( -45.11690586071466669, 21.31720619196558886, -3.746636771225956952 ) ) ;
#11154=CIRCLE ( 'NONE', #30883, 0.5080000000000000071 ) ;
#11157=DIRECTION ( 'NONE',  ( -5.188838149069472160E-16, 1.699382548006136559E-16, 1.000000000000000000 ) ) ;
#11159=CARTESIAN_POINT ( 'NONE',  ( -49.26965912534817704, 17.43349283265777672, -5.070912566603587024 ) ) ;
#11163=CARTESIAN_POINT ( 'NONE',  ( -57.79663075882820777, 0.9446393961914554271, -1.102772590789307339 ) ) ;
#11165=CIRCLE ( 'NONE', #7780, 0.2539999999999998925 ) ;
#11168=CARTESIAN_POINT ( 'NONE',  ( -46.25688858429101202, 20.73875112231587892, -4.700046123029353318 ) ) ;
#11171=ORIENTED_EDGE ( 'NONE', *, *, #39593, .T. ) ;
#11176=CARTESIAN_POINT ( 'NONE',  ( -52.26939619200407350, 13.58078015197115818, -4.476849201000089096 ) ) ;
#11177=DIRECTION ( 'NONE',  ( -5.188838149069472160E-16, 1.699382548006136559E-16, 1.000000000000000000 ) ) ;
#11184=CARTESIAN_POINT ( 'NONE',  ( -8.095114962461808616, 74.19100168833409725, -1.269999999999996687 ) ) ;
#11185=CARTESIAN_POINT ( 'NONE',  ( -13.15921246430372804, 51.38419125632634632, 1.524000000000004018 ) ) ;
#11187=CARTESIAN_POINT ( 'NONE',  ( -58.24002838079472610, 0.001074765447070524793, 0.6562585879479658768 ) ) ;
#11190=CARTESIAN_POINT ( 'NONE',  ( -46.60530155212503445, 26.17382724835477958, -9.383119846931408523E-15 ) ) ;
#11192=CARTESIAN_POINT ( 'NONE',  ( -47.00737061382944404, 25.44871393995562769, -1.744193148937779769 ) ) ;
#11202=ORIENTED_EDGE ( 'NONE', *, *, #11560, .T. ) ;
#11206=CARTESIAN_POINT ( 'NONE',  ( -41.05189575270516400, 23.09451173561988213, 0.7619999999999945706 ) ) ;
#11213=CARTESIAN_POINT ( 'NONE',  ( -54.14414085402640353, 8.624088997047390848, -3.578441826534806580 ) ) ;
#11218=EDGE_LOOP ( 'NONE', ( #25499, #39290, #6875, #28888 ) ) ;
#11221=DIRECTION ( 'NONE',  ( -0.8745520943968281280, 0.4849315768086481238, 5.653143757709536353E-15 ) ) ;
#11226=CARTESIAN_POINT ( 'NONE',  ( -29.73153358407946101, 68.50109170616188692, -1.270000000000007123 ) ) ;
#11229=ADVANCED_FACE ( 'NONE', ( #26753 ), #367, .T. ) ;
#11232=AXIS2_PLACEMENT_3D ( 'NONE', #24220, #31243, #37231 ) ;
#11235=CARTESIAN_POINT ( 'NONE',  ( -57.28641868539627779, 2.042781982619619630, 1.582485259194238658 ) ) ;
#11237=CARTESIAN_POINT ( 'NONE',  ( -58.50860430493789721, 0.7049166599848305514, 0.9756837515128383709 ) ) ;
#11238=CARTESIAN_POINT ( 'NONE',  ( -58.20197065718431162, 0.6251715515077186369, 1.133219051752172080 ) ) ;
#11243=CARTESIAN_POINT ( 'NONE',  ( -49.56090548067184898, 17.87959676410238430, 5.165259844110607013 ) ) ;
#11249=LINE ( 'NONE', #28280, #824 ) ;
#11251=ORIENTED_EDGE ( 'NONE', *, *, #15470, .F. ) ;
#11254=CARTESIAN_POINT ( 'NONE',  ( -41.05189575270519242, 23.09451173561980042, -1.270000000000005125 ) ) ;
#11255=CARTESIAN_POINT ( 'NONE',  ( -46.36020037345180356, 20.58642004075764476, 4.649377256144936688 ) ) ;
#11258=CARTESIAN_POINT ( 'NONE',  ( -33.20758249455312239, 49.81222039523557044, -1.524000000000005572 ) ) ;
#11267=VERTEX_POINT ( 'NONE', #575 ) ;
#11269=CARTESIAN_POINT ( 'NONE',  ( -52.42931032121356338, 11.92852722686772005, 4.179465640474072430 ) ) ;
#11271=AXIS2_PLACEMENT_3D ( 'NONE', #20828, #27033, #10835 ) ;
#11285=DIRECTION ( 'NONE',  ( -0.9469626219732555361, -0.3213437296502561491, -8.537024980200885913E-16 ) ) ;
#11289=ADVANCED_FACE ( 'NONE', ( #32943 ), #36556, .F. ) ;
#11292=LINE ( 'NONE', #37281, #3546 ) ;
#11313=ORIENTED_EDGE ( 'NONE', *, *, #41740, .F. ) ;
#11315=CARTESIAN_POINT ( 'NONE',  ( -3.831877602099685198, 71.07198261757335445, -1.523999999999993804 ) ) ;
#11317=( NAMED_UNIT ( * ) PLANE_ANGLE_UNIT ( ) SI_UNIT ( $, .RADIAN. ) );
#11324=VERTEX_POINT ( 'NONE', #23956 ) ;
#11325=CIRCLE ( 'NONE', #10623, 0.2540000000000025016 ) ;
#11328=EDGE_CURVE ( 'NONE', #32447, #17471, #26022, .T. ) ;
#11329=VECTOR ( 'NONE', #789, 1000.000000000000114 ) ;
#11333=CARTESIAN_POINT ( 'NONE',  ( -54.56827866224503509, 7.775013980772373934, 3.396949012664772560 ) ) ;
#11339=EDGE_CURVE ( 'NONE', #35679, #14172, #15801, .T. ) ;
#11343=EDGE_CURVE ( 'NONE', #34378, #11774, #31463, .T. ) ;
#11344=CARTESIAN_POINT ( 'NONE',  ( -56.89722832398061314, 2.603431824206650536, -0.9028745487782567913 ) ) ;
#11346=AXIS2_PLACEMENT_3D ( 'NONE', #9547, #23145, #35333 ) ;
#11351=CARTESIAN_POINT ( 'NONE',  ( -46.73713699923415277, 25.40205342722763859, 1.701536002565660510 ) ) ;
#11352=CARTESIAN_POINT ( 'NONE',  ( -7.842268484490568348, 73.30875693322846587, 1.270000000000002904 ) ) ;
#11353=DIRECTION ( 'NONE',  ( -0.4849315768086534528, -0.8745520943968250194, -1.030032898892974942E-16 ) ) ;
#11354=CARTESIAN_POINT ( 'NONE',  ( -58.37241122568488549, -0.2962816677227753104, 0.2416009568453807987 ) ) ;
#11356=AXIS2_PLACEMENT_3D ( 'NONE', #736, #11139, #24125 ) ;
#11358=DIRECTION ( 'NONE',  ( 0.5149185422762221354, -0.8572391118119440101, 4.128606161907601007E-16 ) ) ;
#11360=CARTESIAN_POINT ( 'NONE',  ( -44.00561601145676605, 21.61144970255528008, -2.814601217460917404 ) ) ;
#11367=CARTESIAN_POINT ( 'NONE',  ( -51.02349128109572263, 14.61359224283002511, -4.685075518275549911 ) ) ;
#11371=CARTESIAN_POINT ( 'NONE',  ( -52.16429070073207441, 12.35296858188530145, -4.167432729078118570 ) ) ;
#11374=CARTESIAN_POINT ( 'NONE',  ( -47.67648637180143822, 19.71513033058998232, -5.327979952964785326 ) ) ;
#11380=CARTESIAN_POINT ( 'NONE',  ( -58.83227707057486811, -0.08366279997995551554, -1.273395421382134774E-15 ) ) ;
#11381=CIRCLE ( 'NONE', #38616, 0.5080000000000014504 ) ;
#11385=EDGE_CURVE ( 'NONE', #4082, #14480, #21901, .T. ) ;
#11387=EDGE_CURVE ( 'NONE', #36274, #35500, #40315, .T. ) ;
#11394=TOROIDAL_SURFACE ( 'NONE', #41340, 0.7620000000000000107, 0.2540000000000000036 ) ;
#11395=CARTESIAN_POINT ( 'NONE',  ( -58.37241122568488549, -0.2962816677227753104, -1.039428729632917149E-14 ) ) ;
#11397=VERTEX_POINT ( 'NONE', #33986 ) ;
#11398=CARTESIAN_POINT ( 'NONE',  ( -48.57235503434458224, 24.64055110436136431, -0.2038152558995032504 ) ) ;
#11412=CARTESIAN_POINT ( 'NONE',  ( -46.58415285064482703, 20.65776990352928877, -4.869103069372410886 ) ) ;
#11415=ORIENTED_EDGE ( 'NONE', *, *, #11052, .T. ) ;
#11419=CARTESIAN_POINT ( 'NONE',  ( -58.34556966141492040, -0.2407783058112067387, -0.1938516799453308959 ) ) ;
#11430=CARTESIAN_POINT ( 'NONE',  ( -4.095482865093060809, 71.62450171983788039, 1.270000000000005347 ) ) ;
#11431=CARTESIAN_POINT ( 'NONE',  ( -7.961576494521614755, 72.55615504727386167, -1.523999999999996247 ) ) ;
#11437=DIRECTION ( 'NONE',  ( -0.8745520943968423389, 0.4849315768086222556, -5.691349986800581405E-16 ) ) ;
#11438=CARTESIAN_POINT ( 'NONE',  ( -57.88388651883108338, 0.7560526178991631152, 1.004446660134626912 ) ) ;
#11440=CARTESIAN_POINT ( 'NONE',  ( -52.50609217148328867, 12.02659833652626808, 4.260190243505617147 ) ) ;
#11445=CARTESIAN_POINT ( 'NONE',  ( -52.42133349025997546, 11.92692459785933679, 4.172736198742178715 ) ) ;
#11454=FACE_OUTER_BOUND ( 'NONE', #11520, .T. ) ;
#11455=CARTESIAN_POINT ( 'NONE',  ( -43.90699889932533040, 21.43881162649801908, 2.872437248226452411 ) ) ;
#11456=CARTESIAN_POINT ( 'NONE',  ( -20.79116009376201646, 79.67004825550966984, -1.524000000000004018 ) ) ;
#11459=DIRECTION ( 'NONE',  ( 0.3256999990547897461, 0.9454731675810318370, 0.000000000000000000 ) ) ;
#11470=CARTESIAN_POINT ( 'NONE',  ( -50.29507671575589001, 15.72791930032348873, 4.796563717952099459 ) ) ;
#11474=VERTEX_POINT ( 'NONE', #30566 ) ;
#11476=ORIENTED_EDGE ( 'NONE', *, *, #5278, .T. ) ;
#11481=ORIENTED_EDGE ( 'NONE', *, *, #5292, .T. ) ;
#11487=DIRECTION ( 'NONE',  ( -0.8745520943968245753, 0.4849315768086539524, -5.691349986800526185E-16 ) ) ;
#11489=AXIS2_PLACEMENT_3D ( 'NONE', #21235, #5093, #9317 ) ;
#11490=DIRECTION ( 'NONE',  ( 0.1906721105964953034, -0.9816537812491112902, 0.000000000000000000 ) ) ;
#11498=DIRECTION ( 'NONE',  ( -0.9454731675810338354, 0.3256999990547844170, -5.459396135145338185E-16 ) ) ;
#11505=CARTESIAN_POINT ( 'NONE',  ( -58.20820809768405013, 1.420579653404072218, 1.355822160094593887 ) ) ;
#11510=ADVANCED_FACE ( 'NONE', ( #2245 ), #18392, .T. ) ;
#11520=EDGE_LOOP ( 'NONE', ( #28821, #1136, #18908, #37271 ) ) ;
#11532=CARTESIAN_POINT ( 'NONE',  ( -5.924740142096584172, 65.21691166894066782, 1.270000000000005125 ) ) ;
#11539=CARTESIAN_POINT ( 'NONE',  ( -50.55264109715174214, 15.40887103991305018, 4.805487048261737115 ) ) ;
#11546=CIRCLE ( 'NONE', #33309, 0.3810000000000000053 ) ;
#11548=CARTESIAN_POINT ( 'NONE',  ( -57.22211421646271390, 1.778355698664496609, -0.1074917508089587859 ) ) ;
#11557=DIRECTION ( 'NONE',  ( 5.188838149069472160E-16, -1.699382548006136559E-16, -1.000000000000000000 ) ) ;
#11560=EDGE_CURVE ( 'NONE', #24684, #26813, #4949, .T. ) ;
#11561=ORIENTED_EDGE ( 'NONE', *, *, #22948, .T. ) ;
#11562=CARTESIAN_POINT ( 'NONE',  ( -58.79341205368594814, 0.01963237121659078266, -0.1476394306258474176 ) ) ;
#11563=EDGE_CURVE ( 'NONE', #5054, #36653, #37579, .T. ) ;
#11565=CARTESIAN_POINT ( 'NONE',  ( -43.98070909378276383, 21.30087824701856647, -2.736222515986692194 ) ) ;
#11572=CARTESIAN_POINT ( 'NONE',  ( -52.37404615337990776, 12.26367279239957320, -4.302067587320100195 ) ) ;
#11575=FACE_OUTER_BOUND ( 'NONE', #33594, .T. ) ;
#11577=CARTESIAN_POINT ( 'NONE',  ( -51.57356029563064226, 13.43704833176837354, -4.363522926272087155 ) ) ;
#11581=CARTESIAN_POINT ( 'NONE',  ( -52.42133349025997546, 11.92692459785933679, -4.172736198742198255 ) ) ;
#11588=ADVANCED_FACE ( 'NONE', ( #25010 ), #19028, .T. ) ;
#11590=CARTESIAN_POINT ( 'NONE',  ( -57.80205714066466527, 2.371715784325115095, -1.753227392946310470 ) ) ;
#11593=DIRECTION ( 'NONE',  ( -0.9454731675810332803, 0.3256999990547855828, -8.537024980200802097E-16 ) ) ;
#11594=AXIS2_PLACEMENT_3D ( 'NONE', #3589, #26351, #26566 ) ;
#11597=CARTESIAN_POINT ( 'NONE',  ( -54.98111839650035648, 8.542840639972862249, -3.427624633821342304 ) ) ;
#11598=CARTESIAN_POINT ( 'NONE',  ( -41.05189575270519242, 23.09451173561983950, -0.4656666666666720023 ) ) ;
#11601=CIRCLE ( 'NONE', #35395, 0.2539999999999937863 ) ;
#11603=CARTESIAN_POINT ( 'NONE',  ( -58.29601494275114959, -0.1585044380288253008, 0.03613930236862695350 ) ) ;
#11604=CARTESIAN_POINT ( 'NONE',  ( -49.59816314059868603, 17.91649583374772092, 5.069000701391646935 ) ) ;
#11606=ORIENTED_EDGE ( 'NONE', *, *, #28977, .F. ) ;
#11607=CARTESIAN_POINT ( 'NONE',  ( -48.00704091872448487, 20.04541143072568232, -5.176114466449832641 ) ) ;
#11621=FACE_OUTER_BOUND ( 'NONE', #31979, .T. ) ;
#11627=CARTESIAN_POINT ( 'NONE',  ( -58.44555280191370628, -0.4200408777308817232, -0.3231375529350146159 ) ) ;
#11635=ORIENTED_EDGE ( 'NONE', *, *, #36593, .F. ) ;
#11640=DIRECTION ( 'NONE',  ( 6.829619984160660610E-15, 0.000000000000000000, 1.000000000000000000 ) ) ;
#11645=FACE_OUTER_BOUND ( 'NONE', #1681, .T. ) ;
#11653=CARTESIAN_POINT ( 'NONE',  ( -58.01159622203579858, 0.4793617641021541420, 0.8436046718122062194 ) ) ;
#11654=CARTESIAN_POINT ( 'NONE',  ( -29.63955833213042013, 69.20431239923942712, -1.524000000000007127 ) ) ;
#11660=CARTESIAN_POINT ( 'NONE',  ( -48.38589991294942649, 19.15920805527091630, 5.452675306770309760 ) ) ;
#11670=DIRECTION ( 'NONE',  ( -5.188838149069472160E-16, 1.699382548006136559E-16, 1.000000000000000000 ) ) ;
#11671=CARTESIAN_POINT ( 'NONE',  ( -41.09670346151852982, 23.04688172093030474, 1.270085369932500763 ) ) ;
#11672=LINE ( 'NONE', #11456, #35815 ) ;
#11680=AXIS2_PLACEMENT_3D ( 'NONE', #33742, #4566, #20926 ) ;
#11686=CARTESIAN_POINT ( 'NONE',  ( -54.82379132704179625, 7.242239488055856711, 3.238872252923468587 ) ) ;
#11690=ORIENTED_EDGE ( 'NONE', *, *, #19395, .F. ) ;
#11699=CYLINDRICAL_SURFACE ( 'NONE', #9515, 0.2540000000000015024 ) ;
#11711=DIRECTION ( 'NONE',  ( 0.3256999990547897461, 0.9454731675810318370, 0.000000000000000000 ) ) ;
#11716=CARTESIAN_POINT ( 'NONE',  ( -23.69188486464780752, 78.08202335040543574, 1.269999999999993801 ) ) ;
#11720=CYLINDRICAL_SURFACE ( 'NONE', #8805, 0.6350000000000014522 ) ;
#11743=CARTESIAN_POINT ( 'NONE',  ( -17.09258512000246455, 84.17916046765628835, 1.269999999999996243 ) ) ;
#11753=TOROIDAL_SURFACE ( 'NONE', #27382, 0.7620000000000000107, 0.2540000000000000036 ) ;
#11754=CARTESIAN_POINT ( 'NONE',  ( -58.41956937744257061, -0.3672969284060638717, 0.3776070891698000143 ) ) ;
#11762=ADVANCED_FACE ( 'NONE', ( #41853 ), #19242, .F. ) ;
#11764=CARTESIAN_POINT ( 'NONE',  ( -57.34787435976329562, 1.552391619547732748, -0.09937746155961837968 ) ) ;
#11771=CARTESIAN_POINT ( 'NONE',  ( -29.94429436251954613, 71.80236127745905605, -1.270000000000007345 ) ) ;
#11774=VERTEX_POINT ( 'NONE', #25223 ) ;
#11775=CARTESIAN_POINT ( 'NONE',  ( -58.69054519303719530, 0.2722345423086247607, -0.6021937201626393898 ) ) ;
#11776=VERTEX_POINT ( 'NONE', #31826 ) ;
#11778=CIRCLE ( 'NONE', #30812, 0.2539999999999989488 ) ;
#11785=CARTESIAN_POINT ( 'NONE',  ( -51.00929282542724508, 14.63754895018605140, -4.688694305049216915 ) ) ;
#11786=ORIENTED_EDGE ( 'NONE', *, *, #18115, .T. ) ;
#11788=CARTESIAN_POINT ( 'NONE',  ( -10.18297664959815663, 77.66688486464208552, 1.270000000000000906 ) ) ;
#11790=CARTESIAN_POINT ( 'NONE',  ( -56.17496734581288109, 4.395220231953922863, -2.356759703232587100 ) ) ;
#11793=CARTESIAN_POINT ( 'NONE',  ( -56.78650302187183740, 3.241477563879227475, -2.205756828360271093 ) ) ;
#11795=EDGE_CURVE ( 'NONE', #30484, #39372, #34862, .T. ) ;
#11797=EDGE_LOOP ( 'NONE', ( #35754, #14813, #3615, #15345 ) ) ;
#11802=CARTESIAN_POINT ( 'NONE',  ( -58.20820809768403592, 1.420579653404085985, -1.355822160094614759 ) ) ;
#11805=ADVANCED_FACE ( 'NONE', ( #26053 ), #23925, .T. ) ;
#11812=CARTESIAN_POINT ( 'NONE',  ( -42.83068693079387401, 21.70476352389080787, -1.889833665869970369 ) ) ;
#11818=CARTESIAN_POINT ( 'NONE',  ( -58.15296624161964445, 0.1186235457594081444, 0.2061892363119880722 ) ) ;
#11819=CARTESIAN_POINT ( 'NONE',  ( -50.06058399760020450, 19.37794936593257589, 3.106418048087394634 ) ) ;
#11822=CARTESIAN_POINT ( 'NONE',  ( -47.68734114412297487, 23.26096984540084023, -2.152999274035564792 ) ) ;
#11835=DIRECTION ( 'NONE',  ( 0.3582377630123937395, -0.9336303900108844367, -4.972540365716860457E-16 ) ) ;
#11839=DIRECTION ( 'NONE',  ( -0.7548010569845218232, -0.6559537821943318692, 8.877513919532275149E-16 ) ) ;
#11845=CARTESIAN_POINT ( 'NONE',  ( -58.63679809531399201, -0.7731007215647841546, 1.400195018401728875E-12 ) ) ;
#11847=AXIS2_PLACEMENT_3D ( 'NONE', #37913, #28108, #18300 ) ;
#11852=ORIENTED_EDGE ( 'NONE', *, *, #21925, .F. ) ;
#11859=EDGE_CURVE ( 'NONE', #8945, #17215, #28729, .T. ) ;
#11862=DIRECTION ( 'NONE',  ( -0.8745520943968235761, 0.4849315768086558398, -4.268512490100410909E-16 ) ) ;
#11863=DIRECTION ( 'NONE',  ( 5.188838149069472160E-16, -1.699382548006136559E-16, -1.000000000000000000 ) ) ;
#11867=CARTESIAN_POINT ( 'NONE',  ( -43.93316818929329770, 24.49458088220322338, -1.524000000000007349 ) ) ;
#11870=CARTESIAN_POINT ( 'NONE',  ( -58.31137634086686461, -0.1683406079603727845, 0.3070011007334173536 ) ) ;
#11872=ADVANCED_FACE ( 'NONE', ( #38797 ), #21745, .F. ) ;
#11877=CARTESIAN_POINT ( 'NONE',  ( -54.32300027520380326, 9.724537220608771904, 3.743864951777626349 ) ) ;
#11882=DIRECTION ( 'NONE',  ( 5.188838149069472160E-16, -1.699382548006136559E-16, -1.000000000000000000 ) ) ;
#11884=ORIENTED_EDGE ( 'NONE', *, *, #13594, .T. ) ;
#11886=CARTESIAN_POINT ( 'NONE',  ( -29.57045817498815410, 58.76046099843313897, 1.523999999999994026 ) ) ;
#11888=CARTESIAN_POINT ( 'NONE',  ( -41.09676540851936011, 23.04694042099051998, 1.523999999999990917 ) ) ;
#11889=LINE ( 'NONE', #15070, #14722 ) ;
#11901=CARTESIAN_POINT ( 'NONE',  ( -56.40094345217906380, 3.567796355414390330, 1.062368598836890499 ) ) ;
#11905=EDGE_LOOP ( 'NONE', ( #37868, #7292, #13226, #7904 ) ) ;
#11907=ORIENTED_EDGE ( 'NONE', *, *, #8919, .F. ) ;
#11913=CARTESIAN_POINT ( 'NONE',  ( -5.861642722916909243, 64.54502714855203749, 1.270000000000005347 ) ) ;
#11917=FACE_OUTER_BOUND ( 'NONE', #29552, .T. ) ;
#11931=CARTESIAN_POINT ( 'NONE',  ( -18.88948446928058544, 80.17638627449419175, -1.270000000000003348 ) ) ;
#11932=CARTESIAN_POINT ( 'NONE',  ( -10.84307050033138431, 78.30450799593342026, -1.269999999999998685 ) ) ;
#11937=DIRECTION ( 'NONE',  ( -0.8745520943968250194, 0.4849315768086532863, -5.361993529360574930E-16 ) ) ;
#11938=CIRCLE ( 'NONE', #9900, 0.2539999999999990599 ) ;
#11950=CARTESIAN_POINT ( 'NONE',  ( -11.05715273818225342, 82.67346420587206524, 1.269999999999999796 ) ) ;
#11953=CARTESIAN_POINT ( 'NONE',  ( -19.33375693323417011, 80.42273151551299293, -1.270000000000003570 ) ) ;
#11963=CARTESIAN_POINT ( 'NONE',  ( -4.394136353581306054, 70.68697878297604120, 1.524000000000005350 ) ) ;
#11965=CARTESIAN_POINT ( 'NONE',  ( -52.86182053370306733, 11.13604294806845729, 4.079049242073634396 ) ) ;
#11974=CARTESIAN_POINT ( 'NONE',  ( -58.03414100541873211, 0.4564111095344824953, -0.9708715263941704032 ) ) ;
#11977=CARTESIAN_POINT ( 'NONE',  ( -15.74027684387364978, 85.27021604205610572, 1.523999999999996913 ) ) ;
#11978=CARTESIAN_POINT ( 'NONE',  ( -8.095114962461808616, 74.19100168833409725, 1.270000000000002460 ) ) ;
#11981=DIRECTION ( 'NONE',  ( 5.188838149069472160E-16, -1.699382548006136559E-16, -1.000000000000000000 ) ) ;
#11986=CARTESIAN_POINT ( 'NONE',  ( -58.83227707057486811, -0.08366279997995551554, -5.898546760656774196E-15 ) ) ;
#11996=CARTESIAN_POINT ( 'NONE',  ( -58.50406900891774598, -0.02849845305888287772, -0.6794360696606426275 ) ) ;
#11998=AXIS2_PLACEMENT_3D ( 'NONE', #41429, #8621, #8414 ) ;
#12003=CARTESIAN_POINT ( 'NONE',  ( -56.18489917335774209, 4.374450811265827355, -2.350758010980142920 ) ) ;
#12006=CARTESIAN_POINT ( 'NONE',  ( -51.81113891419111894, 13.24950054771400332, -4.495723625053127392 ) ) ;
#12008=ORIENTED_EDGE ( 'NONE', *, *, #26687, .F. ) ;
#12012=CARTESIAN_POINT ( 'NONE',  ( -57.39043856515510811, 2.569568763584578974, -1.997829887931768411 ) ) ;
#12016=CIRCLE ( 'NONE', #29728, 0.6350000000000014522 ) ;
#12017=EDGE_CURVE ( 'NONE', #37307, #13736, #3032, .T. ) ;
#12020=CARTESIAN_POINT ( 'NONE',  ( -21.18564099849817950, 70.71717898851710515, 1.523999999999996691 ) ) ;
#12021=CIRCLE ( 'NONE', #7936, 0.2540000000000010583 ) ;
#12024=CARTESIAN_POINT ( 'NONE',  ( -58.83227707057486811, -0.08366279997995551554, -1.995625700055530397E-14 ) ) ;
#12027=CARTESIAN_POINT ( 'NONE',  ( -49.65811535071824778, 19.11229591699006036, 3.935810587595351517 ) ) ;
#12031=CARTESIAN_POINT ( 'NONE',  ( -49.59145623469802899, 21.58002366008788542, -1.574391596335681154 ) ) ;
#12034=EDGE_LOOP ( 'NONE', ( #31513, #21724, #10282, #1546 ) ) ;
#12039=AXIS2_PLACEMENT_3D ( 'NONE', #14099, #30085, #17501 ) ;
#12049=VERTEX_POINT ( 'NONE', #2618 ) ;
#12060=AXIS2_PLACEMENT_3D ( 'NONE', #42018, #9831, #38607 ) ;
#12063=EDGE_CURVE ( 'NONE', #20091, #18538, #36233, .T. ) ;
#12068=ORIENTED_EDGE ( 'NONE', *, *, #12649, .F. ) ;
#12076=DIRECTION ( 'NONE',  ( -0.8745520943968245753, 0.4849315768086539524, -5.691349986800526185E-16 ) ) ;
#12079=CARTESIAN_POINT ( 'NONE',  ( -58.18307367792519358, 0.1082273239375445423, 0.5849402378816875858 ) ) ;
#12085=ORIENTED_EDGE ( 'NONE', *, *, #14599, .F. ) ;
#12086=CARTESIAN_POINT ( 'NONE',  ( -54.97180548219925100, 8.422794459035404913, 3.467293221275778325 ) ) ;
#12091=CARTESIAN_POINT ( 'NONE',  ( -36.65473259702431363, 28.27472347546385834, 1.523999999999995802 ) ) ;
#12094=CARTESIAN_POINT ( 'NONE',  ( -29.10098582464626915, 61.33321833257333822, 1.523999999999994026 ) ) ;
#12097=CARTESIAN_POINT ( 'NONE',  ( -29.82321757229076908, 71.17901112636586447, 1.523999999999992250 ) ) ;
#12099=DIRECTION ( 'NONE',  ( 0.9998501190848629872, 0.01731298258490743258, 8.537024980200819846E-16 ) ) ;
#12111=CARTESIAN_POINT ( 'NONE',  ( -55.83515739322315596, 4.224161455597911008, 0.1887094293950665747 ) ) ;
#12123=FACE_OUTER_BOUND ( 'NONE', #12323, .T. ) ;
#12130=CARTESIAN_POINT ( 'NONE',  ( -46.86699512455117400, 25.83114541775341522, 0.4845221143632131300 ) ) ;
#12132=CARTESIAN_POINT ( 'NONE',  ( -45.14658554404967106, 22.88857079803865346, 2.562886992506556272 ) ) ;
#12134=ORIENTED_EDGE ( 'NONE', *, *, #1925, .T. ) ;
#12135=ORIENTED_EDGE ( 'NONE', *, *, #6636, .F. ) ;
#12136=CARTESIAN_POINT ( 'NONE',  ( -18.27007371177420936, 83.88799758123168715, -1.524000000000003574 ) ) ;
#12154=ORIENTED_EDGE ( 'NONE', *, *, #32338, .F. ) ;
#12158=CIRCLE ( 'NONE', #35968, 0.6350000000000014522 ) ;
#12161=ORIENTED_EDGE ( 'NONE', *, *, #9005, .F. ) ;
#12163=CARTESIAN_POINT ( 'NONE',  ( -5.580495364573205386, 77.10007210032874525, 1.270000000000004237 ) ) ;
#12166=CARTESIAN_POINT ( 'NONE',  ( -30.44847906516384128, 70.61110078258337808, -1.270000000000007345 ) ) ;
#12170=CARTESIAN_POINT ( 'NONE',  ( -5.809227842914839179, 77.60418761620948658, 1.524000000000003352 ) ) ;
#12177=DIRECTION ( 'NONE',  ( -0.8745520943968243532, 0.4849315768086547296, -5.361993529360573944E-16 ) ) ;
#12180=FACE_OUTER_BOUND ( 'NONE', #37503, .T. ) ;
#12182=CARTESIAN_POINT ( 'NONE',  ( -55.57144106516901161, 6.156191000065342145, 3.024401744045409401 ) ) ;
#12185=DIRECTION ( 'NONE',  ( 0.8745520943968235761, -0.4849315768086558398, 4.268512490100410909E-16 ) ) ;
#12194=FACE_OUTER_BOUND ( 'NONE', #24191, .T. ) ;
#12202=EDGE_LOOP ( 'NONE', ( #34123, #40570, #31134, #6447 ) ) ;
#12203=CARTESIAN_POINT ( 'NONE',  ( -58.83227707057488232, -0.08366279997998327111, -5.792906548978703126E-15 ) ) ;
#12205=AXIS2_PLACEMENT_3D ( 'NONE', #27288, #36890, #7708 ) ;
#12207=DIRECTION ( 'NONE',  ( -0.8745520943968250194, 0.4849315768086532863, -5.361993529360574930E-16 ) ) ;
#12214=CARTESIAN_POINT ( 'NONE',  ( -57.57892384836331701, 1.967499851525790211, -1.750299182700436162 ) ) ;
#12215=VERTEX_POINT ( 'NONE', #15366 ) ;
#12217=CARTESIAN_POINT ( 'NONE',  ( -11.24191166894635430, 82.34025985790688651, 1.270000000000000240 ) ) ;
#12219=CARTESIAN_POINT ( 'NONE',  ( -56.17894221855530645, 4.386908320153513507, -2.354358595961671519 ) ) ;
#12222=CARTESIAN_POINT ( 'NONE',  ( -49.72660956849071567, 16.83360665160238412, -5.072308565479707099 ) ) ;
#12229=CARTESIAN_POINT ( 'NONE',  ( -57.07867440696631434, 2.606095844753547830, -1.988717289889820661 ) ) ;
#12230=AXIS2_PLACEMENT_3D ( 'NONE', #33776, #1400, #14356 ) ;
#12233=CARTESIAN_POINT ( 'NONE',  ( -46.38316532014823679, 26.05065462784537900, 1.523999999999991140 ) ) ;
#12236=CARTESIAN_POINT ( 'NONE',  ( -5.809227842914839179, 77.60418761620948658, -1.523999999999996025 ) ) ;
#12237=CARTESIAN_POINT ( 'NONE',  ( -41.41491986784952672, 22.70581808553410497, -0.08466666666667260754 ) ) ;
#12240=CARTESIAN_POINT ( 'NONE',  ( -58.30521585032268206, -0.1116666926106041347, 0.6575736669891736330 ) ) ;
#12241=CARTESIAN_POINT ( 'NONE',  ( -51.09578318342275338, 14.49152418417465960, 4.666602106937938643 ) ) ;
#12243=DIRECTION ( 'NONE',  ( -5.188838149069472160E-16, 1.699382548006136559E-16, 1.000000000000000000 ) ) ;
#12244=CARTESIAN_POINT ( 'NONE',  ( -50.78366386294959511, 19.84645248585079003, 1.614153572948400672 ) ) ;
#12246=ORIENTED_EDGE ( 'NONE', *, *, #5103, .T. ) ;
#12247=CARTESIAN_POINT ( 'NONE',  ( -49.65811535071824778, 19.11229591699006036, -3.935810587595368837 ) ) ;
#12255=CARTESIAN_POINT ( 'NONE',  ( -8.473844426907703564, 67.77203500197072117, -1.269999999999995799 ) ) ;
#12258=DIRECTION ( 'NONE',  ( -0.8745520943968013716, 0.4849315768086958633, -4.268512490100402527E-16 ) ) ;
#12261=DIRECTION ( 'NONE',  ( 0.9454731675810336133, -0.3256999990547843615, 5.459396135145337199E-16 ) ) ;
#12265=ORIENTED_EDGE ( 'NONE', *, *, #5278, .F. ) ;
#12274=EDGE_CURVE ( 'NONE', #6241, #22953, #13805, .T. ) ;
#12280=CIRCLE ( 'NONE', #10235, 0.5080000000000000071 ) ;
#12287=DIRECTION ( 'NONE',  ( 0.9454731675810359448, -0.3256999990547780333, 5.459396135145339171E-16 ) ) ;
#12292=FACE_OUTER_BOUND ( 'NONE', #31169, .T. ) ;
#12293=CARTESIAN_POINT ( 'NONE',  ( -58.34308235763123918, -0.2355438472691235297, 0.2038357956814182415 ) ) ;
#12295=EDGE_CURVE ( 'NONE', #26813, #28177, #20384, .T. ) ;
#12298=EDGE_LOOP ( 'NONE', ( #24982, #32957, #25320, #17657 ) ) ;
#12305=EDGE_CURVE ( 'NONE', #29332, #26682, #13007, .T. ) ;
#12306=ORIENTED_EDGE ( 'NONE', *, *, #26450, .T. ) ;
#12308=CARTESIAN_POINT ( 'NONE',  ( -29.81772749291372904, 58.81923324269567388, 1.523999999999992916 ) ) ;
#12311=DIRECTION ( 'NONE',  ( -5.188838149069471174E-16, 1.699382548006136313E-16, 1.000000000000000000 ) ) ;
#12323=EDGE_LOOP ( 'NONE', ( #8223, #11606, #31756, #26983 ) ) ;
#12324=CARTESIAN_POINT ( 'NONE',  ( -54.07635852566403400, 7.689673991023174615, 1.154061576158796454 ) ) ;
#12328=ORIENTED_EDGE ( 'NONE', *, *, #16742, .T. ) ;
#12329=DIRECTION ( 'NONE',  ( -0.7770581983690852956, 0.6294287539884014793, -5.101669463485840682E-16 ) ) ;
#12333=ORIENTED_EDGE ( 'NONE', *, *, #32173, .T. ) ;
#12336=FACE_OUTER_BOUND ( 'NONE', #27193, .T. ) ;
#12340=EDGE_CURVE ( 'NONE', #35654, #28485, #33410, .T. ) ;
#12343=CARTESIAN_POINT ( 'NONE',  ( -46.88219813129796165, 25.44970738892517659, 1.667955656040396750 ) ) ;
#12346=CARTESIAN_POINT ( 'NONE',  ( -45.82931853585290582, 22.14969803457954356, 3.600065900675641029 ) ) ;
#12349=EDGE_LOOP ( 'NONE', ( #8010, #26597, #34834, #30368 ) ) ;
#12350=EDGE_LOOP ( 'NONE', ( #9077, #33131, #20604, #23519 ) ) ;
#12356=AXIS2_PLACEMENT_3D ( 'NONE', #29646, #26445, #3250 ) ;
#12361=CARTESIAN_POINT ( 'NONE',  ( -49.59816314059868603, 17.91649583374772092, 5.069000701391646935 ) ) ;
#12366=CYLINDRICAL_SURFACE ( 'NONE', #37841, 0.6349999999999998979 ) ;
#12375=VECTOR ( 'NONE', #1581, 1000.000000000000114 ) ;
#12377=ORIENTED_EDGE ( 'NONE', *, *, #35598, .T. ) ;
#12378=CIRCLE ( 'NONE', #8875, 0.2539999999999989488 ) ;
#12380=FACE_OUTER_BOUND ( 'NONE', #17626, .T. ) ;
#12383=CARTESIAN_POINT ( 'NONE',  ( -58.83227707057486811, -0.08366279997995551554, -1.529465441686574059E-14 ) ) ;
#12387=DIRECTION ( 'NONE',  ( 0.1565721916418051640, 0.9876665170007951078, -6.504343050004418945E-15 ) ) ;
#12395=EDGE_CURVE ( 'NONE', #28559, #19659, #30143, .T. ) ;
#12402=AXIS2_PLACEMENT_3D ( 'NONE', #42022, #10044, #23225 ) ;
#12403=DIRECTION ( 'NONE',  ( -0.4849315768086535083, -0.8745520943968250194, -1.030032898892974695E-16 ) ) ;
#12414=CARTESIAN_POINT ( 'NONE',  ( -15.02280320640473121, 73.03244360434628391, 1.523999999999999577 ) ) ;
#12421=ORIENTED_EDGE ( 'NONE', *, *, #41542, .T. ) ;
#12427=CARTESIAN_POINT ( 'NONE',  ( -58.37309112374112630, 0.2537668557392232516, -0.9020876489291813627 ) ) ;
#12428=EDGE_LOOP ( 'NONE', ( #16088, #33322, #4572, #4154 ) ) ;
#12429=DIRECTION ( 'NONE',  ( 0.8745520943968243532, -0.4849315768086547296, 6.829619984160642269E-16 ) ) ;
#12430=FACE_OUTER_BOUND ( 'NONE', #25610, .T. ) ;
#12432=CYLINDRICAL_SURFACE ( 'NONE', #8254, 0.6350000000000006750 ) ;
#12435=CARTESIAN_POINT ( 'NONE',  ( -56.04137470801128273, 5.508142037592367757, -2.879222540163135058 ) ) ;
#12436=VECTOR ( 'NONE', #17168, 1000.000000000000227 ) ;
#12438=ORIENTED_EDGE ( 'NONE', *, *, #7655, .F. ) ;
#12442=AXIS2_PLACEMENT_3D ( 'NONE', #38705, #32305, #23112 ) ;
#12443=CARTESIAN_POINT ( 'NONE',  ( -47.44699234454018466, 15.94620872345373108, -7.864955498886620583E-15 ) ) ;
#12444=CIRCLE ( 'NONE', #7007, 0.2540000000000051106 ) ;
#12447=DIRECTION ( 'NONE',  ( -0.7770581983690878491, 0.6294287539883980376, -5.101669463485847584E-16 ) ) ;
#12451=CARTESIAN_POINT ( 'NONE',  ( -49.53550897992070645, 16.97828837979668748, -4.976283659310176688 ) ) ;
#12452=DIRECTION ( 'NONE',  ( -0.8745520943968240202, 0.4849315768086553402, -6.829619984160650158E-16 ) ) ;
#12454=CARTESIAN_POINT ( 'NONE',  ( -57.26626398570029863, 3.526386058942967860, 2.205039086913747948 ) ) ;
#12455=CARTESIAN_POINT ( 'NONE',  ( -53.85529552446512724, 9.524763104166618533, 3.781023158207285295 ) ) ;
#12456=CARTESIAN_POINT ( 'NONE',  ( -4.416771755448872128, 71.99420641645033925, 1.270000000000004903 ) ) ;
#12457=VECTOR ( 'NONE', #6399, 999.9999999999998863 ) ;
#12459=CARTESIAN_POINT ( 'NONE',  ( -49.01671973967525275, 18.67808020721671625, 5.174630477995037836 ) ) ;
#12461=ORIENTED_EDGE ( 'NONE', *, *, #4804, .F. ) ;
#12462=CARTESIAN_POINT ( 'NONE',  ( -49.70354155341430413, 23.42381788805148091, -1.038162449038428732E-14 ) ) ;
#12481=CARTESIAN_POINT ( 'NONE',  ( -58.36978701179569384, -0.2915170370950972978, -0.01128054769438853119 ) ) ;
#12504=DIRECTION ( 'NONE',  ( -5.188838149069471174E-16, 1.699382548006136313E-16, 1.000000000000000000 ) ) ;
#12506=CARTESIAN_POINT ( 'NONE',  ( -58.33175842519683840, -0.2116331208230537997, 0.2444927590478287449 ) ) ;
#12516=CARTESIAN_POINT ( 'NONE',  ( -33.20758249455312239, 49.81222039523557044, 1.523999999999994026 ) ) ;
#12523=DIRECTION ( 'NONE',  ( -0.8745520943968245753, 0.4849315768086539524, -5.691349986800526185E-16 ) ) ;
#12530=ORIENTED_EDGE ( 'NONE', *, *, #14350, .T. ) ;
#12531=CARTESIAN_POINT ( 'NONE',  ( -55.69906247323991266, 5.207560852731635492, 2.143283491784331307 ) ) ;
#12534=VECTOR ( 'NONE', #25991, 1000.000000000000227 ) ;
#12535=DIRECTION ( 'NONE',  ( -0.8745520943968251304, 0.4849315768086532863, -5.424246918827961050E-16 ) ) ;
#12541=DIRECTION ( 'NONE',  ( 0.9816537812491077375, 0.1906721105965137331, 4.769617732184457412E-16 ) ) ;
#12546=CYLINDRICAL_SURFACE ( 'NONE', #26819, 0.2539999999999999480 ) ;
#12548=CARTESIAN_POINT ( 'NONE',  ( -46.60530155212499892, 26.17382724835484709, 0.6632222222222139418 ) ) ;
#12550=CARTESIAN_POINT ( 'NONE',  ( -47.02779878473986486, 24.11651466984139702, 2.637840241488476511 ) ) ;
#12551=DIRECTION ( 'NONE',  ( -0.8745520943968241312, 0.4849315768086548406, -5.691349986800536046E-16 ) ) ;
#12552=EDGE_CURVE ( 'NONE', #32933, #18166, #30201, .T. ) ;
#12556=CARTESIAN_POINT ( 'NONE',  ( -23.91048590848665967, 81.84235438443283783, 1.523999999999993138 ) ) ;
#12560=CARTESIAN_POINT ( 'NONE',  ( -46.60530155212502024, 26.17382724835479735, -8.515758108943001820E-15 ) ) ;
#12563=DIRECTION ( 'NONE',  ( 0.7548010569845218232, 0.6559537821943318692, 2.801824109679581255E-16 ) ) ;
#12569=FACE_OUTER_BOUND ( 'NONE', #7299, .T. ) ;
#12573=ORIENTED_EDGE ( 'NONE', *, *, #2230, .T. ) ;
#12580=VERTEX_POINT ( 'NONE', #17411 ) ;
#12588=CARTESIAN_POINT ( 'NONE',  ( -48.12298631510321201, 19.54404807545288847, -5.380074092861952373 ) ) ;
#12591=EDGE_CURVE ( 'NONE', #1811, #20091, #12444, .T. ) ;
#12598=CARTESIAN_POINT ( 'NONE',  ( -58.71347258051977036, -0.3150591082031195533, 0.2754856216383245182 ) ) ;
#12612=DIRECTION ( 'NONE',  ( -0.8745520943968240202, 0.4849315768086551737, -5.361993529360572958E-16 ) ) ;
#12616=DIRECTION ( 'NONE',  ( 5.188838149069472160E-16, -1.699382548006136559E-16, -1.000000000000000000 ) ) ;
#12620=ORIENTED_EDGE ( 'NONE', *, *, #10423, .T. ) ;
#12622=VERTEX_POINT ( 'NONE', #24423 ) ;
#12623=CARTESIAN_POINT ( 'NONE',  ( -6.135835944515187101, 77.40800365160224317, -1.523999999999996247 ) ) ;
#12628=CARTESIAN_POINT ( 'NONE',  ( -53.78496643398889177, 9.658663915604030592, -3.808424989279795003 ) ) ;
#12630=ORIENTED_EDGE ( 'NONE', *, *, #6783, .F. ) ;
#12631=CARTESIAN_POINT ( 'NONE',  ( -58.34169784303185224, -0.2326338189567039860, -0.2089577666115286780 ) ) ;
#12636=CARTESIAN_POINT ( 'NONE',  ( -4.466782427718574588, 71.06098887363195615, -1.269999999999994245 ) ) ;
#12639=CARTESIAN_POINT ( 'NONE',  ( -57.26626398570029863, 3.526386058942967860, -2.205039086913768820 ) ) ;
#12640=VERTEX_POINT ( 'NONE', #27840 ) ;
#12643=ORIENTED_EDGE ( 'NONE', *, *, #5652, .F. ) ;
#12648=CARTESIAN_POINT ( 'NONE',  ( -57.72731561024293967, 0.8685078910841970146, -1.009486960136972124E-14 ) ) ;
#12649=EDGE_CURVE ( 'NONE', #32069, #3009, #36262, .T. ) ;
#12654=FACE_OUTER_BOUND ( 'NONE', #7762, .T. ) ;
#12655=CARTESIAN_POINT ( 'NONE',  ( -49.74050263075070433, 15.22813595918496432, -2.996737790144743840 ) ) ;
#12657=DIRECTION ( 'NONE',  ( 0.8745520943968235761, -0.4849315768086558398, 0.000000000000000000 ) ) ;
#12658=CARTESIAN_POINT ( 'NONE',  ( -15.27962295839633811, 80.49293118800726177, -1.270000000000001350 ) ) ;
#12659=CARTESIAN_POINT ( 'NONE',  ( -49.54931586048707715, 17.00517315445653210, 5.017750506970054758 ) ) ;
#12660=CARTESIAN_POINT ( 'NONE',  ( -23.75665686005077504, 76.91945007112674659, -1.524000000000005128 ) ) ;
#12662=CARTESIAN_POINT ( 'NONE',  ( -57.76461416131697746, 2.594137363129217277, 1.330350326707359754 ) ) ;
#12663=AXIS2_PLACEMENT_3D ( 'NONE', #6865, #22182, #3257 ) ;
#12666=ORIENTED_EDGE ( 'NONE', *, *, #2385, .F. ) ;
#12667=CARTESIAN_POINT ( 'NONE',  ( -55.24575511360199442, 11.19612964283759560, -1.091162240856589107E-14 ) ) ;
#12669=DIRECTION ( 'NONE',  ( -0.6559537821943318692, 0.7548010569845216011, -4.686333752532438436E-16 ) ) ;
#12681=CARTESIAN_POINT ( 'NONE',  ( -22.98045850745952023, 78.35500052582088415, -1.524000000000005128 ) ) ;
#12683=ORIENTED_EDGE ( 'NONE', *, *, #22948, .F. ) ;
#12685=ORIENTED_EDGE ( 'NONE', *, *, #23345, .T. ) ;
#12686=CARTESIAN_POINT ( 'NONE',  ( -16.46263872254443683, 83.91929436251373886, -1.270000000000002460 ) ) ;
#12692=DIRECTION ( 'NONE',  ( 5.188838149069472160E-16, -1.699382548006136559E-16, -1.000000000000000000 ) ) ;
#12699=CARTESIAN_POINT ( 'NONE',  ( -45.91718695868514288, 25.22619731686664224, -1.578102078770073469 ) ) ;
#12700=CIRCLE ( 'NONE', #14725, 0.2540000000000010583 ) ;
#12701=ORIENTED_EDGE ( 'NONE', *, *, #41794, .T. ) ;
#12704=DIRECTION ( 'NONE',  ( -0.4849315768086535638, -0.8745520943968251304, 5.189481155063205320E-13 ) ) ;
#12717=CARTESIAN_POINT ( 'NONE',  ( -20.21600168833980149, 80.16988503754176065, -1.524000000000003796 ) ) ;
#12721=CARTESIAN_POINT ( 'NONE',  ( -29.82321757229076908, 71.17901112636586447, 1.523999999999992250 ) ) ;
#12729=CARTESIAN_POINT ( 'NONE',  ( -54.71920516550231639, 7.857264873378122516, -3.427457936772596803 ) ) ;
#12734=ORIENTED_EDGE ( 'NONE', *, *, #32894, .F. ) ;
#12742=ADVANCED_FACE ( 'NONE', ( #14626 ), #31298, .T. ) ;
#12749=AXIS2_PLACEMENT_3D ( 'NONE', #7503, #13464, #16861 ) ;
#12752=CARTESIAN_POINT ( 'NONE',  ( -46.70260003083688360, 25.98261893038500148, 1.346190830585627607 ) ) ;
#12753=CARTESIAN_POINT ( 'NONE',  ( -46.71787546252079437, 26.08696747599453047, 0.2117558669993397091 ) ) ;
#12755=CARTESIAN_POINT ( 'NONE',  ( -48.04822308881583126, 19.89521662531995005, 5.294633059834397137 ) ) ;
#12756=CARTESIAN_POINT ( 'NONE',  ( -58.68548670125471745, -0.3142138667033253507, 0.3043876634576400675 ) ) ;
#12765=AXIS2_PLACEMENT_3D ( 'NONE', #11788, #15607, #27976 ) ;
#12766=CARTESIAN_POINT ( 'NONE',  ( -5.580495364573204498, 77.10007210032874525, -1.523999999999995802 ) ) ;
#12767=CARTESIAN_POINT ( 'NONE',  ( -30.28638171898572651, 70.19821000523995735, -1.270000000000007345 ) ) ;
#12784=CARTESIAN_POINT ( 'NONE',  ( -41.05189575270517111, 23.09451173561986792, 0.08466666666666186614 ) ) ;
#12790=CARTESIAN_POINT ( 'NONE',  ( -47.98478927898735691, 19.46741901348697468, -5.364673458605423662 ) ) ;
#12791=ADVANCED_FACE ( 'NONE', ( #28492 ), #15831, .T. ) ;
#12798=CARTESIAN_POINT ( 'NONE',  ( -58.08606908514041578, 0.8771027734568864753, 1.270208019422672807 ) ) ;
#12799=ADVANCED_FACE ( 'NONE', ( #28906 ), #35387, .T. ) ;
#12804=DIRECTION ( 'NONE',  ( 5.188838149069472160E-16, -1.699382548006136559E-16, -1.000000000000000000 ) ) ;
#12813=DIRECTION ( 'NONE',  ( -5.188838149069472160E-16, 1.699382548006136559E-16, 1.000000000000000000 ) ) ;
#12815=DIRECTION ( 'NONE',  ( 5.188838149069472160E-16, -1.699382548006136559E-16, -1.000000000000000000 ) ) ;
#12821=EDGE_CURVE ( 'NONE', #30637, #31609, #28830, .T. ) ;
#12826=ORIENTED_EDGE ( 'NONE', *, *, #27964, .T. ) ;
#12827=CARTESIAN_POINT ( 'NONE',  ( -42.03620417734866521, 22.24401450883890519, -1.718184518067733979 ) ) ;
#12833=CARTESIAN_POINT ( 'NONE',  ( -56.39031313087512132, 4.472451144598750261, -2.570725850350818131 ) ) ;
#12834=EDGE_LOOP ( 'NONE', ( #29289, #39672, #27833, #41076 ) ) ;
#12835=CARTESIAN_POINT ( 'NONE',  ( -58.60151899684548482, -0.7129426177418396460, -0.1461293658723255284 ) ) ;
#12840=AXIS2_PLACEMENT_3D ( 'NONE', #29096, #38906, #19086 ) ;
#12844=CARTESIAN_POINT ( 'NONE',  ( -58.09657527255103560, 0.9821181129459344294, -1.359330230256445393 ) ) ;
#12848=ORIENTED_EDGE ( 'NONE', *, *, #20710, .F. ) ;
#12852=CARTESIAN_POINT ( 'NONE',  ( -8.480639930781094904, 68.51064353654967931, 1.270000000000002460 ) ) ;
#12858=DIRECTION ( 'NONE',  ( 0.5149185422762164732, -0.8572391118119474518, -5.501763788286270478E-15 ) ) ;
#12860=CIRCLE ( 'NONE', #10134, 0.7620000000000015650 ) ;
#12861=CARTESIAN_POINT ( 'NONE',  ( -47.89521659674720411, 15.90546175020217312, -0.7967971578063902660 ) ) ;
#12862=AXIS2_PLACEMENT_3D ( 'NONE', #30267, #1108, #692 ) ;
#12864=CARTESIAN_POINT ( 'NONE',  ( -46.75005564411527104, 25.87286441723897568, -1.401665496903889085 ) ) ;
#12865=CARTESIAN_POINT ( 'NONE',  ( -51.05584078844552920, 14.55899147689505391, 4.676820903699452359 ) ) ;
#12866=CARTESIAN_POINT ( 'NONE',  ( -11.34554992887676406, 77.73165686004495001, 1.524000000000000687 ) ) ;
#12868=CARTESIAN_POINT ( 'NONE',  ( -56.03617394834085985, 6.499552843647532718, 2.676235688315251604 ) ) ;
#12869=CARTESIAN_POINT ( 'NONE',  ( -57.83637253161431602, 2.237724655402451024, 1.757929103219288747 ) ) ;
#12872=CARTESIAN_POINT ( 'NONE',  ( -53.84631020977099780, 15.55534180641097386, -0.3033304672099482735 ) ) ;
#12875=ORIENTED_EDGE ( 'NONE', *, *, #2142, .F. ) ;
#12880=DIRECTION ( 'NONE',  ( 0.8745520943968240202, -0.4849315768086553402, 6.829619984160650158E-16 ) ) ;
#12882=ADVANCED_FACE ( 'NONE', ( #37360 ), #8180, .T. ) ;
#12887=CARTESIAN_POINT ( 'NONE',  ( -29.91360363449004822, 70.04874496952839991, -1.270000000000007123 ) ) ;
#12889=ORIENTED_EDGE ( 'NONE', *, *, #25006, .T. ) ;
#12892=CARTESIAN_POINT ( 'NONE',  ( -58.36458372496356617, -0.2806544840891243009, -0.08969953854032418350 ) ) ;
#12898=CARTESIAN_POINT ( 'NONE',  ( -8.305181614181256222, 72.61062586887042869, 1.270000000000002682 ) ) ;
#12905=CARTESIAN_POINT ( 'NONE',  ( -44.90991502375803890, 23.16658271142636139, -2.247441098035906748 ) ) ;
#12909=DIRECTION ( 'NONE',  ( 5.188838149069472160E-16, -1.699382548006136559E-16, -1.000000000000000000 ) ) ;
#12916=CYLINDRICAL_SURFACE ( 'NONE', #1822, 0.2539999999999962288 ) ;
#12932=CARTESIAN_POINT ( 'NONE',  ( -4.466782427718574588, 71.06098887363195615, -1.269999999999994245 ) ) ;
#12941=ORIENTED_EDGE ( 'NONE', *, *, #1190, .T. ) ;
#12944=CIRCLE ( 'NONE', #14303, 0.2539999999999981162 ) ;
#12946=ORIENTED_EDGE ( 'NONE', *, *, #25522, .T. ) ;
#12949=FACE_OUTER_BOUND ( 'NONE', #28274, .T. ) ;
#12951=CIRCLE ( 'NONE', #3465, 0.7619999999999976792 ) ;
#12954=CARTESIAN_POINT ( 'NONE',  ( -50.93622740537085747, 14.57546966384534848, 4.560176109731806982 ) ) ;
#12955=CARTESIAN_POINT ( 'NONE',  ( -46.93283292234357162, 25.30718002661817323, 1.635697237164823514 ) ) ;
#12956=AXIS2_PLACEMENT_3D ( 'NONE', #10632, #14033, #10839 ) ;
#12958=CARTESIAN_POINT ( 'NONE',  ( -43.10982161678889213, 22.52422253607401359, 1.888110242252979631 ) ) ;
#12959=CARTESIAN_POINT ( 'NONE',  ( -7.994219716368544226, 68.36415334912796027, -1.269999999999995577 ) ) ;
#12961=CARTESIAN_POINT ( 'NONE',  ( -58.28497307353763546, -0.1385909279409125450, -0.01567725181050762251 ) ) ;
#12982=VERTEX_POINT ( 'NONE', #28823 ) ;
#12990=CARTESIAN_POINT ( 'NONE',  ( -46.53889185657398286, 18.10826295091780835, 1.459106928557426963 ) ) ;
#12997=DIRECTION ( 'NONE',  ( 5.188838149069472160E-16, -1.699382548006136559E-16, -1.000000000000000000 ) ) ;
#13004=AXIS2_PLACEMENT_3D ( 'NONE', #9762, #3383, #1455 ) ;
#13005=DIRECTION ( 'NONE',  ( 5.188838149069472160E-16, -1.699382548006136559E-16, -1.000000000000000000 ) ) ;
#13006=CARTESIAN_POINT ( 'NONE',  ( -58.22785051087649322, 0.5684335961332193099, 1.101539904997213215 ) ) ;
#13007=LINE ( 'NONE', #7636, #19239 ) ;
#13019=DIRECTION ( 'NONE',  ( 0.4849315768086481238, 0.8745520943968281280, -3.311806702191031061E-15 ) ) ;
#13021=CARTESIAN_POINT ( 'NONE',  ( -7.842268484490568348, 73.30875693322846587, -1.269999999999996243 ) ) ;
#13025=CARTESIAN_POINT ( 'NONE',  ( -46.98348089488076340, 24.79145570443882463, -2.118842393845993044 ) ) ;
#13036=AXIS2_PLACEMENT_3D ( 'NONE', #1092, #16623, #7481 ) ;
#13041=CARTESIAN_POINT ( 'NONE',  ( -58.64992616607198528, -0.3153078225257616718, -0.3300484825081549944 ) ) ;
#13042=EDGE_LOOP ( 'NONE', ( #12620, #31800, #23355, #14667 ) ) ;
#13043=CARTESIAN_POINT ( 'NONE',  ( -58.36915991843427776, -0.2902476589034808097, -0.03232548579177411258 ) ) ;
#13049=CARTESIAN_POINT ( 'NONE',  ( -58.30521585032268206, -0.1116666926106041347, -0.6575736669891941721 ) ) ;
#13050=VERTEX_POINT ( 'NONE', #16080 ) ;
#13053=ORIENTED_EDGE ( 'NONE', *, *, #39249, .T. ) ;
#13057=B_SPLINE_CURVE_WITH_KNOTS ( 'NONE', 3,
 ( #38683, #29510, #19691, #32285, #12481, #23089, #22875, #3542, #42097, #13316, #26302, #41888, #9289, #6305, #39311, #32070, #6101, #31860, #22250, #28661, #12892, #25676, #38887, #3114, #25475, #19484, #2700, #41673, #16074, #9489, #9699, #39100, #22454, #35276, #19064, #22665, #135, #32493, #29292, #14144, #40159, #24148, #3754, #23725, #23939, #39741, #33134, #27147, #10951, #37157, #10540, #33555, #36743, #20314, #13941, #3964, #20525, #29715, #16925, #14345, #557, #33341, #4387, #23509, #1389, #36337, #39950, #36956, #19908, #30135, #26520, #29925, #36536, #4171, #7777, #27355, #16712, #763, #11163, #7355, #32923, #17549, #26733, #17345, #17133, #13532, #974, #4590, #26939, #10744, #33765, #39526, #40368, #10330, #13739, #23300, #30550, #7153, #7565, #30334, #20112, #1181, #20740, #41199, #18595, #34594, #2014, #5216, #8182, #40987, #30965, #24781, #8604, #1601, #12003, #12219, #11790, #4800, #33972, #31604, #18170, #5638, #17751, #41412, #37779, #5006, #2442, #2229, #24995, #21566, #31173, #14767, #40780, #8394, #11371, #30751, #11577, #15403, #14558, #25209, #5423, #18378, #28407, #37362, #37995, #7979, #1806, #31387, #14977, #15190, #20947, #17965, #27978, #27565, #28193, #8819, #40574, #24358 ),
 .UNSPECIFIED., .F., .F.,
 ( 4, 2, 2, 2, 2, 2, 2, 2, 2, 1, 2, 2, 2, 2, 1, 2, 2, 2, 1, 1, 1, 2, 2, 2, 2, 2, 2, 2, 2, 2, 1, 2, 2, 2, 2, 1, 1, 1, 2, 2, 2, 2, 2, 1, 2, 2, 2, 1, 2, 2, 2, 2, 2, 1, 1, 1, 2, 1, 2, 2, 2, 2, 2, 1, 1, 1, 1, 2, 2, 2, 2, 2, 1, 1, 1, 1, 2, 2, 2, 2, 1, 1, 1, 1, 2, 2, 2, 1, 2, 2, 2, 2, 4 ),
 ( 0.000000000000000000, 0.0004882812499988943306, 0.0007324218749983417128, 0.0008544921874980726138, 0.0009765624999978036232, 0.001464843749996776233, 0.001708984374996262538, 0.001953124999995749060, 0.002929687499993625325, 0.003417968749992564542, 0.003662109374992034583, 0.003906249999991504192, 0.005859374999987647901, 0.006835937499985785676, 0.007324218749984854129, 0.007568359374984387489, 0.007812499999983922583, 0.01171874999997702359, 0.01367187499997357149, 0.01464843749997184717, 0.01513671874997098328, 0.01538085937497043684, 0.01562499999996988867, 0.02343749999994880831, 0.02734374999993813282, 0.02929687499993280028, 0.03027343749993023289, 0.03124999999992766897, 0.03906249999990741434, 0.04296874999989729049, 0.04492187499989241245, 0.04589843749988977567, 0.04687499999988713195, 0.05468749999986757121, 0.05859374999985778737, 0.06054687499985289545, 0.06152343749985028643, 0.06201171874984880150, 0.06225585937484824639, 0.06249999999984768434, 0.07031249999985582366, 0.07128906249985692001, 0.07226562499985801635, 0.07421874999986018129, 0.07812499999986419197, 0.08007812499986623200, 0.08105468749986723120, 0.08203124999986824428, 0.08593749999987203292, 0.09374999999987990162, 0.09765624999988384292, 0.09814453124988455068, 0.09863281249988525845, 0.09960937499988636867, 0.1015624999998882283, 0.1093749999998950700, 0.1171874999999019257, 0.1210937499999053396, 0.1230468749999070605, 0.1249999999999087674, 0.1874999999999688860, 0.2187499999999987232, 0.2343750000000136835, 0.2421875000000211220, 0.2460937500000248412, 0.2480468750000264788, 0.2490234375000273670, 0.2495117187500278944, 0.2500000000000284217, 0.3750000000000308087, 0.4375000000000319744, 0.4687500000000323630, 0.4843750000000326961, 0.4921875000000331402, 0.4960937500000334732, 0.4980468750000338618, 0.4990234375000341394, 0.5000000000000344169, 0.6250000000000179856, 0.6875000000000095479, 0.7187500000000052180, 0.7343750000000032196, 0.7421875000000021094, 0.7460937500000018874, 0.7480468750000017764, 0.7500000000000016653, 0.8750000000000047740, 0.9062500000000055511, 0.9218750000000058842, 0.9257812500000057732, 0.9296875000000055511, 0.9375000000000052180, 1.000000000000000000 ),
 .UNSPECIFIED. ) ;
#13058=VECTOR ( 'NONE', #38611, 1000.000000000000114 ) ;
#13059=EDGE_CURVE ( 'NONE', #11474, #25, #23360, .T. ) ;
#13060=CARTESIAN_POINT ( 'NONE',  ( -49.14072577824711630, 13.89916973120783972, -8.531461402113531655E-15 ) ) ;
#13063=CARTESIAN_POINT ( 'NONE',  ( -47.19079517381230460, 25.11791606914811936, 2.000773461933185171 ) ) ;
#13066=CARTESIAN_POINT ( 'NONE',  ( -8.270297712355500153, 69.35377921309405735, -1.523999999999995802 ) ) ;
#13068=CARTESIAN_POINT ( 'NONE',  ( -50.02669608763527265, 12.78473261814652773, -0.3947048150275272449 ) ) ;
#13071=LINE ( 'NONE', #19036, #37014 ) ;
#13072=CARTESIAN_POINT ( 'NONE',  ( -48.73363302905276129, 18.22424113963231207, 5.158540213015197828 ) ) ;
#13075=DIRECTION ( 'NONE',  ( -0.8745520943968235761, 0.4849315768086558953, -5.361993529360570985E-16 ) ) ;
#13077=CARTESIAN_POINT ( 'NONE',  ( -56.91719228404756592, 5.442273006173628858, 0.3640331681397596664 ) ) ;
#13078=EDGE_CURVE ( 'NONE', #18488, #22953, #39050, .T. ) ;
#13079=CARTESIAN_POINT ( 'NONE',  ( -57.29531047346088712, 2.067549486662559222, 1.749273462387482603 ) ) ;
#13081=ORIENTED_EDGE ( 'NONE', *, *, #11560, .F. ) ;
#13082=CARTESIAN_POINT ( 'NONE',  ( -52.06588384954375925, 19.72955628912294301, -0.3571238398875267728 ) ) ;
#13084=ORIENTED_EDGE ( 'NONE', *, *, #17244, .F. ) ;
#13090=VECTOR ( 'NONE', #9575, 1000.000000000000000 ) ;
#13098=DIRECTION ( 'NONE',  ( 0.4849315768086480127, 0.8745520943968279060, 1.030032898892941415E-16 ) ) ;
#13099=ORIENTED_EDGE ( 'NONE', *, *, #7427, .F. ) ;
#13110=AXIS2_PLACEMENT_3D ( 'NONE', #20965, #34607, #21792 ) ;
#13113=EDGE_CURVE ( 'NONE', #13951, #12049, #39730, .T. ) ;
#13114=ORIENTED_EDGE ( 'NONE', *, *, #39889, .T. ) ;
#13117=( BOUNDED_SURFACE ( )  B_SPLINE_SURFACE ( 3, 2, ( 
 ( #20771, #17377, #7187 ),
 ( #20146, #23757, #29751 ),
 ( #30367, #33795, #7386 ),
 ( #17166, #11192, #36779 ),
 ( #7595, #10988, #20346 ),
 ( #13769, #1216, #10363 ) ),
 .UNSPECIFIED., .F., .F., .T. ) 
 B_SPLINE_SURFACE_WITH_KNOTS ( ( 4, 2, 4 ),
 ( 3, 3 ),
 ( 0.000000000000000000, 0.0007381999790946869831, 0.001476399958189373966 ),
 ( 0.000000000000000000, 1.000000000000000000 ),
 .UNSPECIFIED. ) 
 GEOMETRIC_REPRESENTATION_ITEM ( )  RATIONAL_B_SPLINE_SURFACE ( (
 ( 1.000000000000000000, 0.7071067811865393571, 1.000000000000000000),
 ( 1.000000000000000000, 0.7071031648639772849, 1.000000000000000000),
 ( 1.000000000000000000, 0.7049885726714537615, 1.000000000000000000),
 ( 1.000000000000000000, 0.6987948356736179978, 1.000000000000000000),
 ( 1.000000000000000000, 0.6949210395568362619, 1.000000000000000000),
 ( 1.000000000000000000, 0.6916534930271285297, 1.000000000000000000) ) ) 
 REPRESENTATION_ITEM ( '' )  SURFACE ( )  );
#13119=CARTESIAN_POINT ( 'NONE',  ( -45.39816439898302036, 21.06106408185672763, -4.080402960186392036 ) ) ;
#13120=ORIENTED_EDGE ( 'NONE', *, *, #30501, .F. ) ;
#13124=DIRECTION ( 'NONE',  ( -0.8745520943968250194, 0.4849315768086532863, -5.361993529360574930E-16 ) ) ;
#13125=AXIS2_PLACEMENT_3D ( 'NONE', #29441, #10476, #26237 ) ;
#13127=EDGE_CURVE ( 'NONE', #8502, #32851, #3702, .T. ) ;
#13132=CYLINDRICAL_SURFACE ( 'NONE', #39931, 0.6349999999999984546 ) ;
#13135=ADVANCED_FACE ( 'NONE', ( #28882 ), #35490, .T. ) ;
#13138=CARTESIAN_POINT ( 'NONE',  ( -10.32579803928178386, 77.06797118195436269, 1.270000000000000906 ) ) ;
#13141=DIRECTION ( 'NONE',  ( 0.9454731675810330582, -0.3256999990547864710, 5.459396135145336213E-16 ) ) ;
#13143=ORIENTED_EDGE ( 'NONE', *, *, #22178, .F. ) ;
#13151=CARTESIAN_POINT ( 'NONE',  ( -7.994219716368544226, 68.36415334912796027, 1.270000000000003570 ) ) ;
#13158=VECTOR ( 'NONE', #10594, 1000.000000000000000 ) ;
#13169=DIRECTION ( 'NONE',  ( 0.3256999990547876367, 0.9454731675810326141, 8.328397965208553695E-18 ) ) ;
#13172=EDGE_CURVE ( 'NONE', #31070, #9063, #31560, .T. ) ;
#13176=CARTESIAN_POINT ( 'NONE',  ( -46.69404853191296212, 26.00096993889310681, 1.337746353888202622 ) ) ;
#13177=CARTESIAN_POINT ( 'NONE',  ( -47.62967605938791849, 25.45029596856965171, -8.552750547210872508E-15 ) ) ;
#13179=CARTESIAN_POINT ( 'NONE',  ( -53.45432727069204759, 10.77832982246877691, 4.078803160923774485 ) ) ;
#13182=CARTESIAN_POINT ( 'NONE',  ( -58.37241122568488549, -0.2962816677227891882, -1.025775813386803588E-14 ) ) ;
#13183=AXIS2_PLACEMENT_3D ( 'NONE', #5662, #38018, #34829 ) ;
#13184=ORIENTED_EDGE ( 'NONE', *, *, #5549, .T. ) ;
#13189=CARTESIAN_POINT ( 'NONE',  ( -46.79514595010191158, 25.77136020477034606, -0.9526608576032509212 ) ) ;
#13191=AXIS2_PLACEMENT_3D ( 'NONE', #12721, #39351, #39567 ) ;
#13204=DIRECTION ( 'NONE',  ( -5.188838149069471174E-16, 1.699382548006136313E-16, 1.000000000000000000 ) ) ;
#13207=AXIS2_PLACEMENT_3D ( 'NONE', #29622, #457, #19181 ) ;
#13213=ORIENTED_EDGE ( 'NONE', *, *, #6882, .F. ) ;
#13214=CARTESIAN_POINT ( 'NONE',  ( -42.93826774478920072, 21.39662913260299959, 1.244340269653798181 ) ) ;
#13220=CIRCLE ( 'NONE', #4401, 8.794749999999995183 ) ;
#13226=ORIENTED_EDGE ( 'NONE', *, *, #16245, .F. ) ;
#13230=CARTESIAN_POINT ( 'NONE',  ( -58.80981292533127203, -0.2807566353364293610, 0.1195710083426413800 ) ) ;
#13241=CARTESIAN_POINT ( 'NONE',  ( -28.42835727709238114, 77.69497285144578314, 1.269999999999991358 ) ) ;
#13245=CARTESIAN_POINT ( 'NONE',  ( -7.772068811996249771, 69.25462295839062676, -1.269999999999995577 ) ) ;
#13246=CARTESIAN_POINT ( 'NONE',  ( -24.16603736854983708, 76.82831944025377879, -1.524000000000005350 ) ) ;
#13251=LINE ( 'NONE', #6445, #28984 ) ;
#13253=CARTESIAN_POINT ( 'NONE',  ( -18.58115504727956591, 80.30342350548193053, 1.269999999999996243 ) ) ;
#13258=CARTESIAN_POINT ( 'NONE',  ( -58.64011137842675225, -0.3059599299333538580, -0.3495911961056130113 ) ) ;
#13260=CARTESIAN_POINT ( 'NONE',  ( -17.14500000000466784, 71.11999999999886768, -1.270000000000000684 ) ) ;
#13264=CARTESIAN_POINT ( 'NONE',  ( -5.684927786827005392, 65.51297084251929448, -1.269999999999993801 ) ) ;
#13267=CARTESIAN_POINT ( 'NONE',  ( -57.52317756609133426, 3.014644041894651405, -1.981665235817958948 ) ) ;
#13268=ORIENTED_EDGE ( 'NONE', *, *, #32116, .F. ) ;
#13271=ORIENTED_EDGE ( 'NONE', *, *, #35252, .T. ) ;
#13282=CARTESIAN_POINT ( 'NONE',  ( -6.318938770521977055, 64.36956080246774548, 1.524000000000005350 ) ) ;
#13283=CARTESIAN_POINT ( 'NONE',  ( -46.67338572489354931, 16.85372243840488338, -7.793947694802422673E-15 ) ) ;
#13286=CARTESIAN_POINT ( 'NONE',  ( -46.66121569171162520, 26.06868089111461373, -1.308362493757629030 ) ) ;
#13287=CARTESIAN_POINT ( 'NONE',  ( -28.74159376897886276, 60.61225341505600284, 1.269999999999992912 ) ) ;
#13288=CARTESIAN_POINT ( 'NONE',  ( -29.91360363449003401, 70.04874496952835727, -1.524000000000007127 ) ) ;
#13291=FACE_OUTER_BOUND ( 'NONE', #26408, .T. ) ;
#13292=CARTESIAN_POINT ( 'NONE',  ( -56.01560174880540188, 6.374421267034191985, 2.942705720416951110 ) ) ;
#13293=CARTESIAN_POINT ( 'NONE',  ( -57.53497731650991653, 2.247686704661286505, 1.882970859819747433 ) ) ;
#13295=ORIENTED_EDGE ( 'NONE', *, *, #18274, .T. ) ;
#13296=CARTESIAN_POINT ( 'NONE',  ( -51.58376292578905975, 16.21309621351152330, -3.606096628736487730 ) ) ;
#13306=DIRECTION ( 'NONE',  ( -0.6294287539884133587, -0.7770581983690755257, 0.000000000000000000 ) ) ;
#13316=CARTESIAN_POINT ( 'NONE',  ( -58.36932441242797864, -0.2905635077575413061, -0.02691069531237075610 ) ) ;
#13329=EDGE_CURVE ( 'NONE', #33817, #26454, #7103, .T. ) ;
#13330=CARTESIAN_POINT ( 'NONE',  ( -45.68084146533627177, 21.25878370237693815, -4.188014402015116211 ) ) ;
#13339=VECTOR ( 'NONE', #18405, 1000.000000000000000 ) ;
#13344=EDGE_LOOP ( 'NONE', ( #36221, #32085, #38946, #27849 ) ) ;
#13354=ADVANCED_FACE ( 'NONE', ( #1319 ), #16852, .T. ) ;
#13359=ADVANCED_FACE ( 'NONE', ( #14276 ), #8419, .T. ) ;
#13363=DIRECTION ( 'NONE',  ( 5.188838149069472160E-16, -1.699382548006136559E-16, -1.000000000000000000 ) ) ;
#13369=ORIENTED_EDGE ( 'NONE', *, *, #21698, .F. ) ;
#13374=CARTESIAN_POINT ( 'NONE',  ( -44.77556674759969013, 21.10465188057021280, 3.405155276520678065 ) ) ;
#13376=ORIENTED_EDGE ( 'NONE', *, *, #29579, .T. ) ;
#13378=LINE ( 'NONE', #6780, #28358 ) ;
#13379=CARTESIAN_POINT ( 'NONE',  ( -7.961576494521615643, 72.55615504727386167, -1.269999999999996243 ) ) ;
#13380=CIRCLE ( 'NONE', #37193, 0.5079999999999993410 ) ;
#13385=AXIS2_PLACEMENT_3D ( 'NONE', #31450, #8244, #21216 ) ;
#13387=CARTESIAN_POINT ( 'NONE',  ( -47.01877684503696742, 24.36789988528162354, 2.430126310640454257 ) ) ;
#13389=CARTESIAN_POINT ( 'NONE',  ( -48.82738941085167284, 18.57305038084609095, 5.399437279161905856 ) ) ;
#13390=DIRECTION ( 'NONE',  ( -0.7284927773988648658, -0.6850534820564654348, -3.970048430162226266E-15 ) ) ;
#13392=CARTESIAN_POINT ( 'NONE',  ( -58.29601494275114959, -0.1585044380288253008, -0.03613930236864761059 ) ) ;
#13395=CARTESIAN_POINT ( 'NONE',  ( -47.02779878473986486, 24.11651466984139702, 2.637840241488476511 ) ) ;
#13397=ADVANCED_FACE ( 'NONE', ( #29200 ), #3659, .F. ) ;
#13402=DIRECTION ( 'NONE',  ( -5.188838149069471174E-16, 1.699382548006136313E-16, 1.000000000000000000 ) ) ;
#13409=ADVANCED_FACE ( 'NONE', ( #30670 ), #27484, .T. ) ;
#13412=CARTESIAN_POINT ( 'NONE',  ( -8.095114962461808616, 74.19100168833409725, -1.523999999999996691 ) ) ;
#13418=EDGE_CURVE ( 'NONE', #41583, #13983, #19992, .T. ) ;
#13422=CARTESIAN_POINT ( 'NONE',  ( -46.62078961162516322, 17.34433182989875277, 0.7188397291161463531 ) ) ;
#13435=AXIS2_PLACEMENT_3D ( 'NONE', #30681, #2578, #25549 ) ;
#13436=ORIENTED_EDGE ( 'NONE', *, *, #40122, .F. ) ;
#13439=LINE ( 'NONE', #39, #31346 ) ;
#13440=DIRECTION ( 'NONE',  ( 5.188838149069472160E-16, -1.699382548006136559E-16, -1.000000000000000000 ) ) ;
#13443=AXIS2_PLACEMENT_3D ( 'NONE', #10587, #20367, #33389 ) ;
#13445=CARTESIAN_POINT ( 'NONE',  ( -24.23745918283205114, 82.38670122043342303, -1.270000000000006457 ) ) ;
#13457=CARTESIAN_POINT ( 'NONE',  ( -4.476425760464393555, 71.61790547347303004, 1.270000000000004903 ) ) ;
#13462=FACE_OUTER_BOUND ( 'NONE', #16109, .T. ) ;
#13463=EDGE_LOOP ( 'NONE', ( #21621, #1657, #32103, #28403 ) ) ;
#13464=DIRECTION ( 'NONE',  ( -0.9454731675810352787, 0.3256999990547799206, -7.420046207093943154E-15 ) ) ;
#13470=ADVANCED_FACE ( 'NONE', ( #23856 ), #33613, .T. ) ;
#13472=CARTESIAN_POINT ( 'NONE',  ( -58.80888331074255859, -0.2806509898663787084, -0.1196884892477749346 ) ) ;
#13474=CARTESIAN_POINT ( 'NONE',  ( -58.35474420885217484, -0.2600319066113354616, -0.1537082109189478740 ) ) ;
#13479=EDGE_CURVE ( 'NONE', #702, #25607, #11154, .T. ) ;
#13482=CARTESIAN_POINT ( 'NONE',  ( -57.36719850051837000, 1.975114663830185302, -1.756955940785672077 ) ) ;
#13491=CIRCLE ( 'NONE', #39337, 0.2539999999999937863 ) ;
#13492=CARTESIAN_POINT ( 'NONE',  ( -57.83370854706706865, 0.8645507274500086048, 1.063039573801799031 ) ) ;
#13498=CARTESIAN_POINT ( 'NONE',  ( -7.921807157844598102, 72.80702234259206307, -1.269999999999996243 ) ) ;
#13499=CARTESIAN_POINT ( 'NONE',  ( -54.02436534585504546, 7.965282956745534548, -1.622780670314687868 ) ) ;
#13502=DIRECTION ( 'NONE',  ( 0.8745520943968249084, -0.4849315768086534528, 5.361993529360573944E-16 ) ) ;
#13504=DIRECTION ( 'NONE',  ( 5.188838149069472160E-16, -1.699382548006136559E-16, -1.000000000000000000 ) ) ;
#13507=DIRECTION ( 'NONE',  ( 5.188838149069472160E-16, -1.699382548006136559E-16, -1.000000000000000000 ) ) ;
#13508=CARTESIAN_POINT ( 'NONE',  ( -57.66243511465492588, 3.255537196535582378, 0.1194500880619485950 ) ) ;
#13509=CARTESIAN_POINT ( 'NONE',  ( -56.04137470801128273, 5.508142037592367757, 2.879222540163115074 ) ) ;
#13511=ORIENTED_EDGE ( 'NONE', *, *, #33709, .T. ) ;
#13512=CARTESIAN_POINT ( 'NONE',  ( -53.18864123405685262, 14.74122628988702743, -1.932938280191028202 ) ) ;
#13514=AXIS2_PLACEMENT_3D ( 'NONE', #7534, #1780, #34359 ) ;
#13515=ORIENTED_EDGE ( 'NONE', *, *, #37950, .F. ) ;
#13518=AXIS2_PLACEMENT_3D ( 'NONE', #128, #42089, #13306 ) ;
#13523=CARTESIAN_POINT ( 'NONE',  ( -30.15519950990045572, 69.97033940222175374, 1.269999999999991802 ) ) ;
#13527=DIRECTION ( 'NONE',  ( 5.188838149069472160E-16, -1.699382548006136559E-16, -1.000000000000000000 ) ) ;
#13532=CARTESIAN_POINT ( 'NONE',  ( -57.71595586907567821, 1.118948197508295328, -1.187837037485634628 ) ) ;
#13546=CARTESIAN_POINT ( 'NONE',  ( -45.82931853585289872, 22.14969803457954356, -3.600065900675656128 ) ) ;
#13556=CARTESIAN_POINT ( 'NONE',  ( -46.33290834485746501, 20.59977736898093070, -4.631597800898671125 ) ) ;
#13557=ORIENTED_EDGE ( 'NONE', *, *, #12649, .T. ) ;
#13568=EDGE_CURVE ( 'NONE', #4125, #120, #18621, .T. ) ;
#13586=CARTESIAN_POINT ( 'NONE',  ( -4.085839532347240066, 71.06758511999679229, -1.523999999999994026 ) ) ;
#13591=CARTESIAN_POINT ( 'NONE',  ( -18.01920641645601151, 83.84822824455467583, 1.523999999999996025 ) ) ;
#13594=EDGE_CURVE ( 'NONE', #35463, #33914, #295, .T. ) ;
#13598=CARTESIAN_POINT ( 'NONE',  ( -50.92517188622475288, 14.59490250589506921, 4.563427635915562774 ) ) ;
#13599=CARTESIAN_POINT ( 'NONE',  ( -47.59569394876871939, 21.45978420380969354, 4.300550031832332643 ) ) ;
#13601=CARTESIAN_POINT ( 'NONE',  ( -53.00789483126595769, 12.40033530745290236, 4.180047681284801975 ) ) ;
#13602=CARTESIAN_POINT ( 'NONE',  ( -58.36929466660706112, 0.2635729057794952701, 0.9100288767555340108 ) ) ;
#13604=CARTESIAN_POINT ( 'NONE',  ( -58.11144429832071268, 0.1746852717545849254, -0.04262357901410007005 ) ) ;
#13607=CARTESIAN_POINT ( 'NONE',  ( -47.00787117332040310, 24.49876931072293829, 2.333946431867817584 ) ) ;
#13613=( NAMED_UNIT ( * ) SI_UNIT ( $, .STERADIAN. ) SOLID_ANGLE_UNIT ( ) );
#13622=DIRECTION ( 'NONE',  ( 5.188838149069472160E-16, -1.699382548006136559E-16, -1.000000000000000000 ) ) ;
#13628=ORIENTED_EDGE ( 'NONE', *, *, #13329, .F. ) ;
#13629=EDGE_CURVE ( 'NONE', #25488, #41561, #37080, .T. ) ;
#13630=CARTESIAN_POINT ( 'NONE',  ( -44.35420297070785978, 19.68308750433651966, 0.4327882352162311097 ) ) ;
#13641=EDGE_CURVE ( 'NONE', #1503, #34270, #41761, .T. ) ;
#13646=DIRECTION ( 'NONE',  ( 0.1906721105965186736, -0.9816537812491066273, 0.000000000000000000 ) ) ;
#13651=EDGE_CURVE ( 'NONE', #26382, #5996, #27687, .T. ) ;
#13664=CARTESIAN_POINT ( 'NONE',  ( -33.20758249455312239, 49.81222039523557044, 1.269999999999993578 ) ) ;
#13670=CARTESIAN_POINT ( 'NONE',  ( -26.29578028364076658, 73.87584665086983193, 1.523999999999993360 ) ) ;
#13679=CARTESIAN_POINT ( 'NONE',  ( -58.60178378695536594, -0.2365438316893033466, -0.4554716356075824701 ) ) ;
#13680=ORIENTED_EDGE ( 'NONE', *, *, #37416, .T. ) ;
#13686=DIRECTION ( 'NONE',  ( -5.188838149069472160E-16, 1.699382548006136559E-16, 1.000000000000000000 ) ) ;
#13690=FACE_OUTER_BOUND ( 'NONE', #40974, .T. ) ;
#13695=VERTEX_POINT ( 'NONE', #33470 ) ;
#13697=CARTESIAN_POINT ( 'NONE',  ( -26.51793118801306548, 72.98537704160715123, 1.523999999999993360 ) ) ;
#13698=CARTESIAN_POINT ( 'NONE',  ( -58.31060438690772685, -0.1666892599193892099, 0.3090539641401659487 ) ) ;
#13703=EDGE_CURVE ( 'NONE', #40718, #25505, #23639, .T. ) ;
#13707=CARTESIAN_POINT ( 'NONE',  ( -55.77633192430580777, 4.649224570933515821, -0.8844362032702758336 ) ) ;
#13711=FACE_OUTER_BOUND ( 'NONE', #21682, .T. ) ;
#13715=DIRECTION ( 'NONE',  ( 0.4849315768086480127, 0.8745520943968279060, 1.030032898892941415E-16 ) ) ;
#13716=CARTESIAN_POINT ( 'NONE',  ( -58.62011547798931588, 0.4741971735572336755, 0.2911429440373402566 ) ) ;
#13717=CARTESIAN_POINT ( 'NONE',  ( -58.30521585032268206, -0.1116666926106041347, 0.6575736669891736330 ) ) ;
#13719=ORIENTED_EDGE ( 'NONE', *, *, #17931, .T. ) ;
#13720=CARTESIAN_POINT ( 'NONE',  ( -57.67985703563598321, 3.143487229238031588, -0.2637475255842378630 ) ) ;
#13731=FACE_OUTER_BOUND ( 'NONE', #4336, .T. ) ;
#13736=VERTEX_POINT ( 'NONE', #24068 ) ;
#13739=CARTESIAN_POINT ( 'NONE',  ( -57.59849520485223451, 1.372415327657551032, -1.305467049941703594 ) ) ;
#13746=DIRECTION ( 'NONE',  ( -0.2290273297124634233, 0.9734199927291296017, -2.580167833703404029E-15 ) ) ;
#13749=EDGE_LOOP ( 'NONE', ( #40805, #14918, #27352, #866 ) ) ;
#13754=CARTESIAN_POINT ( 'NONE',  ( -56.80697847991661575, 4.636179106009441497, -2.484889565616585472 ) ) ;
#13763=EDGE_LOOP ( 'NONE', ( #18117, #30983, #22892, #16904 ) ) ;
#13767=ORIENTED_EDGE ( 'NONE', *, *, #41740, .T. ) ;
#13769=CARTESIAN_POINT ( 'NONE',  ( -46.96231544241639710, 24.98353995950039419, -1.991484372665529579 ) ) ;
#13770=ORIENTED_EDGE ( 'NONE', *, *, #38572, .F. ) ;
#13779=CARTESIAN_POINT ( 'NONE',  ( -41.34500286397576474, 23.15616463071227571, -1.524000640040308330 ) ) ;
#13785=CARTESIAN_POINT ( 'NONE',  ( -58.50248613192575675, -0.02569321026361925941, -0.6864972099078561207 ) ) ;
#13786=CARTESIAN_POINT ( 'NONE',  ( -17.09698261757901960, 84.43312239790384410, 1.269999999999996243 ) ) ;
#13793=FACE_OUTER_BOUND ( 'NONE', #27294, .T. ) ;
#13796=ORIENTED_EDGE ( 'NONE', *, *, #18928, .F. ) ;
#13804=CARTESIAN_POINT ( 'NONE',  ( -19.15923810799328209, 79.68098548105338352, 1.269999999999995799 ) ) ;
#13805=CIRCLE ( 'NONE', #24683, 0.2540000000000062208 ) ;
#13808=CARTESIAN_POINT ( 'NONE',  ( -57.03986430441516831, 2.569584422222054076, 1.777618630297834734 ) ) ;
#13809=CARTESIAN_POINT ( 'NONE',  ( -47.99025707952957021, 21.67807857130912907, 3.596429695783027292 ) ) ;
#13811=CARTESIAN_POINT ( 'NONE',  ( -52.26939619200407350, 13.58078015197115818, 4.476849201000069556 ) ) ;
#13812=CARTESIAN_POINT ( 'NONE',  ( -58.62105023224247446, -0.2745841218223041280, 0.4015347698698587542 ) ) ;
#13814=ORIENTED_EDGE ( 'NONE', *, *, #31398, .F. ) ;
#13815=CARTESIAN_POINT ( 'NONE',  ( -46.81005371095109524, 25.73327194510133253, 1.583310528698471664 ) ) ;
#13818=VECTOR ( 'NONE', #39390, 1000.000000000000114 ) ;
#13830=CARTESIAN_POINT ( 'NONE',  ( -3.909619041219700719, 60.89059347946586342, 1.524000000000007349 ) ) ;
#13837=AXIS2_PLACEMENT_3D ( 'NONE', #26381, #30000, #35979 ) ;
#13839=ORIENTED_EDGE ( 'NONE', *, *, #9963, .F. ) ;
#13840=CARTESIAN_POINT ( 'NONE',  ( -47.14728576169839869, 19.79714445405676670, 4.666695388795770505 ) ) ;
#13850=EDGE_LOOP ( 'NONE', ( #15224, #29274, #36132, #19906 ) ) ;
#13853=CIRCLE ( 'NONE', #32936, 0.2539999999999992819 ) ;
#13860=AXIS2_PLACEMENT_3D ( 'NONE', #7483, #17670, #8306 ) ;
#13866=EDGE_LOOP ( 'NONE', ( #9461, #38640, #5442, #20723 ) ) ;
#13872=DIRECTION ( 'NONE',  ( 0.8745520943968249084, -0.4849315768086533418, 5.271987356194193006E-16 ) ) ;
#13875=DIRECTION ( 'NONE',  ( -5.188838149069471174E-16, 1.699382548006136313E-16, 1.000000000000000000 ) ) ;
#13882=ORIENTED_EDGE ( 'NONE', *, *, #13113, .F. ) ;
#13884=VECTOR ( 'NONE', #41118, 1000.000000000000114 ) ;
#13888=EDGE_CURVE ( 'NONE', #14753, #18130, #17263, .T. ) ;
#13889=ORIENTED_EDGE ( 'NONE', *, *, #40979, .F. ) ;
#13897=DIRECTION ( 'NONE',  ( 0.6294287539884068083, 0.7770581983690809658, 1.945484789722802745E-16 ) ) ;
#13898=EDGE_CURVE ( 'NONE', #41432, #22599, #31935, .T. ) ;
#13905=CARTESIAN_POINT ( 'NONE',  ( -52.79140191244064084, 11.19429870258845128, 3.959798436812983713 ) ) ;
#13912=CARTESIAN_POINT ( 'NONE',  ( -50.77948459960266092, 12.22376025917672138, -0.7375277020707465825 ) ) ;
#13915=CARTESIAN_POINT ( 'NONE',  ( -12.79279280188647760, 63.69337819391066091, -1.269999999999997353 ) ) ;
#13916=CARTESIAN_POINT ( 'NONE',  ( -29.16381924947294024, 66.91553870234344004, 1.269999999999992024 ) ) ;
#13920=CARTESIAN_POINT ( 'NONE',  ( -58.26284211471887176, 1.387681237079871455, 0.7239480823116738462 ) ) ;
#13923=ADVANCED_FACE ( 'NONE', ( #15525 ), #28732, .F. ) ;
#13925=CARTESIAN_POINT ( 'NONE',  ( -57.78461401849435930, 2.885363594410716992, -0.1114619696582919983 ) ) ;
#13927=ORIENTED_EDGE ( 'NONE', *, *, #33778, .T. ) ;
#13928=DIRECTION ( 'NONE',  ( -0.8745520943968250194, 0.4849315768086532863, -5.361993529360574930E-16 ) ) ;
#13935=CARTESIAN_POINT ( 'NONE',  ( -29.66844284761598871, 68.28155107131718182, 1.269999999999993356 ) ) ;
#13941=CARTESIAN_POINT ( 'NONE',  ( -58.08011890042329384, 0.3308434713582167341, -0.7480479229743117742 ) ) ;
#13946=CARTESIAN_POINT ( 'NONE',  ( -46.31144060707497090, 24.05480373873685451, -2.308638262703932575 ) ) ;
#13951=VERTEX_POINT ( 'NONE', #41744 ) ;
#13956=CARTESIAN_POINT ( 'NONE',  ( -54.12303657725384198, 9.464413707472848714, -3.807237671326768602 ) ) ;
#13957=DIRECTION ( 'NONE',  ( -5.188838149069472160E-16, 1.699382548006136559E-16, 1.000000000000000000 ) ) ;
#13968=CARTESIAN_POINT ( 'NONE',  ( -48.36699572807423664, 24.50126085711046997, -0.4363764532069382973 ) ) ;
#13971=ORIENTED_EDGE ( 'NONE', *, *, #633, .F. ) ;
#13972=CARTESIAN_POINT ( 'NONE',  ( -26.03112572612057818, 72.30369090346633243, 1.269999999999993578 ) ) ;
#13976=DIRECTION ( 'NONE',  ( -0.9816537812491126225, -0.1906721105964872265, -8.537024980200846470E-16 ) ) ;
#13978=VERTEX_POINT ( 'NONE', #28099 ) ;
#13981=DIRECTION ( 'NONE',  ( -0.8745520943968235761, 0.4849315768086558398, -4.268512490100410909E-16 ) ) ;
#13982=CARTESIAN_POINT ( 'NONE',  ( -19.15923810799328209, 79.68098548105338352, 1.523999999999996025 ) ) ;
#13983=VERTEX_POINT ( 'NONE', #9352 ) ;
#13985=ADVANCED_FACE ( 'NONE', ( #11917 ), #12546, .T. ) ;
#13988=CARTESIAN_POINT ( 'NONE',  ( -57.93805369095603197, 0.6893004133203329831, -1.202053765808154040 ) ) ;
#13993=ORIENTED_EDGE ( 'NONE', *, *, #41474, .F. ) ;
#13996=CYLINDRICAL_SURFACE ( 'NONE', #17920, 0.5080000000000000071 ) ;
#14009=CARTESIAN_POINT ( 'NONE',  ( -53.46379006321816973, 9.876576013476611848, 3.680876057010925795 ) ) ;
#14010=CARTESIAN_POINT ( 'NONE',  ( -49.18824384045164777, 22.20099125052343680, 1.469723468883180173 ) ) ;
#14011=CARTESIAN_POINT ( 'NONE',  ( -49.19743978460682143, 17.65503563884207594, 5.190924102448284394 ) ) ;
#14012=CARTESIAN_POINT ( 'NONE',  ( -58.60445817883077524, -0.2419304147805778904, 0.4480943822351404759 ) ) ;
#14017=CARTESIAN_POINT ( 'NONE',  ( -45.67973391888839529, 25.66060799623228661, 1.523999999999991806 ) ) ;
#14028=CARTESIAN_POINT ( 'NONE',  ( -47.84756666395249880, 19.38928433903623016, 5.209054514891913179 ) ) ;
#14029=VECTOR ( 'NONE', #25845, 1000.000000000000000 ) ;
#14033=DIRECTION ( 'NONE',  ( 5.188838149069472160E-16, -1.699382548006136559E-16, -1.000000000000000000 ) ) ;
#14043=CARTESIAN_POINT ( 'NONE',  ( -49.65974013515536711, 15.91765330076391116, 3.790917083309703006 ) ) ;
#14049=ORIENTED_EDGE ( 'NONE', *, *, #41455, .T. ) ;
#14059=CARTESIAN_POINT ( 'NONE',  ( -5.924740142096584172, 65.21691166894066782, -1.523999999999994026 ) ) ;
#14062=CARTESIAN_POINT ( 'NONE',  ( -7.772068811996249771, 69.25462295839062676, -1.269999999999995577 ) ) ;
#14064=CARTESIAN_POINT ( 'NONE',  ( -8.095114962461808616, 74.19100168833409725, -1.269999999999996687 ) ) ;
#14067=EDGE_LOOP ( 'NONE', ( #19442, #5279, #40268, #24671 ) ) ;
#14074=TOROIDAL_SURFACE ( 'NONE', #30403, 8.794749999999998735, 0.2540000000000000036 ) ;
#14081=EDGE_CURVE ( 'NONE', #22433, #22644, #8459, .T. ) ;
#14083=CARTESIAN_POINT ( 'NONE',  ( -22.95370498042275642, 82.54569470718179502, -1.270000000000005791 ) ) ;
#14086=DIRECTION ( 'NONE',  ( -0.8745520943968235761, 0.4849315768086558953, -5.361993529360570985E-16 ) ) ;
#14093=CIRCLE ( 'NONE', #35880, 0.5079999999999984528 ) ;
#14096=CARTESIAN_POINT ( 'NONE',  ( -46.58415294817042707, 20.65776983473033823, 4.869103127773887429 ) ) ;
#14099=CARTESIAN_POINT ( 'NONE',  ( -19.33375693323417366, 80.42273151551299293, 1.269999999999995577 ) ) ;
#14103=ORIENTED_EDGE ( 'NONE', *, *, #22477, .T. ) ;
#14106=CARTESIAN_POINT ( 'NONE',  ( -58.14608079600216684, 0.1881903270890411539, 0.6509722733310221443 ) ) ;
#14116=VECTOR ( 'NONE', #30071, 1000.000000000000114 ) ;
#14117=CARTESIAN_POINT ( 'NONE',  ( -54.22787649382025421, 6.886497292746610377, -9.681224659302749425E-15 ) ) ;
#14119=CARTESIAN_POINT ( 'NONE',  ( -29.30569680504977370, 61.36914094216600546, -1.270000000000005347 ) ) ;
#14123=CARTESIAN_POINT ( 'NONE',  ( -58.33482727260577860, 1.278009831242016281, 0.06942977984275174042 ) ) ;
#14127=CARTESIAN_POINT ( 'NONE',  ( -56.90576330281450623, 4.524090327013369439, -2.207515467630546180 ) ) ;
#14130=CARTESIAN_POINT ( 'NONE',  ( -47.85244527695899563, 19.39403540832956807, -5.219971639306755229 ) ) ;
#14141=ORIENTED_EDGE ( 'NONE', *, *, #12821, .F. ) ;
#14144=CARTESIAN_POINT ( 'NONE',  ( -58.30215177840349128, -0.1486083857870257596, -0.3315235503724106580 ) ) ;
#14148=CARTESIAN_POINT ( 'NONE',  ( -47.20791569504334717, 21.28685671521062517, -4.803936552638846891 ) ) ;
#14152=ORIENTED_EDGE ( 'NONE', *, *, #17533, .F. ) ;
#14157=CARTESIAN_POINT ( 'NONE',  ( -50.78166962549567387, 16.07998339508975860, -4.893817234114181680 ) ) ;
#14158=EDGE_CURVE ( 'NONE', #41143, #27874, #39765, .T. ) ;
#14167=DIRECTION ( 'NONE',  ( 0.7770581983690878491, -0.6294287539883980376, 5.101669463485847584E-16 ) ) ;
#14170=CARTESIAN_POINT ( 'NONE',  ( -57.34787435976329562, 1.552391619547732748, 0.09937746155959813199 ) ) ;
#14172=VERTEX_POINT ( 'NONE', #38746 ) ;
#14173=CARTESIAN_POINT ( 'NONE',  ( -47.63491852694408379, 24.04202919463459409, -1.290898778641178080 ) ) ;
#14176=VERTEX_POINT ( 'NONE', #32777 ) ;
#14177=CARTESIAN_POINT ( 'NONE',  ( -17.14500000000466784, 71.11999999999886768, 1.269999999999998241 ) ) ;
#14180=AXIS2_PLACEMENT_3D ( 'NONE', #27284, #36251, #26440 ) ;
#14184=ORIENTED_EDGE ( 'NONE', *, *, #8919, .T. ) ;
#14193=CARTESIAN_POINT ( 'NONE',  ( -58.22785051087659980, 0.5684335961349124000, -1.101539904998067865 ) ) ;
#14197=ORIENTED_EDGE ( 'NONE', *, *, #33778, .F. ) ;
#14202=CARTESIAN_POINT ( 'NONE',  ( -47.59458007651505795, 19.66657808744504976, 5.176039278149815459 ) ) ;
#14207=FACE_OUTER_BOUND ( 'NONE', #41288, .T. ) ;
#14213=CARTESIAN_POINT ( 'NONE',  ( -57.20840289379589905, 2.209747822858734612, 1.646108566719461042 ) ) ;
#14216=CARTESIAN_POINT ( 'NONE',  ( -57.85534701229748578, 0.8496279762696679061, 1.203237356453206619 ) ) ;
#14217=CARTESIAN_POINT ( 'NONE',  ( -57.60391329870441979, 1.913983619093638122, 1.729326818512549657 ) ) ;
#14221=CARTESIAN_POINT ( 'NONE',  ( -43.10982161678889213, 22.52422253607401359, 1.888110242252979631 ) ) ;
#14222=TOROIDAL_SURFACE ( 'NONE', #2668, 8.794749999999996959, 0.2540000000000000036 ) ;
#14224=CIRCLE ( 'NONE', #16255, 0.7620000000000015650 ) ;
#14232=B_SPLINE_CURVE_WITH_KNOTS ( 'NONE', 3,
 ( #29050, #22844, #19877, #22635, #13286, #32042, #35456, #26271, #2879, #26062, #29686, #41861, #6278, #42068, #16047, #39072, #12864, #25850, #6694, #19663, #29477, #319, #36092, #30521, #4562, #4358, #17725, #20081, #20498, #27117, #14319, #37133, #16894, #17521, #10511, #39710, #33104, #33525, #20922 ),
 .UNSPECIFIED., .F., .F.,
 ( 4, 2, 1, 1, 1, 2, 2, 2, 2, 1, 1, 2, 2, 2, 2, 1, 2, 2, 2, 1, 2, 2, 4 ),
 ( 0.000000000000000000, 0.06250000000019394208, 0.09375000000028790859, 0.1093750000003349682, 0.1171875000003639727, 0.1210937500003731876, 0.1250000000003823886, 0.1875000000005171974, 0.2187500000005817291, 0.2343750000006132317, 0.2421875000006274425, 0.2460937500006222522, 0.2500000000006170620, 0.3750000000004883871, 0.4375000000004232170, 0.4687500000003906320, 0.4843750000003776979, 0.5000000000003647083, 0.6250000000002644551, 0.6875000000002159384, 0.7187500000001945111, 0.7500000000001730838, 1.000000000000000000 ),
 .UNSPECIFIED. ) ;
#14234=CARTESIAN_POINT ( 'NONE',  ( -30.28638171898572651, 70.19821000523995735, 1.269999999999990692 ) ) ;
#14237=LINE ( 'NONE', #11258, #10263 ) ;
#14246=CARTESIAN_POINT ( 'NONE',  ( -50.02669608763527265, 12.78473261814652773, 0.3947048150275107581 ) ) ;
#14256=VECTOR ( 'NONE', #6736, 1000.000000000000114 ) ;
#14259=CIRCLE ( 'NONE', #38080, 0.2539999999999956737 ) ;
#14276=FACE_OUTER_BOUND ( 'NONE', #2068, .T. ) ;
#14278=DIRECTION ( 'NONE',  ( -0.8745520943968243532, 0.4849315768086547296, -5.361993529360573944E-16 ) ) ;
#14284=LINE ( 'NONE', #17068, #14116 ) ;
#14290=ORIENTED_EDGE ( 'NONE', *, *, #1206, .T. ) ;
#14291=ORIENTED_EDGE ( 'NONE', *, *, #13479, .F. ) ;
#14303=AXIS2_PLACEMENT_3D ( 'NONE', #27890, #37077, #11285 ) ;
#14305=CARTESIAN_POINT ( 'NONE',  ( -57.45676042279916373, 1.677525466756688122, 1.437765377952616275 ) ) ;
#14310=CIRCLE ( 'NONE', #8950, 0.3810000000000015041 ) ;
#14316=CARTESIAN_POINT ( 'NONE',  ( -55.10067240196883631, 5.634149028679341420, -0.4880682687716038637 ) ) ;
#14319=CARTESIAN_POINT ( 'NONE',  ( -46.87659121548133356, 25.47535466239702728, -1.649981827335061713 ) ) ;
#14321=PLANE ( 'NONE',  #11356 ) ;
#14322=VECTOR ( 'NONE', #28455, 1000.000000000000000 ) ;
#14324=FACE_OUTER_BOUND ( 'NONE', #31158, .T. ) ;
#14325=CARTESIAN_POINT ( 'NONE',  ( -58.80872392184672037, -0.02106340533553074934, 0.1867271868312104510 ) ) ;
#14329=CARTESIAN_POINT ( 'NONE',  ( -58.10740272659374739, 1.828491270143103975, -0.5949618876680415891 ) ) ;
#14331=VERTEX_POINT ( 'NONE', #1462 ) ;
#14332=CARTESIAN_POINT ( 'NONE',  ( -46.36020037344893296, 20.58642004076050469, -4.649377256145048598 ) ) ;
#14333=AXIS2_PLACEMENT_3D ( 'NONE', #17042, #34092, #33677 ) ;
#14339=CARTESIAN_POINT ( 'NONE',  ( -30.84347056137454146, 55.46442681907723937, 1.269999999999994023 ) ) ;
#14341=CARTESIAN_POINT ( 'NONE',  ( -48.86598066419526276, 18.03485269033233607, -5.140156453303863948 ) ) ;
#14345=CARTESIAN_POINT ( 'NONE',  ( -58.03609167196196239, 0.4261842582088196107, -0.8102809492608903374 ) ) ;
#14349=CARTESIAN_POINT ( 'NONE',  ( -43.10982161678889213, 22.52422253607401359, -1.888110242252992066 ) ) ;
#14350=EDGE_CURVE ( 'NONE', #26023, #10127, #10394, .T. ) ;
#14356=DIRECTION ( 'NONE',  ( 0.8745520943968235761, -0.4849315768086558398, 0.000000000000000000 ) ) ;
#14359=CARTESIAN_POINT ( 'NONE',  ( -54.97180548219925100, 8.422794459035404913, -3.467293221275798309 ) ) ;
#14372=CARTESIAN_POINT ( 'NONE',  ( -57.97703582661664967, 0.5002880090035632943, 0.5798895178195145883 ) ) ;
#14373=EDGE_CURVE ( 'NONE', #22759, #30888, #8358, .T. ) ;
#14375=ORIENTED_EDGE ( 'NONE', *, *, #11343, .F. ) ;
#14376=CARTESIAN_POINT ( 'NONE',  ( -46.72388148998840762, 26.09838203902186393, -9.431828030254277901E-15 ) ) ;
#14378=CARTESIAN_POINT ( 'NONE',  ( -17.64950171984354199, 84.16951713491046405, 1.523999999999996247 ) ) ;
#14383=AXIS2_PLACEMENT_3D ( 'NONE', #10416, #36204, #3839 ) ;
#14385=CARTESIAN_POINT ( 'NONE',  ( -41.06677624538416183, 23.07857903911245501, 1.524000000000167221 ) ) ;
#14392=AXIS2_PLACEMENT_3D ( 'NONE', #916, #36062, #26244 ) ;
#14393=CARTESIAN_POINT ( 'NONE',  ( -41.25198945386213722, 23.25239630053127016, -1.523999999999987587 ) ) ;
#14399=CARTESIAN_POINT ( 'NONE',  ( -58.41257333834580834, 0.1697474083101613296, -0.8453419536803969958 ) ) ;
#14403=EDGE_CURVE ( 'NONE', #10127, #38754, #30141, .T. ) ;
#14414=CARTESIAN_POINT ( 'NONE',  ( -29.50088714511802834, 67.43771171077483473, -1.270000000000005569 ) ) ;
#14419=DIRECTION ( 'NONE',  ( -0.1565721916418034432, -0.9876665170007953298, 8.659954811667511346E-17 ) ) ;
#14422=CARTESIAN_POINT ( 'NONE',  ( -57.77486378051489169, 0.9916650371046533685, 1.126111947105124189 ) ) ;
#14424=CARTESIAN_POINT ( 'NONE',  ( -58.33777482027510786, 1.113448835244251756, 1.208045587469420701 ) ) ;
#14425=CARTESIAN_POINT ( 'NONE',  ( -58.62423747511084571, -0.2805004185027809571, 0.3924598736681575439 ) ) ;
#14429=CARTESIAN_POINT ( 'NONE',  ( -48.53848336910535011, 19.22582880449973075, 5.323527254358031868 ) ) ;
#14434=( LENGTH_UNIT ( ) NAMED_UNIT ( * ) SI_UNIT ( .MILLI., .METRE. ) );
#14436=ORIENTED_EDGE ( 'NONE', *, *, #13568, .T. ) ;
#14439=CARTESIAN_POINT ( 'NONE',  ( -41.05193670661653016, 23.09446788613700363, -1.270000000071892066 ) ) ;
#14440=CARTESIAN_POINT ( 'NONE',  ( -44.18728704178793265, 21.36917510656546781, 3.097942224162542058 ) ) ;
#14444=DIRECTION ( 'NONE',  ( -0.9454731675810330582, 0.3256999990547865265, -7.568290090144850389E-15 ) ) ;
#14454=ORIENTED_EDGE ( 'NONE', *, *, #25944, .F. ) ;
#14455=CARTESIAN_POINT ( 'NONE',  ( -51.26804087848103819, 14.04722136430348201, 4.535752393750700939 ) ) ;
#14459=ORIENTED_EDGE ( 'NONE', *, *, #19393, .T. ) ;
#14461=ADVANCED_FACE ( 'NONE', ( #17618 ), #25362, .T. ) ;
#14467=VERTEX_POINT ( 'NONE', #33412 ) ;
#14472=LINE ( 'NONE', #40693, #29978 ) ;
#14478=CARTESIAN_POINT ( 'NONE',  ( -21.32888081312385253, 55.91420173801096638, 1.523999999999999133 ) ) ;
#14480=VERTEX_POINT ( 'NONE', #10817 ) ;
#14488=FACE_OUTER_BOUND ( 'NONE', #30843, .T. ) ;
#14494=VERTEX_POINT ( 'NONE', #27221 ) ;
#14499=ORIENTED_EDGE ( 'NONE', *, *, #39197, .T. ) ;
#14506=EDGE_CURVE ( 'NONE', #25488, #2275, #234, .T. ) ;
#14509=AXIS2_PLACEMENT_3D ( 'NONE', #2528, #41286, #28063 ) ;
#14515=AXIS2_PLACEMENT_3D ( 'NONE', #8874, #11221, #11640 ) ;
#14517=ORIENTED_EDGE ( 'NONE', *, *, #11052, .F. ) ;
#14520=VECTOR ( 'NONE', #14786, 1000.000000000000227 ) ;
#14521=CARTESIAN_POINT ( 'NONE',  ( -58.45640570440981065, -0.4407481023139777632, 0.3169051027096812523 ) ) ;
#14530=CARTESIAN_POINT ( 'NONE',  ( -57.66977034847604955, 1.126272260461025354, -0.8071799157849589568 ) ) ;
#14533=CIRCLE ( 'NONE', #7057, 0.2539999999999973390 ) ;
#14534=DIRECTION ( 'NONE',  ( -0.8745520943968250194, 0.4849315768086532863, -5.361993529360574930E-16 ) ) ;
#14536=DIRECTION ( 'NONE',  ( -0.8745520943968344563, 0.4849315768086362999, -6.829619984160689601E-16 ) ) ;
#14539=FACE_OUTER_BOUND ( 'NONE', #6992, .T. ) ;
#14544=CARTESIAN_POINT ( 'NONE',  ( -57.66243511465492588, 3.255537196535582378, -0.1194500880619697308 ) ) ;
#14550=AXIS2_PLACEMENT_3D ( 'NONE', #2913, #22460, #15875 ) ;
#14554=CARTESIAN_POINT ( 'NONE',  ( -53.52914546082846670, 10.14270320506335210, -3.905849526455717147 ) ) ;
#14558=CARTESIAN_POINT ( 'NONE',  ( -51.17288806236419418, 14.15688068541630429, -4.489013846348126613 ) ) ;
#14563=CARTESIAN_POINT ( 'NONE',  ( -42.33919149967392315, 22.05006338260229271, -1.842566675324098568 ) ) ;
#14565=ORIENTED_EDGE ( 'NONE', *, *, #30470, .F. ) ;
#14570=CARTESIAN_POINT ( 'NONE',  ( -56.78650302187183740, 3.241477563879227475, -2.205756828360271093 ) ) ;
#14578=FACE_OUTER_BOUND ( 'NONE', #10313, .T. ) ;
#14581=CARTESIAN_POINT ( 'NONE',  ( -57.60038635073813396, 1.097546858218847898, 0.08229580080364437555 ) ) ;
#14584=CARTESIAN_POINT ( 'NONE',  ( -47.29848140234559395, 25.70219632838243484, -9.636386808203001053E-15 ) ) ;
#14587=ORIENTED_EDGE ( 'NONE', *, *, #24172, .F. ) ;
#14598=CARTESIAN_POINT ( 'NONE',  ( -45.77009211284281776, 21.09669927562158165, -4.287731556584716941 ) ) ;
#14599=EDGE_CURVE ( 'NONE', #34680, #16326, #37607, .T. ) ;
#14601=DIRECTION ( 'NONE',  ( -5.188838149069471174E-16, 1.699382548006136313E-16, 1.000000000000000000 ) ) ;
#14602=ORIENTED_EDGE ( 'NONE', *, *, #37416, .F. ) ;
#14606=CARTESIAN_POINT ( 'NONE',  ( -58.54549369845722850, -0.1193337916018388789, -0.6006683616744088461 ) ) ;
#14611=EDGE_CURVE ( 'NONE', #21468, #27342, #19937, .T. ) ;
#14612=EDGE_LOOP ( 'NONE', ( #18673, #41522, #16768, #9442, #26471 ) ) ;
#14615=LINE ( 'NONE', #34032, #39719 ) ;
#14617=ADVANCED_FACE ( 'NONE', ( #12292 ), #27843, .F. ) ;
#14619=B_SPLINE_SURFACE_WITH_KNOTS ( 'NONE', 3, 3, ( 
 ( #14683, #5137, #18088, #31093, #14892 ),
 ( #27894, #40902, #3179, #15731, #32145 ),
 ( #28736, #6375, #35345, #38750, #32558 ),
 ( #35765, #22315, #16143, #15529, #8942 ),
 ( #29145, #12958, #18716, #28533, #21907 ),
 ( #2570, #6582, #2775, #19141, #2977 ),
 ( #9155, #35559, #12132, #34937, #12550 ),
 ( #5763, #19548, #31725, #25540, #41539 ),
 ( #19345, #25741, #12346, #18929, #32352 ),
 ( #15314, #41954, #28319, #41329, #25123 ),
 ( #38125, #41749, #25335, #25952, #9770 ),
 ( #15941, #38959, #22734, #38541, #6172 ),
 ( #28936, #9356, #38337, #12755, #22112 ),
 ( #35141, #5968, #31939, #22318, #9559 ),
 ( #22530, #23157, #13389, #16791, #1048 ),
 ( #3611, #14011, #27018, #36823, #26809 ),
 ( #7641, #10610, #7433, #39385, #23803 ),
 ( #10820, #20600, #9975, #36193, #26376 ),
 ( #40027, #3393, #16574, #16359, #39600 ),
 ( #7014, #29365, #32781, #13811, #23592 ),
 ( #29792, #39817, #36614, #20391, #13601 ),
 ( #29585, #419, #13179, #26591, #204 ),
 ( #26166, #33417, #4248, #10187, #10403 ),
 ( #39168, #19759, #19982, #33211, #32999 ),
 ( #631, #23375, #17210, #3827, #36408 ),
 ( #7226, #30208, #20185, #4036, #22949 ),
 ( #35975, #16997, #6792, #29997, #836 ),
 ( #15426, #9262, #1467, #12454, #18829 ),
 ( #33837, #27225, #15213, #22017, #31834 ),
 ( #4665, #40238, #1261, #20811, #25448 ),
 ( #34046, #31625, #28427, #8839, #38446 ),
 ( #31410, #41435, #24014, #33631, #11033 ),
 ( #37033, #7850, #25232, #2463, #17622 ),
 ( #38236, #4459, #17416, #18619, #30413 ),
 ( #14216, #2251, #30624, #21023, #14424 ),
 ( #28635, #2673, #27431, #40445, #11237 ),
 ( #24221, #12240, #37232, #41222, #9052 ),
 ( #35046, #5867, #28215, #41647, #8050 ),
 ( #21802, #15631, #4876, #18403, #12024 ) ),
 .UNSPECIFIED., .F., .F., .F.,
 ( 4, 1, 1, 1, 1, 1, 1, 1, 1, 1, 1, 2, 1, 1, 1, 1, 1, 1, 1, 1, 1, 1, 1, 1, 1, 1, 1, 1, 1, 1, 1, 1, 1, 1, 1, 4 ),
 ( 4, 1, 4 ),
 ( 0.000000000000000000, 0.01653533301974152367, 0.03307066603948304734, 0.04960599905922460223, 0.06614133207896609468, 0.08267666509870763569, 0.09921199811844919059, 0.1322826641579321894, 0.1653533301974152714, 0.1984239962368983812, 0.2314946622763813522, 0.2645653283158643787, 0.3105299952961229071, 0.3335123287862520880, 0.3564946622763812689, 0.4024593292566397418, 0.4484239962368982702, 0.4943886632171566875, 0.5403533301974150493, 0.5863179971776735222, 0.6322826641579321061, 0.6782473311381906900, 0.7242119981184491628, 0.7701766650987074136, 0.8161413320789658865, 0.8621059990592241373, 0.8735971658042887000, 0.8850883325493537068, 0.8965794992944182695, 0.9080706660394826102, 0.9195618327845473949, 0.9310529995296121797, 0.9425441662746769644, 0.9540353330197415271, 0.9770176665098706525, 1.000000000000000000 ),
 ( 0.000000000000000000, 0.5000000000000000000, 1.000000000000000000 ),
 .UNSPECIFIED. ) ;
#14622=DIRECTION ( 'NONE',  ( 0.3256999990547780333, 0.9454731675810359448, 8.328397965203031669E-18 ) ) ;
#14626=FACE_OUTER_BOUND ( 'NONE', #14612, .T. ) ;
#14629=EDGE_CURVE ( 'NONE', #2316, #41065, #8473, .T. ) ;
#14631=CARTESIAN_POINT ( 'NONE',  ( -57.68540670336199128, 1.184946625668306330, 1.219309026451214306 ) ) ;
#14632=CARTESIAN_POINT ( 'NONE',  ( -54.22048251907422411, 8.823772151126235030, 3.634456437801601325 ) ) ;
#14633=EDGE_CURVE ( 'NONE', #27648, #19349, #29464, .T. ) ;
#14637=CARTESIAN_POINT ( 'NONE',  ( -49.13940628111213016, 17.59503125033257120, 5.062072503518671773 ) ) ;
#14638=EDGE_CURVE ( 'NONE', #32933, #29748, #41696, .T. ) ;
#14643=CARTESIAN_POINT ( 'NONE',  ( -28.95189557068615116, 64.41341631820179714, 1.523999999999993582 ) ) ;
#14648=DIRECTION ( 'NONE',  ( -0.8745520943968244643, 0.4849315768086544520, -4.268512490100399076E-16 ) ) ;
#14662=CARTESIAN_POINT ( 'NONE',  ( -51.32320689156235005, 13.70825103427969438, 4.126761985266667487 ) ) ;
#14667=ORIENTED_EDGE ( 'NONE', *, *, #37313, .F. ) ;
#14673=ORIENTED_EDGE ( 'NONE', *, *, #23185, .F. ) ;
#14681=DIRECTION ( 'NONE',  ( 0.9816537812491107351, 0.1906721105964981344, -6.949828216605166964E-15 ) ) ;
#14683=CARTESIAN_POINT ( 'NONE',  ( -41.05189575270516400, 23.09451173561986081, 1.523999999999992472 ) ) ;
#14686=AXIS2_PLACEMENT_3D ( 'NONE', #6477, #29046, #32461 ) ;
#14696=ADVANCED_FACE ( 'NONE', ( #19299 ), #19935, .T. ) ;
#14697=DIRECTION ( 'NONE',  ( -0.8745520943968243532, 0.4849315768086547296, -6.829619984160642269E-16 ) ) ;
#14708=EDGE_CURVE ( 'NONE', #26023, #33608, #22274, .T. ) ;
#14722=VECTOR ( 'NONE', #40466, 1000.000000000000000 ) ;
#14725=AXIS2_PLACEMENT_3D ( 'NONE', #35245, #3290, #29472 ) ;
#14729=CARTESIAN_POINT ( 'NONE',  ( -58.54486130997005233, -0.6084878433727288760, 0.2286541811371931576 ) ) ;
#14734=AXIS2_PLACEMENT_3D ( 'NONE', #23675, #13897, #17299 ) ;
#14738=CARTESIAN_POINT ( 'NONE',  ( -57.53554607470949378, 1.398951746849091959, -0.8928682508385608063 ) ) ;
#14740=VECTOR ( 'NONE', #10599, 1000.000000000000000 ) ;
#14743=CARTESIAN_POINT ( 'NONE',  ( -17.31000046771894318, 62.32679794340116786, -1.269999999999999352 ) ) ;
#14748=DIRECTION ( 'NONE',  ( 5.188838149069472160E-16, -1.699382548006136559E-16, -1.000000000000000000 ) ) ;
#14749=CARTESIAN_POINT ( 'NONE',  ( -58.83227707057485389, -0.08366279997994163775, -1.544404338758123352E-14 ) ) ;
#14750=CARTESIAN_POINT ( 'NONE',  ( -58.83227707057486811, -0.08366279997995551554, -1.995625700055530397E-14 ) ) ;
#14752=AXIS2_PLACEMENT_3D ( 'NONE', #11978, #8158, #25187 ) ;
#14753=VERTEX_POINT ( 'NONE', #15891 ) ;
#14754=DIRECTION ( 'NONE',  ( -0.8745520943968250194, 0.4849315768086532863, -5.361993529360574930E-16 ) ) ;
#14755=ORIENTED_EDGE ( 'NONE', *, *, #6452, .F. ) ;
#14756=CARTESIAN_POINT ( 'NONE',  ( -43.44488126592453625, 21.78892034651219944, -2.392822157540683836 ) ) ;
#14763=CARTESIAN_POINT ( 'NONE',  ( -50.28518799591763866, 15.83636413734068249, -4.862251023740228995 ) ) ;
#14765=CARTESIAN_POINT ( 'NONE',  ( -10.93398011767285460, 82.89560043784887000, 1.269999999999999574 ) ) ;
#14767=CARTESIAN_POINT ( 'NONE',  ( -53.66072396849355641, 9.491867573702387872, -3.600208096711306816 ) ) ;
#14770=CARTESIAN_POINT ( 'NONE',  ( -47.35944255389382107, 21.37623662739424191, -4.722871667523179440 ) ) ;
#14774=EDGE_LOOP ( 'NONE', ( #4737, #15848, #5162, #15777 ) ) ;
#14778=CARTESIAN_POINT ( 'NONE',  ( -57.83637253161431602, 2.237724655402451024, -1.757929103219309397 ) ) ;
#14779=VECTOR ( 'NONE', #41609, 1000.000000000000114 ) ;
#14780=DIRECTION ( 'NONE',  ( -0.8745520943968245753, 0.4849315768086539524, -5.691349986800526185E-16 ) ) ;
#14785=CARTESIAN_POINT ( 'NONE',  ( -56.80697847991661575, 4.636179106009441497, -2.484889565616585472 ) ) ;
#14786=DIRECTION ( 'NONE',  ( -0.4849315768086534528, -0.8745520943968250194, -1.030032898892974942E-16 ) ) ;
#14791=CARTESIAN_POINT ( 'NONE',  ( -57.48728866487982714, 1.341405240446180702, 0.2210608495301386867 ) ) ;
#14792=CARTESIAN_POINT ( 'NONE',  ( -48.56815661899839398, 19.24492339269599839, 5.224590812749970503 ) ) ;
#14794=ORIENTED_EDGE ( 'NONE', *, *, #8763, .T. ) ;
#14795=CARTESIAN_POINT ( 'NONE',  ( -48.81380759447691275, 19.38479668107215304, -4.754960688114476142 ) ) ;
#14807=FACE_OUTER_BOUND ( 'NONE', #32490, .T. ) ;
#14813=ORIENTED_EDGE ( 'NONE', *, *, #5353, .T. ) ;
#14815=CARTESIAN_POINT ( 'NONE',  ( -9.909999474182706436, 76.95545850745379823, -1.523999999999998023 ) ) ;
#14817=CARTESIAN_POINT ( 'NONE',  ( -57.87993506102255736, 0.7648122704444343389, -1.011066771892038085 ) ) ;
#14822=ORIENTED_EDGE ( 'NONE', *, *, #7655, .T. ) ;
#14828=ORIENTED_EDGE ( 'NONE', *, *, #3265, .F. ) ;
#14831=ADVANCED_FACE ( 'NONE', ( #16739 ), #19716, .T. ) ;
#14838=DIRECTION ( 'NONE',  ( -5.188838149069472160E-16, 1.699382548006136559E-16, 1.000000000000000000 ) ) ;
#14839=CARTESIAN_POINT ( 'NONE',  ( -58.04313065737859745, 0.4109646669389979134, 0.8003343135030365207 ) ) ;
#14840=CARTESIAN_POINT ( 'NONE',  ( -29.02482657613216332, 65.73348897311474559, -1.524000000000006905 ) ) ;
#14846=CARTESIAN_POINT ( 'NONE',  ( -53.00789483126595769, 12.40033530745290236, 4.180047681284801975 ) ) ;
#14852=CARTESIAN_POINT ( 'NONE',  ( -20.79116009376201646, 79.67004825550966984, -1.270000000000004015 ) ) ;
#14857=DIRECTION ( 'NONE',  ( 0.9454731675810332803, -0.3256999990547855828, 8.537024980200802097E-16 ) ) ;
#14858=CARTESIAN_POINT ( 'NONE',  ( -42.18385791109447780, 22.43440044418187185, 1.696665287888085460 ) ) ;
#14859=LINE ( 'NONE', #24447, #5906 ) ;
#14861=VECTOR ( 'NONE', #42067, 1000.000000000000114 ) ;
#14872=ORIENTED_EDGE ( 'NONE', *, *, #29749, .F. ) ;
#14873=CARTESIAN_POINT ( 'NONE',  ( -53.01551111795198068, 8.729259440421092364, 0.3204493394367104453 ) ) ;
#14877=EDGE_LOOP ( 'NONE', ( #40031, #26421, #40601, #6047 ) ) ;
#14886=CARTESIAN_POINT ( 'NONE',  ( -11.05715273818225164, 82.67346420587206524, 1.524000000000000021 ) ) ;
#14889=AXIS2_PLACEMENT_3D ( 'NONE', #40753, #30307, #21125 ) ;
#14892=CARTESIAN_POINT ( 'NONE',  ( -46.60530155212503445, 26.17382724835477958, 1.523999999999991140 ) ) ;
#14903=FACE_OUTER_BOUND ( 'NONE', #27203, .T. ) ;
#14904=CARTESIAN_POINT ( 'NONE',  ( -56.01560174880540188, 6.374421267034191985, 2.942705720416951110 ) ) ;
#14908=EDGE_CURVE ( 'NONE', #37389, #22515, #6126, .T. ) ;
#14918=ORIENTED_EDGE ( 'NONE', *, *, #24523, .T. ) ;
#14919=CIRCLE ( 'NONE', #31247, 0.2540000000000000036 ) ;
#14924=EDGE_CURVE ( 'NONE', #32706, #39773, #36254, .T. ) ;
#14928=AXIS2_PLACEMENT_3D ( 'NONE', #26608, #4054, #17015 ) ;
#14939=CARTESIAN_POINT ( 'NONE',  ( -58.34279097978161133, -0.2008976519008942030, 0.5874393231764968304 ) ) ;
#14949=CARTESIAN_POINT ( 'NONE',  ( -56.90063064090522715, 2.680628813859151194, -1.231466298089203937 ) ) ;
#14951=LINE ( 'NONE', #23694, #27828 ) ;
#14956=CARTESIAN_POINT ( 'NONE',  ( -41.28107547821694112, 23.22158991241130011, 1.523999999999988475 ) ) ;
#14957=CARTESIAN_POINT ( 'NONE',  ( -58.83227707057489653, -0.08366279998001102669, -1.541589583118017482E-14 ) ) ;
#14961=CARTESIAN_POINT ( 'NONE',  ( -58.33777482027512207, 1.113448835244237767, -1.208045587469442017 ) ) ;
#14964=CARTESIAN_POINT ( 'NONE',  ( -4.085839532347240066, 71.06758511999679229, 1.270000000000005125 ) ) ;
#14971=EDGE_CURVE ( 'NONE', #17471, #25107, #24678, .T. ) ;
#14972=CARTESIAN_POINT ( 'NONE',  ( -50.15850345609781158, 16.04140918442848829, -4.890455600740700959 ) ) ;
#14973=ORIENTED_EDGE ( 'NONE', *, *, #27398, .T. ) ;
#14975=CARTESIAN_POINT ( 'NONE',  ( -8.761523658392190939, 74.56051954986229191, 1.524000000000002242 ) ) ;
#14977=CARTESIAN_POINT ( 'NONE',  ( -48.97240568284989592, 17.83076478022523048, -5.072389016522397931 ) ) ;
#14979=AXIS2_PLACEMENT_3D ( 'NONE', #30661, #40484, #37269 ) ;
#14981=CARTESIAN_POINT ( 'NONE',  ( -52.26939619200407350, 13.58078015197115818, -4.476849201000089096 ) ) ;
#14987=EDGE_CURVE ( 'NONE', #20566, #36869, #4587, .T. ) ;
#14989=CARTESIAN_POINT ( 'NONE',  ( -57.69570286664291103, 2.558035660193719529, -1.875687456014384802 ) ) ;
#14997=LINE ( 'NONE', #2249, #14520 ) ;
#15001=DIRECTION ( 'NONE',  ( 0.7770581983690836303, -0.6294287539884032556, 5.101669463485833779E-16 ) ) ;
#15002=CARTESIAN_POINT ( 'NONE',  ( -58.16721443865020547, 0.09938604254088045931, 0.2878065994479881429 ) ) ;
#15003=CARTESIAN_POINT ( 'NONE',  ( -51.09183723991096571, 15.73968240350219538, 4.743875354842988834 ) ) ;
#15006=CARTESIAN_POINT ( 'NONE',  ( -51.38196307734524737, 20.99359796827592817, -0.3730309213897348153 ) ) ;
#15009=ORIENTED_EDGE ( 'NONE', *, *, #4291, .T. ) ;
#15014=CARTESIAN_POINT ( 'NONE',  ( -21.91949108387693457, 59.24500507708427932, -1.270000000000001128 ) ) ;
#15017=LINE ( 'NONE', #34848, #2652 ) ;
#15020=CARTESIAN_POINT ( 'NONE',  ( -17.09258512000246100, 84.17916046765628835, -1.524000000000002908 ) ) ;
#15021=CARTESIAN_POINT ( 'NONE',  ( -8.857543928232141539, 74.53795647042551309, 1.270000000000002016 ) ) ;
#15022=ORIENTED_EDGE ( 'NONE', *, *, #6991, .F. ) ;
#15024=CARTESIAN_POINT ( 'NONE',  ( -14.38915334913366806, 80.27078028363496287, -1.270000000000000906 ) ) ;
#15026=CARTESIAN_POINT ( 'NONE',  ( -57.74058121727584592, 1.065718057878028979, -1.162857118035388160 ) ) ;
#15033=VERTEX_POINT ( 'NONE', #26759 ) ;
#15039=DIRECTION ( 'NONE',  ( -5.188838149069472160E-16, 1.699382548006136066E-16, 1.000000000000000000 ) ) ;
#15048=DIRECTION ( 'NONE',  ( 0.4849315768086426282, 0.8745520943968309036, 1.030032898892908135E-16 ) ) ;
#15049=CARTESIAN_POINT ( 'NONE',  ( -57.97682026406428690, 0.5548386587714120299, 0.8895012536376524226 ) ) ;
#15053=CARTESIAN_POINT ( 'NONE',  ( -21.18564099849817239, 70.71717898851710515, -1.270000000000002682 ) ) ;
#15057=CARTESIAN_POINT ( 'NONE',  ( -54.39768377094780760, 8.094885465611476150, 3.421923752996821833 ) ) ;
#15063=CARTESIAN_POINT ( 'NONE',  ( -6.422645615570758970, 77.88548590848095898, -1.523999999999996469 ) ) ;
#15067=CARTESIAN_POINT ( 'NONE',  ( -32.57684172266954903, 51.47351799184504273, 1.270000000001143992 ) ) ;
#15068=FACE_OUTER_BOUND ( 'NONE', #23922, .T. ) ;
#15069=CARTESIAN_POINT ( 'NONE',  ( -42.66890350025247614, 21.80565315997285225, 1.797223148894693034 ) ) ;
#15070=CARTESIAN_POINT ( 'NONE',  ( -28.92060043785469503, 77.33101988233063651, -1.524000000000008015 ) ) ;
#15074=CARTESIAN_POINT ( 'NONE',  ( -4.518622368304341386, 75.45558079800476037, -1.269999999999994911 ) ) ;
#15081=VERTEX_POINT ( 'NONE', #10770 ) ;
#15082=CARTESIAN_POINT ( 'NONE',  ( -56.37071950982826252, 3.976973756211601874, 2.203872415222109193 ) ) ;
#15088=AXIS2_PLACEMENT_3D ( 'NONE', #2789, #22125, #1946 ) ;
#15094=DIRECTION ( 'NONE',  ( -0.4849315768086480127, -0.8745520943968279060, -1.030032898892941415E-16 ) ) ;
#15096=DIRECTION ( 'NONE',  ( 5.188838149069472160E-16, -1.699382548006136559E-16, -1.000000000000000000 ) ) ;
#15123=ORIENTED_EDGE ( 'NONE', *, *, #41507, .T. ) ;
#15130=AXIS2_PLACEMENT_3D ( 'NONE', #39064, #9255, #12447 ) ;
#15131=VERTEX_POINT ( 'NONE', #1000 ) ;
#15132=CARTESIAN_POINT ( 'NONE',  ( -27.10368288468284348, 75.59070314479281194, -1.270000000000006679 ) ) ;
#15140=DIRECTION ( 'NONE',  ( -5.188838149069472160E-16, 1.699382548006136559E-16, 1.000000000000000000 ) ) ;
#15145=VERTEX_POINT ( 'NONE', #4822 ) ;
#15149=CARTESIAN_POINT ( 'NONE',  ( -57.79605042197209031, 0.9991760233552228199, 1.356629168144736441 ) ) ;
#15155=AXIS2_PLACEMENT_3D ( 'NONE', #10564, #20340, #23539 ) ;
#15159=CARTESIAN_POINT ( 'NONE',  ( -57.89731077922513691, 0.5615449381113218896, -1.034775302914740585E-14 ) ) ;
#15163=DIRECTION ( 'NONE',  ( -0.4849315768086535083, -0.8745520943968250194, -1.030032898892974695E-16 ) ) ;
#15166=DIRECTION ( 'NONE',  ( -0.8745520943968249084, 0.4849315768086534528, -5.361993529360573944E-16 ) ) ;
#15168=EDGE_CURVE ( 'NONE', #500, #9109, #33561, .T. ) ;
#15171=ORIENTED_EDGE ( 'NONE', *, *, #7183, .T. ) ;
#15172=CARTESIAN_POINT ( 'NONE',  ( -58.05614784158871799, 2.052449344323428626, -0.2046694337772892169 ) ) ;
#15173=ADVANCED_FACE ( 'NONE', ( #36563 ), #38989, .T. ) ;
#15174=EDGE_LOOP ( 'NONE', ( #30115, #14673, #23645, #11852 ) ) ;
#15184=CARTESIAN_POINT ( 'NONE',  ( -58.47923685707677777, 0.02532785185772538222, -0.7272094296869233698 ) ) ;
#15185=CIRCLE ( 'NONE', #29931, 0.7620000000000000107 ) ;
#15188=CARTESIAN_POINT ( 'NONE',  ( -5.719305292821792008, 76.92870498041706639, -1.269999999999995799 ) ) ;
#15190=CARTESIAN_POINT ( 'NONE',  ( -48.88984042444451461, 17.95628636586173599, -5.089849583058218663 ) ) ;
#15193=CARTESIAN_POINT ( 'NONE',  ( -55.73247374733729487, 5.492406230130003841, -2.854677165782116610 ) ) ;
#15200=CARTESIAN_POINT ( 'NONE',  ( -58.11258158571958177, 1.603013069906233934, -1.501710181103033781 ) ) ;
#15201=CARTESIAN_POINT ( 'NONE',  ( -10.15441061790785682, 81.86333342972157823, -1.269999999999998908 ) ) ;
#15213=CARTESIAN_POINT ( 'NONE',  ( -57.39043856515510811, 2.569568763584578974, 1.997829887931748427 ) ) ;
#15215=AXIS2_PLACEMENT_3D ( 'NONE', #12898, #38894, #9705 ) ;
#15216=CARTESIAN_POINT ( 'NONE',  ( -58.37241122568484286, -0.2962816677227336770, -1.039428729632916517E-14 ) ) ;
#15217=CARTESIAN_POINT ( 'NONE',  ( -51.24266872689721453, 19.11669921072455836, 1.581762766848667123 ) ) ;
#15220=CARTESIAN_POINT ( 'NONE',  ( -48.88162864671050301, 20.15829640254822408, -3.957548906738506123 ) ) ;
#15223=CIRCLE ( 'NONE', #20664, 0.2540000000000038338 ) ;
#15224=ORIENTED_EDGE ( 'NONE', *, *, #26070, .F. ) ;
#15227=AXIS2_PLACEMENT_3D ( 'NONE', #15923, #35127, #12535 ) ;
#15232=EDGE_CURVE ( 'NONE', #1811, #5717, #33579, .T. ) ;
#15237=CARTESIAN_POINT ( 'NONE',  ( -41.28107547821697665, 23.22158991241121129, -1.524000000000029775 ) ) ;
#15253=ORIENTED_EDGE ( 'NONE', *, *, #37950, .T. ) ;
#15255=DIRECTION ( 'NONE',  ( -0.8745520943968243532, 0.4849315768086547296, -6.829619984160642269E-16 ) ) ;
#15263=CARTESIAN_POINT ( 'NONE',  ( -58.16454994639720155, 0.1482675199355112661, 0.6170558006857020938 ) ) ;
#15264=DIRECTION ( 'NONE',  ( -0.8745520943968548844, 0.4849315768085996070, -4.268512490100397104E-16 ) ) ;
#15269=CARTESIAN_POINT ( 'NONE',  ( -54.12303657725384198, 9.464413707472848714, 3.807237671326749506 ) ) ;
#15275=CYLINDRICAL_SURFACE ( 'NONE', #7600, 0.2539999999999956737 ) ;
#15276=EDGE_CURVE ( 'NONE', #37721, #24344, #20763, .T. ) ;
#15279=CARTESIAN_POINT ( 'NONE',  ( -29.61277755921473442, 68.29894143241583038, 1.270000000001148877 ) ) ;
#15280=DIRECTION ( 'NONE',  ( 0.9575201071113178530, -0.2883665106726683858, 8.537024980200786319E-16 ) ) ;
#15281=DIRECTION ( 'NONE',  ( -5.188838149069472160E-16, 1.699382548006136559E-16, 1.000000000000000000 ) ) ;
#15282=CARTESIAN_POINT ( 'NONE',  ( -41.08172402297545744, 23.06268970575965938, 1.270028526666263646 ) ) ;
#15293=EDGE_LOOP ( 'NONE', ( #24765, #3616, #13927, #17951 ) ) ;
#15294=CARTESIAN_POINT ( 'NONE',  ( -57.24575050778504703, 1.871741192705528301, 0.5496743666258914196 ) ) ;
#15298=ORIENTED_EDGE ( 'NONE', *, *, #14908, .T. ) ;
#15300=ORIENTED_EDGE ( 'NONE', *, *, #25522, .F. ) ;
#15303=CIRCLE ( 'NONE', #1076, 0.2539999999999956737 ) ;
#15307=DIRECTION ( 'NONE',  ( 5.188838149069472160E-16, -1.699382548006136559E-16, -1.000000000000000000 ) ) ;
#15314=CARTESIAN_POINT ( 'NONE',  ( -45.39816439898302036, 21.06106408185672763, 4.080402960186377825 ) ) ;
#15315=CARTESIAN_POINT ( 'NONE',  ( -28.92060043785469503, 77.33101988233063651, 1.269999999999991136 ) ) ;
#15326=CARTESIAN_POINT ( 'NONE',  ( -58.70413935429054675, 0.2332485698458008905, 0.6626129746612758886 ) ) ;
#15331=EDGE_CURVE ( 'NONE', #41136, #1859, #32911, .T. ) ;
#15334=CIRCLE ( 'NONE', #9246, 8.794749999999993406 ) ;
#15345=ORIENTED_EDGE ( 'NONE', *, *, #32407, .T. ) ;
#15346=CARTESIAN_POINT ( 'NONE',  ( -41.05189575270519242, 23.09451173561983950, 0.4656666666666613996 ) ) ;
#15360=DIRECTION ( 'NONE',  ( -0.9816537812491126225, -0.1906721105964872265, -8.537024980200846470E-16 ) ) ;
#15362=CARTESIAN_POINT ( 'NONE',  ( -58.47668496617072975, -0.4796687618228244743, 0.2989310191336559952 ) ) ;
#15363=TOROIDAL_SURFACE ( 'NONE', #30357, 2.286000000000000032, 0.2540000000000000036 ) ;
#15366=CARTESIAN_POINT ( 'NONE',  ( -17.65389921742010060, 84.42347906515803402, 1.269999999999995799 ) ) ;
#15372=EDGE_CURVE ( 'NONE', #2842, #4427, #8836, .T. ) ;
#15374=CARTESIAN_POINT ( 'NONE',  ( -56.88731995051696089, 2.378615435641953546, -0.1283520312635632321 ) ) ;
#15377=DIRECTION ( 'NONE',  ( 0.01731298258487451447, -0.9998501190848635423, 1.788962107505245826E-16 ) ) ;
#15378=CARTESIAN_POINT ( 'NONE',  ( -19.86616884172038766, 72.62886460123898758, -1.270000000000002460 ) ) ;
#15381=CARTESIAN_POINT ( 'NONE',  ( -6.135835944515187101, 77.40800365160224317, 1.270000000000003793 ) ) ;
#15382=DIRECTION ( 'NONE',  ( -5.188838149069472160E-16, 1.699382548006136559E-16, 1.000000000000000000 ) ) ;
#15387=CARTESIAN_POINT ( 'NONE',  ( -5.809227842914839179, 77.60418761620948658, 1.270000000000003126 ) ) ;
#15388=VERTEX_POINT ( 'NONE', #31408 ) ;
#15389=DIRECTION ( 'NONE',  ( -5.188838149069472160E-16, 1.699382548006136559E-16, 1.000000000000000000 ) ) ;
#15395=AXIS2_PLACEMENT_3D ( 'NONE', #40871, #7869, #8067 ) ;
#15397=CARTESIAN_POINT ( 'NONE',  ( -54.11170070365439955, 9.036272999044422605, -3.680880771591853229 ) ) ;
#15398=EDGE_CURVE ( 'NONE', #32706, #11324, #14997, .T. ) ;
#15399=ORIENTED_EDGE ( 'NONE', *, *, #39258, .F. ) ;
#15400=CIRCLE ( 'NONE', #9303, 0.7620000000000000107 ) ;
#15403=CARTESIAN_POINT ( 'NONE',  ( -51.39111418837354961, 13.76717004397113087, -4.421739674169018031 ) ) ;
#15406=CARTESIAN_POINT ( 'NONE',  ( -49.13940628111213016, 17.59503125033257120, -5.062072503518689537 ) ) ;
#15408=EDGE_LOOP ( 'NONE', ( #28304, #34498, #33384, #20140 ) ) ;
#15413=CARTESIAN_POINT ( 'NONE',  ( -57.64973313486724038, 1.352533784701764885, -1.499908592384923134 ) ) ;
#15417=AXIS2_PLACEMENT_3D ( 'NONE', #8463, #1868, #34657 ) ;
#15418=ADVANCED_FACE ( 'NONE', ( #14578 ), #41197, .F. ) ;
#15423=CARTESIAN_POINT ( 'NONE',  ( -41.05189575270519242, 23.09451173561982174, -0.2116666666666723873 ) ) ;
#15424=ORIENTED_EDGE ( 'NONE', *, *, #991, .T. ) ;
#15426=CARTESIAN_POINT ( 'NONE',  ( -56.71132732703541990, 3.319205314284062958, 2.191228219141345246 ) ) ;
#15427=CARTESIAN_POINT ( 'NONE',  ( -53.06925326111847596, 10.99994025872287118, 4.072059781937412914 ) ) ;
#15430=CARTESIAN_POINT ( 'NONE',  ( -50.42190507837991476, 20.37545339363690999, 1.629190407695419784 ) ) ;
#15432=ORIENTED_EDGE ( 'NONE', *, *, #15331, .T. ) ;
#15433=CARTESIAN_POINT ( 'NONE',  ( -49.18824384045164777, 22.20099125052343680, -1.469723468883198825 ) ) ;
#15445=CARTESIAN_POINT ( 'NONE',  ( -17.32429653712378936, 61.56493206124108042, 1.269999999999999796 ) ) ;
#15448=DIRECTION ( 'NONE',  ( 5.188838149069472160E-16, -1.699382548006136559E-16, -1.000000000000000000 ) ) ;
#15451=ORIENTED_EDGE ( 'NONE', *, *, #37372, .T. ) ;
#15453=LINE ( 'NONE', #37409, #14322 ) ;
#15465=CARTESIAN_POINT ( 'NONE',  ( -15.27962295839633811, 80.49293118800726177, 1.523999999999998023 ) ) ;
#15466=CARTESIAN_POINT ( 'NONE',  ( -42.09814309847200064, 23.46876350539121248, -1.524000000000005794 ) ) ;
#15470=EDGE_CURVE ( 'NONE', #39412, #34293, #26762, .T. ) ;
#15472=VECTOR ( 'NONE', #34802, 1000.000000000000227 ) ;
#15474=EDGE_CURVE ( 'NONE', #4252, #2129, #21999, .T. ) ;
#15477=CARTESIAN_POINT ( 'NONE',  ( -45.76673701974917208, 25.51931200435043934, -1.524000000000008237 ) ) ;
#15480=CARTESIAN_POINT ( 'NONE',  ( -58.27229612817279047, -0.08447917103104905789, 0.4063237998337170254 ) ) ;
#15481=CARTESIAN_POINT ( 'NONE',  ( -9.960492004070044203, 64.81807050032566053, 1.270000000000003126 ) ) ;
#15482=UNCERTAINTY_MEASURE_WITH_UNIT (LENGTH_MEASURE( 1.000000000000000082E-05 ), #14434, 'distance_accuracy_value', 'NONE');
#15485=ORIENTED_EDGE ( 'NONE', *, *, #40949, .T. ) ;
#15486=CARTESIAN_POINT ( 'NONE',  ( -55.11216289415786207, 6.786895728730008237, 3.177266426849158609 ) ) ;
#15490=DIRECTION ( 'NONE',  ( 0.7548010569845451379, 0.6559537821943047797, 0.000000000000000000 ) ) ;
#15494=CARTESIAN_POINT ( 'NONE',  ( -28.94717034999018068, 63.96727089256646082, 1.523999999999993582 ) ) ;
#15495=DIRECTION ( 'NONE',  ( -0.8745520943968250194, 0.4849315768086535083, -5.424246918827963022E-16 ) ) ;
#15496=CARTESIAN_POINT ( 'NONE',  ( -42.60041433329244853, 22.17261999083466506, 1.881317670890278126 ) ) ;
#15499=CARTESIAN_POINT ( 'NONE',  ( -4.095482865093060809, 71.62450171983788039, -1.269999999999994023 ) ) ;
#15509=CARTESIAN_POINT ( 'NONE',  ( -57.25386126824266597, 1.903786294961781866, 0.7664973485411351595 ) ) ;
#15513=ORIENTED_EDGE ( 'NONE', *, *, #21522, .F. ) ;
#15525=FACE_OUTER_BOUND ( 'NONE', #21738, .T. ) ;
#15529=CARTESIAN_POINT ( 'NONE',  ( -46.07906060731711761, 24.80782705053048076, 1.769089518195985367 ) ) ;
#15533=ORIENTED_EDGE ( 'NONE', *, *, #36996, .T. ) ;
#15535=AXIS2_PLACEMENT_3D ( 'NONE', #25849, #18828, #12657 ) ;
#15543=CARTESIAN_POINT ( 'NONE',  ( -55.34794038087419210, 7.786537553440359360, 3.264576684945853291 ) ) ;
#15548=FACE_OUTER_BOUND ( 'NONE', #33909, .T. ) ;
#15566=CARTESIAN_POINT ( 'NONE',  ( -5.369399562154598904, 64.90898011766716991, -1.523999999999993582 ) ) ;
#15570=ORIENTED_EDGE ( 'NONE', *, *, #16742, .F. ) ;
#15572=DIRECTION ( 'NONE',  ( -0.3256999990547897461, -0.9454731675810318370, 0.000000000000000000 ) ) ;
#15573=AXIS2_PLACEMENT_3D ( 'NONE', #24713, #24929, #18524 ) ;
#15574=DIRECTION ( 'NONE',  ( -5.188838149069471174E-16, 1.699382548006136313E-16, 1.000000000000000000 ) ) ;
#15575=CARTESIAN_POINT ( 'NONE',  ( -58.67120857663415734, -0.3138064510425503384, 0.3172299661764326761 ) ) ;
#15586=DIRECTION ( 'NONE',  ( -0.9816537812491090698, -0.1906721105965065721, -4.769617732184476148E-16 ) ) ;
#15587=DIRECTION ( 'NONE',  ( 0.01731298258488512057, -0.9998501190848634312, 6.551018405069406341E-15 ) ) ;
#15594=ORIENTED_EDGE ( 'NONE', *, *, #14403, .T. ) ;
#15596=AXIS2_PLACEMENT_3D ( 'NONE', #18896, #31905, #1896 ) ;
#15604=CARTESIAN_POINT ( 'NONE',  ( -56.22360126104668154, 4.817347650610097176, -2.667469593848362130 ) ) ;
#15607=DIRECTION ( 'NONE',  ( 5.188838149069472160E-16, -1.699382548006136559E-16, -1.000000000000000000 ) ) ;
#15612=CARTESIAN_POINT ( 'NONE',  ( -50.36516092884956208, 15.79195539882771726, -4.916963016749614113 ) ) ;
#15618=EDGE_CURVE ( 'NONE', #24697, #30779, #34246, .T. ) ;
#15628=CARTESIAN_POINT ( 'NONE',  ( -46.43071087740785430, 19.11736041196146374, -2.831212230509051686 ) ) ;
#15629=ORIENTED_EDGE ( 'NONE', *, *, #40979, .T. ) ;
#15631=CARTESIAN_POINT ( 'NONE',  ( -58.43690671596436914, -0.4125963578781866037, -1.035377653829272970E-14 ) ) ;
#15632=CARTESIAN_POINT ( 'NONE',  ( -54.02024612309215001, 9.209302577745638985, 3.715716622219290777 ) ) ;
#15635=CARTESIAN_POINT ( 'NONE',  ( -53.18864123405685262, 14.74122628988702743, 1.932938280191007996 ) ) ;
#15638=CARTESIAN_POINT ( 'NONE',  ( -47.16890147375944764, 22.20336809214633433, -4.187060126831887885 ) ) ;
#15653=CARTESIAN_POINT ( 'NONE',  ( -17.64290547347870941, 83.78857423953914463, 1.269999999999996909 ) ) ;
#15663=DIRECTION ( 'NONE',  ( -0.7770581983690701966, 0.6294287539884197979, -8.537024980200731099E-16 ) ) ;
#15670=PLANE ( 'NONE',  #21290 ) ;
#15671=VERTEX_POINT ( 'NONE', #40030 ) ;
#15676=DIRECTION ( 'NONE',  ( -0.8745520943968245753, 0.4849315768086539524, -5.691349986800526185E-16 ) ) ;
#15680=EDGE_CURVE ( 'NONE', #25646, #6455, #257, .T. ) ;
#15683=CARTESIAN_POINT ( 'NONE',  ( -57.95663924081166130, 0.5986300452915040982, 0.9156402804120569172 ) ) ;
#15691=CIRCLE ( 'NONE', #6870, 0.3810000000000015041 ) ;
#15696=DIRECTION ( 'NONE',  ( -0.8745520943968250194, 0.4849315768086532863, -5.361993529360574930E-16 ) ) ;
#15698=CARTESIAN_POINT ( 'NONE',  ( -42.32312746590549324, 22.34068395104253213, 1.752427511502289370 ) ) ;
#15712=CARTESIAN_POINT ( 'NONE',  ( -56.89020484191215132, 2.444072280526621288, 0.3054065742134224881 ) ) ;
#15720=CYLINDRICAL_SURFACE ( 'NONE', #11346, 0.2540000000000012248 ) ;
#15726=CARTESIAN_POINT ( 'NONE',  ( -19.33375693323417011, 80.42273151551299293, -1.524000000000003574 ) ) ;
#15729=CARTESIAN_POINT ( 'NONE',  ( -46.60530155212508419, 26.17382724835469432, 1.171222222222213505 ) ) ;
#15731=CARTESIAN_POINT ( 'NONE',  ( -45.76673701974917208, 25.51931200435043934, 1.523999999999991806 ) ) ;
#15734=ADVANCED_FACE ( 'NONE', ( #24643 ), #38349, .T. ) ;
#15741=CIRCLE ( 'NONE', #12356, 0.5080000000000000071 ) ;
#15745=CARTESIAN_POINT ( 'NONE',  ( -15.37877921309977047, 79.99470228764801050, 1.269999999999996909 ) ) ;
#15746=DIRECTION ( 'NONE',  ( -0.8745520943968225769, 0.4849315768086578382, -5.691349986800571545E-16 ) ) ;
#15751=DIRECTION ( 'NONE',  ( 5.188838149069472160E-16, -1.699382548006136559E-16, -1.000000000000000000 ) ) ;
#15754=ORIENTED_EDGE ( 'NONE', *, *, #31878, .T. ) ;
#15758=VECTOR ( 'NONE', #6376, 999.9999999999998863 ) ;
#15763=ORIENTED_EDGE ( 'NONE', *, *, #24064, .F. ) ;
#15765=EDGE_LOOP ( 'NONE', ( #41984, #3784, #17398, #16364 ) ) ;
#15766=FACE_OUTER_BOUND ( 'NONE', #36102, .T. ) ;
#15773=CARTESIAN_POINT ( 'NONE',  ( -48.28978369826177186, 19.63653578263564015, -5.206999999995405304 ) ) ;
#15777=ORIENTED_EDGE ( 'NONE', *, *, #30869, .T. ) ;
#15778=CARTESIAN_POINT ( 'NONE',  ( -8.584014518950164430, 73.13423810798757074, -1.523999999999996691 ) ) ;
#15786=CIRCLE ( 'NONE', #2896, 0.5080000000000000071 ) ;
#15787=CARTESIAN_POINT ( 'NONE',  ( -8.210443557797230341, 69.68696903609418314, -1.523999999999995802 ) ) ;
#15793=CARTESIAN_POINT ( 'NONE',  ( -10.44685452804831804, 82.62549350906336088, -1.269999999999999130 ) ) ;
#15794=CARTESIAN_POINT ( 'NONE',  ( -17.99070523305416813, 61.93444992276926797, -1.523999999999999799 ) ) ;
#15796=CARTESIAN_POINT ( 'NONE',  ( -47.16890147375937659, 22.20336809214646578, -4.187060126831891438 ) ) ;
#15801=CIRCLE ( 'NONE', #7684, 0.3810000000000000053 ) ;
#15806=CARTESIAN_POINT ( 'NONE',  ( -42.18385791109623995, 22.43440044418303714, -1.696665287888123208 ) ) ;
#15812=CARTESIAN_POINT ( 'NONE',  ( -58.09669861156134374, 0.8533854034191163951, -1.257397024040518563 ) ) ;
#15813=ORIENTED_EDGE ( 'NONE', *, *, #6532, .F. ) ;
#15814=CARTESIAN_POINT ( 'NONE',  ( -57.55255837555640852, 1.471581310123148967, -1.351947345341661721 ) ) ;
#15818=CARTESIAN_POINT ( 'NONE',  ( -17.97610982144389524, 83.97333317030323485, 1.523999999999995802 ) ) ;
#15822=AXIS2_PLACEMENT_3D ( 'NONE', #7340, #20095, #29700 ) ;
#15823=ORIENTED_EDGE ( 'NONE', *, *, #29542, .T. ) ;
#15831=TOROIDAL_SURFACE ( 'NONE', #26336, 8.794749999999996959, 0.2540000000000000036 ) ;
#15834=DIRECTION ( 'NONE',  ( 0.6675346791886971332, -0.7445787077807445309, -3.514707485634470267E-14 ) ) ;
#15837=CARTESIAN_POINT ( 'NONE',  ( -10.39456080247344083, 81.94606122948148652, 1.270000000000000240 ) ) ;
#15838=CARTESIAN_POINT ( 'NONE',  ( -47.20049172920048619, 19.11349993950443249, -3.907078929042799853 ) ) ;
#15840=CARTESIAN_POINT ( 'NONE',  ( -17.14500000000466784, 71.11999999999886768, -1.524000000000000909 ) ) ;
#15841=DIRECTION ( 'NONE',  ( -0.8745520943968235761, 0.4849315768086558398, -4.268512490100410909E-16 ) ) ;
#15842=CARTESIAN_POINT ( 'NONE',  ( -49.61317302244366090, 16.90600142608853318, 5.005032797918173237 ) ) ;
#15843=CARTESIAN_POINT ( 'NONE',  ( -33.42971872652992005, 49.93539301574497102, -1.524000000000005572 ) ) ;
#15844=CIRCLE ( 'NONE', #27416, 0.2539999999999997260 ) ;
#15846=CARTESIAN_POINT ( 'NONE',  ( -54.34407705511657127, 12.44913727002957415, 1.242021477015509578 ) ) ;
#15848=ORIENTED_EDGE ( 'NONE', *, *, #29037, .T. ) ;
#15849=CARTESIAN_POINT ( 'NONE',  ( -52.41299847468118855, 17.00754718993399095, -1.481513115354252452 ) ) ;
#15858=TOROIDAL_SURFACE ( 'NONE', #40392, 0.7620000000000000107, 0.2540000000000000036 ) ;
#15864=FACE_OUTER_BOUND ( 'NONE', #21937, .T. ) ;
#15865=EDGE_CURVE ( 'NONE', #1003, #3266, #25429, .T. ) ;
#15869=CARTESIAN_POINT ( 'NONE',  ( -47.84356795211458291, 19.38525671449504983, 5.197506975155153697 ) ) ;
#15875=DIRECTION ( 'NONE',  ( -0.8745520943968250194, 0.4849315768086535083, -5.424246918827963022E-16 ) ) ;
#15879=CIRCLE ( 'NONE', #19978, 0.2540000000000052771 ) ;
#15881=CARTESIAN_POINT ( 'NONE',  ( -43.87210973174860129, 22.05421410453335795, -2.454571855453439255 ) ) ;
#15885=CARTESIAN_POINT ( 'NONE',  ( -17.14500000000466784, 71.11999999999886768, -1.270000000000000684 ) ) ;
#15891=CARTESIAN_POINT ( 'NONE',  ( -19.97113776634630611, 79.44829951959813741, 1.523999999999995802 ) ) ;
#15893=CARTESIAN_POINT ( 'NONE',  ( -58.37116772670351850, -0.2940390518722524327, -2.603646672650065119E-13 ) ) ;
#15906=CARTESIAN_POINT ( 'NONE',  ( -29.20589784623331653, 64.40785669711193862, 1.269999999999897211 ) ) ;
#15908=CARTESIAN_POINT ( 'NONE',  ( -23.75997692595333177, 82.67351089148900201, -1.270000000000006235 ) ) ;
#15918=AXIS2_PLACEMENT_3D ( 'NONE', #24690, #31091, #34714 ) ;
#15923=CARTESIAN_POINT ( 'NONE',  ( -17.14500000000466784, 71.11999999999886768, -1.524000000000000909 ) ) ;
#15930=AXIS2_PLACEMENT_3D ( 'NONE', #41960, #35147, #16148 ) ;
#15931=DIRECTION ( 'NONE',  ( -0.8745520943968235761, 0.4849315768086558398, -4.268512490100410909E-16 ) ) ;
#15937=CARTESIAN_POINT ( 'NONE',  ( -46.75595590928379863, 25.85823223380729985, 1.409582097145047674 ) ) ;
#15941=CARTESIAN_POINT ( 'NONE',  ( -47.11704014324646295, 20.18577099567727373, 5.127035723291425207 ) ) ;
#15942=CARTESIAN_POINT ( 'NONE',  ( -58.66106266037335359, -0.3146683754999778926, 0.3235272937950393612 ) ) ;
#15944=EDGE_LOOP ( 'NONE', ( #12826, #19172, #35602, #6721 ) ) ;
#15945=VERTEX_POINT ( 'NONE', #8986 ) ;
#15954=CARTESIAN_POINT ( 'NONE',  ( -18.01920641645601151, 83.84822824455466161, -1.524000000000003352 ) ) ;
#15963=DIRECTION ( 'NONE',  ( 0.9575201071113187412, -0.2883665106726659433, -1.122696976216275637E-15 ) ) ;
#15968=ORIENTED_EDGE ( 'NONE', *, *, #24603, .F. ) ;
#15969=ORIENTED_EDGE ( 'NONE', *, *, #5827, .F. ) ;
#15970=CARTESIAN_POINT ( 'NONE',  ( -41.31984638471809745, 22.80761424078405497, 1.396846000931794007 ) ) ;
#15977=FACE_OUTER_BOUND ( 'NONE', #37938, .T. ) ;
#15981=ADVANCED_FACE ( 'NONE', ( #34984 ), #15858, .T. ) ;
#15982=ORIENTED_EDGE ( 'NONE', *, *, #29205, .T. ) ;
#15983=CARTESIAN_POINT ( 'NONE',  ( -10.84307050033138786, 78.30450799593342026, 1.270000000000000240 ) ) ;
#15985=DIRECTION ( 'NONE',  ( -0.9454731675810336133, 0.3256999990547843615, -5.459396135145337199E-16 ) ) ;
#15987=CARTESIAN_POINT ( 'NONE',  ( -24.57769139521899149, 76.70147894597536720, -1.524000000000005572 ) ) ;
#15996=VECTOR ( 'NONE', #20810, 1000.000000000000227 ) ;
#16001=CARTESIAN_POINT ( 'NONE',  ( -10.75478607932181241, 82.07015292912137738, 1.270000000000000684 ) ) ;
#16005=DIRECTION ( 'NONE',  ( -0.8745520943968240202, 0.4849315768086551737, -5.361993529360572958E-16 ) ) ;
#16011=LINE ( 'NONE', #32636, #18863 ) ;
#16013=DIRECTION ( 'NONE',  ( 0.9816537812491126225, 0.1906721105964872265, 8.537024980200846470E-16 ) ) ;
#16018=CARTESIAN_POINT ( 'NONE',  ( -56.12001930601648070, 5.030854614368569955, -2.726109727168831931 ) ) ;
#16019=ORIENTED_EDGE ( 'NONE', *, *, #37299, .T. ) ;
#16020=CARTESIAN_POINT ( 'NONE',  ( -58.14608079600321133, 0.1881903270869317302, -0.6509722733302600872 ) ) ;
#16022=CARTESIAN_POINT ( 'NONE',  ( -17.09258512000246100, 84.17916046765628835, -1.270000000000002904 ) ) ;
#16023=B_SPLINE_SURFACE_WITH_KNOTS ( 'NONE', 3, 3, ( 
 ( #32348, #38539, #15729, #5761, #12548, #31937, #28934, #22110, #28734 ),
 ( #32143, #41327, #42160, #5966, #41747, #9354, #12753, #6169, #9153 ),
 ( #22316, #41952, #29143, #35342, #8939, #12130, #19546, #19342, #28531 ),
 ( #38957, #12955, #19139, #9555, #22527, #41536, #35556, #25949, #6372 ),
 ( #21905, #22732, #9768, #35763, #31723, #38335, #35139, #6790, #13177 ),
 ( #13387, #36406, #16789, #9973, #33209, #7640, #33414, #20184, #30206 ),
 ( #39166, #201, #4034, #16995, #26807, #39815, #36821, #29790, #23589 ),
 ( #7223, #629, #7011, #35973, #32996, #20389, #4458, #29994, #10819 ),
 ( #19756, #7431, #23802, #26588, #3825, #10401, #22946, #834, #36191 ),
 ( #39382, #13599, #13809, #39598, #29583, #14010, #23373, #40025, #32779 ),
 ( #20599, #26374, #19980, #10608, #4246, #3609, #36612, #17208, #1046 ),
 ( #27017, #33630, #16571, #29363, #26164, #417, #10185, #23154, #38021 ),
 ( #18406, #41225, #31413, #21805, #8842, #24588, #37801, #2255, #1828 ),
 ( #14792, #5239, #8421, #18194, #34619, #15430, #41439, #37595, #34205 ),
 ( #12459, #25236, #12027, #11819, #25019, #12244, #28002, #21379, #27795 ),
 ( #11604, #34832, #5666, #18623, #8627, #15217, #34405, #31628, #17990 ),
 ( #2677, #30987, #31195, #21590, #2468, #41011, #28432, #5446, #2038 ),
 ( #15003, #5032, #24808, #38240, #18834, #9057, #40803, #28219, #31838 ),
 ( #22022, #35050, #5871, #41651, #15635, #28640, #25453, #8205, #21177 ),
 ( #114, #6078, #9468, #38864, #25652, #15846, #29267, #36099, #19669 ),
 ( #32683, #38660, #22431, #19040, #16263, #35460, #10093, #9675, #6485 ),
 ( #39287, #3093, #22640, #19460, #9880, #3300, #6283, #28852, #16052 ),
 ( #13292, #12868, #32046, #9266, #16687, #16479, #19254, #32263, #6913 ),
 ( #35676, #29055, #42073, #25856, #32470, #23066, #13077, #26277, #29483 ),
 ( #22225, #41865, #534, #19883, #26068, #39078, #22850, #325, #35890 ),
 ( #2883, #29692, #12662, #6700, #3518, #32898, #3729, #13508, #38450 ),
 ( #35254, #39716, #20928, #7131, #23487, #26914, #36935, #4148, #40138 ),
 ( #741, #10720, #10516, #10307, #36512, #23919, #37139, #27337, #36311 ),
 ( #7960, #30734, #1367, #17111, #10930, #17732, #33319, #7755, #30112 ),
 ( #952, #11143, #23701, #13920, #40349, #23275, #33951, #4783, #24130 ),
 ( #20087, #17527, #36721, #39928, #33110, #7543, #20504, #14123, #7333 ),
 ( #33532, #20291, #4364, #1582, #13716, #26497, #17324, #39501, #30313 ),
 ( #1158, #27123, #14325, #20720, #3941, #16901, #29903, #4568, #26710 ),
 ( #33744, #30528, #14957, #21338, #18151, #14749, #37760, #28388, #24761 ) ),
 .UNSPECIFIED., .F., .F., .F.,
 ( 4, 1, 1, 1, 1, 1, 1, 1, 1, 1, 1, 2, 1, 1, 1, 1, 1, 1, 1, 1, 1, 1, 1, 1, 1, 1, 1, 1, 1, 1, 4 ),
 ( 4, 1, 1, 1, 1, 1, 4 ),
 ( 0.000000000000000000, 0.01653533301974152714, 0.03307066603948305428, 0.04960599905922458142, 0.06614133207896610855, 0.09921199811844916283, 0.1322826641579322171, 0.1653533301974152714, 0.1984239962368983257, 0.2314946622763813799, 0.2500000000000000000, 0.2645653283158644342, 0.3105299952961229071, 0.3335123287862520325, 0.3564946622763812689, 0.4024593292566397418, 0.4943886632171566875, 0.5863179971776735222, 0.6666666666666666297, 0.6782473311381906900, 0.7701766650987074136, 0.8161413320789658865, 0.8850883325493537068, 0.8965794992944182695, 0.9080706660394826102, 0.9195618327845473949, 0.9310529995296121797, 0.9425441662746769644, 0.9540353330197415271, 0.9770176665098706525, 1.000000000000000000 ),
 ( 0.000000000000000000, 0.2500000000000000000, 0.4444444444444445308, 0.5000000000000000000, 0.7500000000000000000, 0.8333333333333333703, 1.000000000000000000 ),
 .UNSPECIFIED. ) ;
#16025=CARTESIAN_POINT ( 'NONE',  ( -28.60507221318228943, 76.72702915747851193, 1.269999999999991358 ) ) ;
#16028=CARTESIAN_POINT ( 'NONE',  ( -58.07447437077728125, 1.735896131820596766, -1.499107834811110429 ) ) ;
#16029=ORIENTED_EDGE ( 'NONE', *, *, #1445, .F. ) ;
#16032=AXIS2_PLACEMENT_3D ( 'NONE', #26138, #22917, #23559 ) ;
#16033=ORIENTED_EDGE ( 'NONE', *, *, #20043, .T. ) ;
#16036=LINE ( 'NONE', #42056, #40843 ) ;
#16037=CARTESIAN_POINT ( 'NONE',  ( -14.60888863026623952, 79.54114996201613508, 1.523999999999998467 ) ) ;
#16044=CARTESIAN_POINT ( 'NONE',  ( -51.58367816905025194, 14.91232437457545146, -4.609044670965841917 ) ) ;
#16045=CARTESIAN_POINT ( 'NONE',  ( -44.40685758373556524, 19.43703734468909516, -6.894256627225939810E-15 ) ) ;
#16047=CARTESIAN_POINT ( 'NONE',  ( -46.74696603144393237, 25.88044175092360888, -1.397587819153285338 ) ) ;
#16048=CARTESIAN_POINT ( 'NONE',  ( -56.42620073798607194, 4.397991135091313453, 2.549475455950332758 ) ) ;
#16050=DIRECTION ( 'NONE',  ( -0.1565721916417968096, -0.9876665170007964401, 0.000000000000000000 ) ) ;
#16052=CARTESIAN_POINT ( 'NONE',  ( -55.80532936045926107, 9.325833942460080905, -1.040959450429527543E-14 ) ) ;
#16053=CIRCLE ( 'NONE', #3160, 0.2539999999999998925 ) ;
#16055=TOROIDAL_SURFACE ( 'NONE', #28986, 0.7620000000000000107, 0.2540000000000000036 ) ;
#16057=CARTESIAN_POINT ( 'NONE',  ( -55.15137202863810728, 10.98262019425784430, -0.5441000652716039276 ) ) ;
#16059=VERTEX_POINT ( 'NONE', #40224 ) ;
#16064=DIRECTION ( 'NONE',  ( 5.188838149069472160E-16, -1.699382548006136559E-16, -1.000000000000000000 ) ) ;
#16067=DIRECTION ( 'NONE',  ( -0.8745520943968245753, 0.4849315768086539524, -5.691349986800526185E-16 ) ) ;
#16070=CARTESIAN_POINT ( 'NONE',  ( -14.42383115828894624, 69.61113539875873357, -1.269999999999998908 ) ) ;
#16071=CARTESIAN_POINT ( 'NONE',  ( -10.15441061790785859, 81.86333342972157823, 1.270000000000000018 ) ) ;
#16074=CARTESIAN_POINT ( 'NONE',  ( -58.35078352787948575, -0.2517290638376923906, -0.1717528990698407032 ) ) ;
#16080=CARTESIAN_POINT ( 'NONE',  ( -30.19451713491628553, 70.61549828015994024, -1.524000000000007571 ) ) ;
#16086=CARTESIAN_POINT ( 'NONE',  ( -46.40591231939538375, 23.70796668624020853, -2.618124260499401945 ) ) ;
#16087=VECTOR ( 'NONE', #4138, 999.9999999999998863 ) ;
#16088=ORIENTED_EDGE ( 'NONE', *, *, #21410, .F. ) ;
#16091=DIRECTION ( 'NONE',  ( 2.458663194297837693E-13, 4.507549189546035939E-13, 1.000000000000000000 ) ) ;
#16098=AXIS2_PLACEMENT_3D ( 'NONE', #11532, #37521, #18755 ) ;
#16101=ORIENTED_EDGE ( 'NONE', *, *, #30576, .F. ) ;
#16103=LINE ( 'NONE', #22279, #31908 ) ;
#16104=VECTOR ( 'NONE', #7374, 1000.000000000000114 ) ;
#16109=EDGE_LOOP ( 'NONE', ( #11786, #13767, #24465, #14049 ) ) ;
#16113=DIRECTION ( 'NONE',  ( 5.188838149069472160E-16, -1.699382548006136559E-16, -1.000000000000000000 ) ) ;
#16114=AXIS2_PLACEMENT_3D ( 'NONE', #19613, #9413, #35405 ) ;
#16115=DIRECTION ( 'NONE',  ( -0.4849315768086426282, -0.8745520943968310146, -1.030032898892908135E-16 ) ) ;
#16127=DIRECTION ( 'NONE',  ( 2.731847993664264244E-14, 2.731847993664264244E-14, -1.000000000000000000 ) ) ;
#16129=ORIENTED_EDGE ( 'NONE', *, *, #25832, .F. ) ;
#16137=CIRCLE ( 'NONE', #39998, 0.7620000000000000107 ) ;
#16140=CARTESIAN_POINT ( 'NONE',  ( -46.75105655819150030, 25.87039714800365431, 1.402995854639100815 ) ) ;
#16143=CARTESIAN_POINT ( 'NONE',  ( -44.40534991575952972, 23.82367036525651116, 1.730788704199185624 ) ) ;
#16147=ORIENTED_EDGE ( 'NONE', *, *, #41455, .F. ) ;
#16148=DIRECTION ( 'NONE',  ( -0.8745520943968236871, 0.4849315768086558953, -5.361993529360571971E-16 ) ) ;
#16154=TOROIDAL_SURFACE ( 'NONE', #12765, 0.7620000000000000107, 0.2540000000000000036 ) ;
#16157=CARTESIAN_POINT ( 'NONE',  ( -41.23752580366543441, 23.26788267949596900, -1.270000000000005125 ) ) ;
#16165=EDGE_LOOP ( 'NONE', ( #15432, #25459, #30583, #40217 ) ) ;
#16174=VERTEX_POINT ( 'NONE', #2073 ) ;
#16176=CARTESIAN_POINT ( 'NONE',  ( -44.22601141000046709, 20.28211486706537414, 1.272444536529917958 ) ) ;
#16183=DIRECTION ( 'NONE',  ( -5.188838149069472160E-16, 1.699382548006136559E-16, 1.000000000000000000 ) ) ;
#16189=DIRECTION ( 'NONE',  ( 0.4849315768086480127, 0.8745520943968279060, 1.030032898892941415E-16 ) ) ;
#16197=DIRECTION ( 'NONE',  ( -0.9336303900108815501, -0.3582377630124009560, -4.235673982319039874E-16 ) ) ;
#16199=ADVANCED_FACE ( 'NONE', ( #22059 ), #15670, .F. ) ;
#16207=CARTESIAN_POINT ( 'NONE',  ( -41.28107547821700507, 23.22158991241123616, 1.269999999999992912 ) ) ;
#16215=ORIENTED_EDGE ( 'NONE', *, *, #14158, .T. ) ;
#16217=DIRECTION ( 'NONE',  ( -0.8745520943968244643, 0.4849315768086544520, -4.268512490100399076E-16 ) ) ;
#16219=CARTESIAN_POINT ( 'NONE',  ( -26.37263903973852663, 72.23735686029533554, -1.524000000000005794 ) ) ;
#16224=CARTESIAN_POINT ( 'NONE',  ( -58.56286374058253585, -0.1552305836484945689, -0.5530141226461045001 ) ) ;
#16231=EDGE_CURVE ( 'NONE', #23452, #27418, #37842, .T. ) ;
#16235=CARTESIAN_POINT ( 'NONE',  ( -57.07867440696631434, 2.606095844753547830, -1.988717289889820661 ) ) ;
#16236=ADVANCED_FACE ( 'NONE', ( #5481 ), #4189, .T. ) ;
#16237=EDGE_LOOP ( 'NONE', ( #10495, #30596, #28298, #7605 ) ) ;
#16244=CARTESIAN_POINT ( 'NONE',  ( -45.58494389689084869, 18.10922195552001313, -7.361215080689235889E-15 ) ) ;
#16245=EDGE_CURVE ( 'NONE', #33280, #20566, #22291, .T. ) ;
#16253=CARTESIAN_POINT ( 'NONE',  ( -47.93564525088164885, 15.36257551998183857, -8.154853246613427015E-15 ) ) ;
#16254=VERTEX_POINT ( 'NONE', #24368 ) ;
#16255=AXIS2_PLACEMENT_3D ( 'NONE', #38973, #9990, #19774 ) ;
#16258=CARTESIAN_POINT ( 'NONE',  ( -46.95911617132934879, 24.98948415085533270, 1.986615011824473864 ) ) ;
#16261=CARTESIAN_POINT ( 'NONE',  ( -58.82991074935231524, -0.2577531494038359794, -1.058401375502683064E-14 ) ) ;
#16263=CARTESIAN_POINT ( 'NONE',  ( -54.91040913962392978, 10.45702928859090086, 1.592171597931398619 ) ) ;
#16265=CARTESIAN_POINT ( 'NONE',  ( -57.39043856515510811, 2.569568763584578974, 1.997829887931748427 ) ) ;
#16269=CARTESIAN_POINT ( 'NONE',  ( -52.43464216530867361, 18.97776253654341616, -0.3470174342361405095 ) ) ;
#16276=DIRECTION ( 'NONE',  ( 5.188838149069472160E-16, -1.699382548006136559E-16, -1.000000000000000000 ) ) ;
#16279=CARTESIAN_POINT ( 'NONE',  ( -10.57002714855771686, 82.40335727708655611, -1.523999999999999355 ) ) ;
#16284=FACE_OUTER_BOUND ( 'NONE', #33808, .T. ) ;
#16295=EDGE_CURVE ( 'NONE', #23403, #21375, #25905, .T. ) ;
#16297=AXIS2_PLACEMENT_3D ( 'NONE', #28151, #23951, #15360 ) ;
#16298=ADVANCED_FACE ( 'NONE', ( #35238 ), #41637, .T. ) ;
#16303=CIRCLE ( 'NONE', #40128, 8.794749999999996959 ) ;
#16306=CARTESIAN_POINT ( 'NONE',  ( -48.08949201794742123, 19.91830422262442468, -5.194343260851647770 ) ) ;
#16307=EDGE_LOOP ( 'NONE', ( #22116, #13081, #6613, #25675 ) ) ;
#16315=CARTESIAN_POINT ( 'NONE',  ( -47.72134626992409778, 19.52826264939519163, -5.191136457097766943 ) ) ;
#16319=VERTEX_POINT ( 'NONE', #12852 ) ;
#16326=VERTEX_POINT ( 'NONE', #25436 ) ;
#16335=CARTESIAN_POINT ( 'NONE',  ( -14.64596739026573857, 69.73430801926814127, 1.269999999999999796 ) ) ;
#16341=ORIENTED_EDGE ( 'NONE', *, *, #32859, .T. ) ;
#16345=CARTESIAN_POINT ( 'NONE',  ( -26.29578028364076658, 73.87584665086983193, 1.269999999999993134 ) ) ;
#16355=CARTESIAN_POINT ( 'NONE',  ( -50.35389404691220960, 15.58445134054611003, 4.726195680281481515 ) ) ;
#16357=CIRCLE ( 'NONE', #30667, 0.3810000000000029474 ) ;
#16359=CARTESIAN_POINT ( 'NONE',  ( -51.54051843738712080, 14.84038450301108192, 4.692172599169413871 ) ) ;
#16360=LINE ( 'NONE', #39169, #15758 ) ;
#16364=ORIENTED_EDGE ( 'NONE', *, *, #21925, .T. ) ;
#16370=CARTESIAN_POINT ( 'NONE',  ( -46.95766867967832070, 25.94401225812155332, -9.481001462019121602E-15 ) ) ;
#16374=FACE_OUTER_BOUND ( 'NONE', #720, .T. ) ;
#16384=CARTESIAN_POINT ( 'NONE',  ( -8.428339483816529309, 74.57444062528223583, 1.270000000000002238 ) ) ;
#16391=EDGE_LOOP ( 'NONE', ( #26243, #37086, #11561, #34788, #3178 ) ) ;
#16392=CARTESIAN_POINT ( 'NONE',  ( -42.80040666669066241, 21.79149265709745009, 2.067570201390446449 ) ) ;
#16399=AXIS2_PLACEMENT_3D ( 'NONE', #11953, #37944, #40935 ) ;
#16405=CARTESIAN_POINT ( 'NONE',  ( -7.917360960270791281, 70.00264313970245666, 1.524000000000003574 ) ) ;
#16407=LINE ( 'NONE', #32827, #782 ) ;
#16411=VECTOR ( 'NONE', #23654, 1000.000000000000114 ) ;
#16426=CARTESIAN_POINT ( 'NONE',  ( -47.71508057896579658, 20.49549959222711593, -5.111566084959475731 ) ) ;
#16440=CARTESIAN_POINT ( 'NONE',  ( -58.67004091686991529, -0.3138842535942401590, -0.3180043108007239994 ) ) ;
#16441=VERTEX_POINT ( 'NONE', #16037 ) ;
#16442=CARTESIAN_POINT ( 'NONE',  ( -23.21760062652228385, 78.26400813401573942, 1.523999999999993360 ) ) ;
#16449=CARTESIAN_POINT ( 'NONE',  ( -58.83227707057486811, -0.08366279997995551554, -0.2458995907045101459 ) ) ;
#16458=CIRCLE ( 'NONE', #28044, 0.6349999999999998979 ) ;
#16459=CARTESIAN_POINT ( 'NONE',  ( -42.12253153191133492, 21.94389511927448311, -6.431429377749453771E-15 ) ) ;
#16467=AXIS2_PLACEMENT_3D ( 'NONE', #38010, #40793, #11593 ) ;
#16469=CARTESIAN_POINT ( 'NONE',  ( -47.40532530373579334, 16.48158934372809270, -0.7854836779716005690 ) ) ;
#16472=DIRECTION ( 'NONE',  ( -5.188838149069471174E-16, 1.699382548006136313E-16, 1.000000000000000000 ) ) ;
#16473=CARTESIAN_POINT ( 'NONE',  ( -23.09297118196009535, 77.93920196072180318, -1.524000000000005128 ) ) ;
#16479=CARTESIAN_POINT ( 'NONE',  ( -56.17386367503594613, 7.314326147911789811, 0.9214986423944734328 ) ) ;
#16480=CARTESIAN_POINT ( 'NONE',  ( -57.69570286664291103, 2.558035660193719529, 1.875687456014364152 ) ) ;
#16483=CARTESIAN_POINT ( 'NONE',  ( -54.68578128246380743, 13.03233524003756472, -0.2705950194913063767 ) ) ;
#16486=DIRECTION ( 'NONE',  ( 5.188838149069472160E-16, -1.699382548006136559E-16, -1.000000000000000000 ) ) ;
#16490=CARTESIAN_POINT ( 'NONE',  ( -6.401666570281891566, 64.12941061790216679, -1.269999999999994023 ) ) ;
#16498=CARTESIAN_POINT ( 'NONE',  ( -23.69188486464780752, 78.08202335040543574, -1.270000000000005347 ) ) ;
#16501=ORIENTED_EDGE ( 'NONE', *, *, #32307, .T. ) ;
#16517=CARTESIAN_POINT ( 'NONE',  ( -43.10982161678889213, 22.52422253607401359, -1.888110242252992066 ) ) ;
#16521=ADVANCED_FACE ( 'NONE', ( #723 ), #19319, .T. ) ;
#16523=AXIS2_PLACEMENT_3D ( 'NONE', #6814, #13622, #25976 ) ;
#16538=ADVANCED_FACE ( 'NONE', ( #3233 ), #3443, .F. ) ;
#16542=EDGE_LOOP ( 'NONE', ( #30605, #27265, #40094, #38708 ) ) ;
#16550=CARTESIAN_POINT ( 'NONE',  ( -49.26674734213554530, 17.44270459986159594, -5.073646373245743746 ) ) ;
#16561=AXIS2_PLACEMENT_3D ( 'NONE', #30557, #33772, #4806 ) ;
#16570=CARTESIAN_POINT ( 'NONE',  ( -46.70910030332949248, 25.96830944048481982, 1.353001860315405924 ) ) ;
#16571=CARTESIAN_POINT ( 'NONE',  ( -48.69154271504742582, 20.42972839736894386, 3.938715850604322721 ) ) ;
#16574=CARTESIAN_POINT ( 'NONE',  ( -51.34009458250667279, 14.66650723912346699, 4.800162786360129274 ) ) ;
#16579=ORIENTED_EDGE ( 'NONE', *, *, #22521, .F. ) ;
#16586=CARTESIAN_POINT ( 'NONE',  ( -46.81070079724250377, 25.76746909427398435, -1.215830024444428892 ) ) ;
#16588=AXIS2_PLACEMENT_3D ( 'NONE', #20745, #13746, #769 ) ;
#16600=CIRCLE ( 'NONE', #1666, 0.7620000000000015650 ) ;
#16607=CARTESIAN_POINT ( 'NONE',  ( -46.25688858429104044, 20.73875112231585760, 4.700046123029338219 ) ) ;
#16615=DIRECTION ( 'NONE',  ( -0.8745520943968235761, 0.4849315768086558398, -5.691349986800547879E-16 ) ) ;
#16619=ORIENTED_EDGE ( 'NONE', *, *, #33957, .T. ) ;
#16620=DIRECTION ( 'NONE',  ( 0.8745520943968236871, -0.4849315768086559508, 6.829619984160659032E-16 ) ) ;
#16623=DIRECTION ( 'NONE',  ( -0.4849315768086535083, -0.8745520943968250194, -1.030032898892974695E-16 ) ) ;
#16638=FACE_OUTER_BOUND ( 'NONE', #12349, .T. ) ;
#16652=CARTESIAN_POINT ( 'NONE',  ( -58.82993483412206359, -0.2576888758964282489, -0.02106341969870843475 ) ) ;
#16653=ORIENTED_EDGE ( 'NONE', *, *, #26678, .T. ) ;
#16658=CARTESIAN_POINT ( 'NONE',  ( -46.98357734554679155, 20.33138817508191210, 5.073745976080627607 ) ) ;
#16661=CARTESIAN_POINT ( 'NONE',  ( -58.37934292759150168, 0.9822739792931106662, -1.208960021102219340 ) ) ;
#16662=ORIENTED_EDGE ( 'NONE', *, *, #7382, .F. ) ;
#16665=ORIENTED_EDGE ( 'NONE', *, *, #19339, .T. ) ;
#16670=CARTESIAN_POINT ( 'NONE',  ( -54.09072575248404036, 8.649776409421397361, 3.422340198163080327 ) ) ;
#16678=CARTESIAN_POINT ( 'NONE',  ( -46.38316532014830784, 26.05065462784526176, -1.524000000000014676 ) ) ;
#16679=CARTESIAN_POINT ( 'NONE',  ( -55.00324375927522169, 6.200002331679180578, -1.420877854375708127 ) ) ;
#16684=CARTESIAN_POINT ( 'NONE',  ( -32.35167636075468778, 51.35580826818691236, -1.524000000000005128 ) ) ;
#16686=CARTESIAN_POINT ( 'NONE',  ( -17.09698261757901960, 84.43312239790384410, -1.270000000000002904 ) ) ;
#16687=CARTESIAN_POINT ( 'NONE',  ( -56.13924587166188473, 7.155854391526911051, 1.290439134121102782 ) ) ;
#16688=CARTESIAN_POINT ( 'NONE',  ( -58.10099831372669854, 0.3475205698689753930, 0.9728495803591148405 ) ) ;
#16691=EDGE_LOOP ( 'NONE', ( #24933, #9504, #5783, #27825 ) ) ;
#16692=CARTESIAN_POINT ( 'NONE',  ( -54.56940519185135230, 9.666406039105165604, -3.302709833357616365 ) ) ;
#16695=CYLINDRICAL_SURFACE ( 'NONE', #7670, 9.048749999999998295 ) ;
#16707=ORIENTED_EDGE ( 'NONE', *, *, #31345, .F. ) ;
#16708=CIRCLE ( 'NONE', #10596, 0.5080000000000014504 ) ;
#16712=CARTESIAN_POINT ( 'NONE',  ( -57.83236317642370494, 0.8674604446124462021, -1.063638734186429291 ) ) ;
#16727=EDGE_CURVE ( 'NONE', #11005, #40169, #30045, .T. ) ;
#16728=CARTESIAN_POINT ( 'NONE',  ( -42.33919149967392315, 22.05006338260229271, -1.842566675324098568 ) ) ;
#16732=DIRECTION ( 'NONE',  ( -5.188838149069472160E-16, 1.699382548006136559E-16, 1.000000000000000000 ) ) ;
#16737=AXIS2_PLACEMENT_3D ( 'NONE', #15132, #2388, #34969 ) ;
#16739=FACE_OUTER_BOUND ( 'NONE', #21098, .T. ) ;
#16741=CARTESIAN_POINT ( 'NONE',  ( -58.36969448265841720, -0.2913820931539540249, 0.003449905599825503141 ) ) ;
#16742=EDGE_CURVE ( 'NONE', #37219, #42027, #31404, .T. ) ;
#16746=DIRECTION ( 'NONE',  ( -5.188838149069472160E-16, 1.699382548006136559E-16, 1.000000000000000000 ) ) ;
#16755=DIRECTION ( 'NONE',  ( 5.188838149069472160E-16, -1.699382548006136559E-16, -1.000000000000000000 ) ) ;
#16756=DIRECTION ( 'NONE',  ( -0.8745520943968241312, 0.4849315768086548961, -5.424246918827962036E-16 ) ) ;
#16758=ADVANCED_FACE ( 'NONE', ( #467 ), #18463, .T. ) ;
#16762=CARTESIAN_POINT ( 'NONE',  ( -4.466782427718574588, 71.06098887363195615, 1.524000000000005128 ) ) ;
#16766=VERTEX_POINT ( 'NONE', #36659 ) ;
#16768=ORIENTED_EDGE ( 'NONE', *, *, #7082, .F. ) ;
#16771=EDGE_CURVE ( 'NONE', #37389, #32811, #11601, .T. ) ;
#16773=LINE ( 'NONE', #23141, #13158 ) ;
#16774=EDGE_CURVE ( 'NONE', #31966, #6546, #36107, .T. ) ;
#16779=DIRECTION ( 'NONE',  ( 5.188838149069472160E-16, -1.699382548006136559E-16, -1.000000000000000000 ) ) ;
#16787=VECTOR ( 'NONE', #8879, 1000.000000000000000 ) ;
#16788=CARTESIAN_POINT ( 'NONE',  ( -46.68753544603657701, 26.01473869131327277, 1.331541039591896070 ) ) ;
#16789=CARTESIAN_POINT ( 'NONE',  ( -47.17284909187768704, 24.49633334977720978, 1.858123130129375244 ) ) ;
#16790=DIRECTION ( 'NONE',  ( -0.8745520943968250194, 0.4849315768086532863, -5.361993529360574930E-16 ) ) ;
#16791=CARTESIAN_POINT ( 'NONE',  ( -48.98489377192316852, 18.65252824715059177, 5.272350768541908650 ) ) ;
#16792=CARTESIAN_POINT ( 'NONE',  ( -58.67922015684681014, -0.3140008337426106744, 0.3102499017298660511 ) ) ;
#16797=CARTESIAN_POINT ( 'NONE',  ( -43.93316818929329770, 24.49458088220322338, 1.523999999999992916 ) ) ;
#16802=CARTESIAN_POINT ( 'NONE',  ( -10.57002714855771863, 82.40335727708655611, 1.269999999999999796 ) ) ;
#16805=EDGE_CURVE ( 'NONE', #10192, #20421, #17022, .T. ) ;
#16813=FACE_OUTER_BOUND ( 'NONE', #30861, .T. ) ;
#16820=ORIENTED_EDGE ( 'NONE', *, *, #34009, .F. ) ;
#16821=CARTESIAN_POINT ( 'NONE',  ( -47.30388380253317138, 17.78501317193704168, 2.251402236601635742 ) ) ;
#16828=ADVANCED_FACE ( 'NONE', ( #40071 ), #2077, .T. ) ;
#16832=CIRCLE ( 'NONE', #13435, 9.048749999999998295 ) ;
#16833=ORIENTED_EDGE ( 'NONE', *, *, #8614, .T. ) ;
#16836=DIRECTION ( 'NONE',  ( -0.8745520943968243532, 0.4849315768086547296, -5.361993529360573944E-16 ) ) ;
#16851=CARTESIAN_POINT ( 'NONE',  ( -23.94760723868026631, 77.08694321397520355, -1.270000000000005347 ) ) ;
#16852=CYLINDRICAL_SURFACE ( 'NONE', #2332, 0.2540000000000051106 ) ;
#16855=FACE_OUTER_BOUND ( 'NONE', #30456, .T. ) ;
#16860=ORIENTED_EDGE ( 'NONE', *, *, #12063, .F. ) ;
#16861=DIRECTION ( 'NONE',  ( 0.3256999990547836399, 0.9454731675810339464, 0.000000000000000000 ) ) ;
#16868=CARTESIAN_POINT ( 'NONE',  ( -58.70775671454279632, -0.3148938609545903211, -0.2814231133491895132 ) ) ;
#16870=DIRECTION ( 'NONE',  ( -0.8745520943968235761, 0.4849315768086558398, -4.268512490100410909E-16 ) ) ;
#16884=CARTESIAN_POINT ( 'NONE',  ( -58.33447198145985624, -0.2173903971932067414, 0.2351149084158423719 ) ) ;
#16891=CARTESIAN_POINT ( 'NONE',  ( -54.95604735203036029, 6.474113128985478305, -1.942216106931691444 ) ) ;
#16894=CARTESIAN_POINT ( 'NONE',  ( -46.89996537977940960, 25.36638690764230475, -1.726091171922216727 ) ) ;
#16895=CARTESIAN_POINT ( 'NONE',  ( -48.12344719333864163, 19.06868139646365634, 5.226126700700302941 ) ) ;
#16896=CARTESIAN_POINT ( 'NONE',  ( -29.05311006333617740, 61.33684941847489114, -1.524000000000005128 ) ) ;
#16898=CYLINDRICAL_SURFACE ( 'NONE', #17791, 0.5080000000000000071 ) ;
#16899=LINE ( 'NONE', #32681, #3529 ) ;
#16901=CARTESIAN_POINT ( 'NONE',  ( -58.76922381231047865, 0.08391971067571446508, 0.07695160083611271573 ) ) ;
#16902=CARTESIAN_POINT ( 'NONE',  ( -58.07447437077728125, 1.735896131820596766, 1.499107834811089113 ) ) ;
#16904=ORIENTED_EDGE ( 'NONE', *, *, #1190, .F. ) ;
#16905=CARTESIAN_POINT ( 'NONE',  ( -57.34105142390578891, 4.241571993195719870, -1.052207516753799910E-14 ) ) ;
#16907=TOROIDAL_SURFACE ( 'NONE', #6764, 0.7620000000000000107, 0.2540000000000000036 ) ;
#16908=VERTEX_POINT ( 'NONE', #20025 ) ;
#16912=AXIS2_PLACEMENT_3D ( 'NONE', #29284, #39092, #9894 ) ;
#16917=CARTESIAN_POINT ( 'NONE',  ( -29.35745042155304674, 66.56063108281016127, 1.269999999999993801 ) ) ;
#16920=CARTESIAN_POINT ( 'NONE',  ( -48.40208230357499275, 18.68930050447353253, -5.198873216397010388 ) ) ;
#16921=FACE_OUTER_BOUND ( 'NONE', #29232, .T. ) ;
#16925=CARTESIAN_POINT ( 'NONE',  ( -58.06141239495070749, 0.3713401805837863723, -0.7746908926762229308 ) ) ;
#16932=ADVANCED_FACE ( 'NONE', ( #10867 ), #19744, .T. ) ;
#16935=ORIENTED_EDGE ( 'NONE', *, *, #40233, .T. ) ;
#16940=CARTESIAN_POINT ( 'NONE',  ( -51.81113891419111894, 13.24950054771400332, -4.495723625053127392 ) ) ;
#16949=CARTESIAN_POINT ( 'NONE',  ( -43.35906100199900948, 21.49635880980144265, -2.252931129856535097 ) ) ;
#16951=DIRECTION ( 'NONE',  ( 5.188838149069472160E-16, -1.699382548006136559E-16, -1.000000000000000000 ) ) ;
#16961=ORIENTED_EDGE ( 'NONE', *, *, #31930, .F. ) ;
#16965=CYLINDRICAL_SURFACE ( 'NONE', #32637, 0.6350000000000006750 ) ;
#16970=CARTESIAN_POINT ( 'NONE',  ( -58.13403979463072346, 0.7724927387370850163, -1.216435378340507745 ) ) ;
#16971=LINE ( 'NONE', #13786, #24319 ) ;
#16976=VERTEX_POINT ( 'NONE', #39645 ) ;
#16979=CARTESIAN_POINT ( 'NONE',  ( -41.09670346151922615, 23.04688172092959775, 1.270085369932517194 ) ) ;
#16984=PLANE ( 'NONE',  #1150 ) ;
#16990=AXIS2_PLACEMENT_3D ( 'NONE', #19921, #20124, #17358 ) ;
#16994=CARTESIAN_POINT ( 'NONE',  ( -57.92433820120297838, 0.6686165507389044693, 0.9561099433084984112 ) ) ;
#16995=CARTESIAN_POINT ( 'NONE',  ( -47.42394374581075311, 23.94708628835674702, 1.773793246466830453 ) ) ;
#16997=CARTESIAN_POINT ( 'NONE',  ( -56.34046819891496938, 4.202508019718290022, 2.501728563949842776 ) ) ;
#16998=CARTESIAN_POINT ( 'NONE',  ( -58.64399535964418675, -0.3105835279867479315, 0.3406522351893582767 ) ) ;
#16999=EDGE_CURVE ( 'NONE', #22644, #22759, #14472, .T. ) ;
#17001=DIRECTION ( 'NONE',  ( -0.8745520943968249084, 0.4849315768086533418, -5.271987356194193006E-16 ) ) ;
#17003=CARTESIAN_POINT ( 'NONE',  ( -47.07934102874904170, 22.98505637820369429, 3.579966862081928713 ) ) ;
#17004=EDGE_CURVE ( 'NONE', #19659, #11397, #25865, .T. ) ;
#17015=DIRECTION ( 'NONE',  ( -0.8745520943968249084, 0.4849315768086533418, -5.311926654347176508E-16 ) ) ;
#17016=CARTESIAN_POINT ( 'NONE',  ( -11.32337086946255056, 78.46996359545325106, -1.269999999999998908 ) ) ;
#17020=CYLINDRICAL_SURFACE ( 'NONE', #21108, 0.2539999999999937863 ) ;
#17022=CIRCLE ( 'NONE', #25211, 0.3810000000000007825 ) ;
#17027=ORIENTED_EDGE ( 'NONE', *, *, #4507, .F. ) ;
#17028=CARTESIAN_POINT ( 'NONE',  ( -44.02811856515548783, 21.20684991433588351, 2.650346054289406172 ) ) ;
#17030=SHAPE_DEFINITION_REPRESENTATION ( #7581, #22056 ) ;
#17037=FACE_OUTER_BOUND ( 'NONE', #2956, .T. ) ;
#17041=CARTESIAN_POINT ( 'NONE',  ( -23.69188486464780752, 78.08202335040543574, -1.524000000000005350 ) ) ;
#17042=CARTESIAN_POINT ( 'NONE',  ( -15.71196903609989626, 80.05455644220629097, -1.524000000000001798 ) ) ;
#17043=AXIS2_PLACEMENT_3D ( 'NONE', #42043, #5847, #32019 ) ;
#17047=DIRECTION ( 'NONE',  ( 5.188838149069472160E-16, -1.699382548006136559E-16, -1.000000000000000000 ) ) ;
#17050=DIRECTION ( 'NONE',  ( 5.188838149069472160E-16, -1.699382548006136559E-16, -1.000000000000000000 ) ) ;
#17060=EDGE_CURVE ( 'NONE', #16254, #39389, #12944, .T. ) ;
#17061=DIRECTION ( 'NONE',  ( 0.000000000000000000, 0.000000000000000000, -1.000000000000000000 ) ) ;
#17066=EDGE_CURVE ( 'NONE', #3855, #21812, #27902, .T. ) ;
#17068=CARTESIAN_POINT ( 'NONE',  ( -25.97603047661466036, 74.27059221564131519, -1.270000000000006013 ) ) ;
#17069=ORIENTED_EDGE ( 'NONE', *, *, #39197, .F. ) ;
#17073=AXIS2_PLACEMENT_3D ( 'NONE', #6509, #9903, #32708 ) ;
#17075=CARTESIAN_POINT ( 'NONE',  ( -58.63704644534278998, -0.3018330928726550844, -0.3571578142998330097 ) ) ;
#17076=ORIENTED_EDGE ( 'NONE', *, *, #24320, .T. ) ;
#17077=CARTESIAN_POINT ( 'NONE',  ( -58.35171525856278407, -0.2536858515839318651, -0.1680674994487795226 ) ) ;
#17079=( NAMED_UNIT ( * ) SI_UNIT ( $, .STERADIAN. ) SOLID_ANGLE_UNIT ( ) );
#17083=TOROIDAL_SURFACE ( 'NONE', #20443, 0.3810000000000000608, 0.2540000000000000036 ) ;
#17085=CARTESIAN_POINT ( 'NONE',  ( -10.73808814597608574, 77.14487411131506178, 1.270000000000000684 ) ) ;
#17091=CARTESIAN_POINT ( 'NONE',  ( -58.35474420885229563, -0.2600319066115991395, 0.1537082109190309465 ) ) ;
#17099=EDGE_CURVE ( 'NONE', #22469, #30132, #39509, .T. ) ;
#17100=CARTESIAN_POINT ( 'NONE',  ( -51.79385399617232366, 10.81633633057992050, -0.6965991018155879289 ) ) ;
#17105=CARTESIAN_POINT ( 'NONE',  ( -10.75478607932181241, 82.07015292912137738, -1.269999999999999130 ) ) ;
#17106=CARTESIAN_POINT ( 'NONE',  ( -31.81160527991017872, 53.04071001975501076, -1.523999999997152521 ) ) ;
#17110=DIRECTION ( 'NONE',  ( -5.188838149069472160E-16, 1.699382548006136559E-16, 1.000000000000000000 ) ) ;
#17111=CARTESIAN_POINT ( 'NONE',  ( -58.13344828981739454, 1.721081384412917359, 0.8123818723938425190 ) ) ;
#17115=CARTESIAN_POINT ( 'NONE',  ( -56.26154134542980501, 7.775270144418685803, -1.077953313861507864E-14 ) ) ;
#17117=ORIENTED_EDGE ( 'NONE', *, *, #33964, .T. ) ;
#17118=DIRECTION ( 'NONE',  ( -0.8745520943968235761, 0.4849315768086558953, -5.361993529360570985E-16 ) ) ;
#17126=CARTESIAN_POINT ( 'NONE',  ( -30.04222987988044835, 57.94556081694326366, 1.269999999999993801 ) ) ;
#17133=CARTESIAN_POINT ( 'NONE',  ( -57.73431293437639056, 1.079294370200192699, -1.168893109563275301 ) ) ;
#17138=B_SPLINE_CURVE_WITH_KNOTS ( 'NONE', 3,
 ( #4121, #919, #36690, #10692, #7724, #16658, #10064, #14096, #20690, #33715, #4536, #17498, #1337, #26248, #39257, #23035, #37733, #8341, #1757, #33919, #34550, #11113, #27520, #24730 ),
 .UNSPECIFIED., .F., .F.,
 ( 4, 2, 2, 2, 2, 2, 2, 2, 2, 2, 2, 4 ),
 ( 0.000000000000000000, 0.0005547041830063565359, 0.001109408366012713072, 0.001664112549019069716, 0.002218816732025426144, 0.003328225098038139432, 0.004437633464050852287, 0.005547041830063565576, 0.006656450196076278865, 0.007211154379082635076, 0.007765858562088991286, 0.008875266928101688962 ),
 .UNSPECIFIED. ) ;
#17139=CARTESIAN_POINT ( 'NONE',  ( -42.79661761208809168, 21.81806929429799879, -2.089873509012822428 ) ) ;
#17140=CIRCLE ( 'NONE', #37534, 0.2540000000000000036 ) ;
#17147=CARTESIAN_POINT ( 'NONE',  ( -58.85052583756497313, -0.2027389052197895725, -7.881329963315141238E-15 ) ) ;
#17149=CARTESIAN_POINT ( 'NONE',  ( -49.13940628111213016, 17.59503125033257120, -5.062072503518689537 ) ) ;
#17150=B_SPLINE_CURVE_WITH_KNOTS ( 'NONE', 3,
 ( #23792, #26798, #10810, #23579, #11226, #14414, #36813, #36399, #17821, #33826, #27421, #4449, #30613, #40435, #39807, #33201, #30197, #21014 ),
 .UNSPECIFIED., .F., .F.,
 ( 4, 2, 1, 1, 2, 2, 2, 2, 2, 4 ),
 ( -5.999999999820153193E-08, 0.0006526371903139581345, 0.001305334380627914612, 0.002610728761255789402, 0.003916123141883664192, 0.005221517522511539416, 0.01044309504502295531, 0.01305388380627865198, 0.01566467256753434692, 0.02088625009004572639 ),
 .UNSPECIFIED. ) ;
#17151=CARTESIAN_POINT ( 'NONE',  ( -23.91048590848665611, 81.84235438443283783, -1.524000000000006239 ) ) ;
#17154=VECTOR ( 'NONE', #37970, 1000.000000000000227 ) ;
#17159=CARTESIAN_POINT ( 'NONE',  ( -46.91190649557952952, 20.26356613537010887, -4.963267847376400255 ) ) ;
#17161=TOROIDAL_SURFACE ( 'NONE', #8997, 0.7620000000000000107, 0.2540000000000000036 ) ;
#17162=EDGE_CURVE ( 'NONE', #14331, #15131, #6165, .T. ) ;
#17166=CARTESIAN_POINT ( 'NONE',  ( -46.78089565521672455, 25.32111429335394348, -1.738356225806591882 ) ) ;
#17168=DIRECTION ( 'NONE',  ( -0.6825627711659328911, -0.7308269722843309113, -2.299753143848213649E-16 ) ) ;
#17172=CARTESIAN_POINT ( 'NONE',  ( -41.09676540851937432, 23.04694042099054840, 1.523999999999987587 ) ) ;
#17183=CARTESIAN_POINT ( 'NONE',  ( -58.80981292533109439, -0.2807566353365542611, -0.1195710083432118126 ) ) ;
#17192=CARTESIAN_POINT ( 'NONE',  ( -42.04985097881080236, 22.19100705996942935, 1.479702663569726573 ) ) ;
#17194=ORIENTED_EDGE ( 'NONE', *, *, #33957, .F. ) ;
#17198=LINE ( 'NONE', #7839, #29343 ) ;
#17204=EDGE_CURVE ( 'NONE', #29982, #2001, #35432, .T. ) ;
#17207=CARTESIAN_POINT ( 'NONE',  ( -53.65353144418239140, 9.505953006310818409, 3.603183245156613701 ) ) ;
#17208=CARTESIAN_POINT ( 'NONE',  ( -50.64083583777225073, 22.17031204481727258, 0.3653657693499628989 ) ) ;
#17210=CARTESIAN_POINT ( 'NONE',  ( -55.41603145274652320, 6.826612083464994818, 3.210495615568572436 ) ) ;
#17211=CARTESIAN_POINT ( 'NONE',  ( -58.62683610494525510, -0.2852240180758755517, 0.3850767576232742018 ) ) ;
#17215=VERTEX_POINT ( 'NONE', #24262 ) ;
#17216=CARTESIAN_POINT ( 'NONE',  ( -46.97515415817095175, 24.89137758704647396, 2.045406795549891577 ) ) ;
#17219=STYLED_ITEM ( 'NONE', ( #4676 ), #24793 ) ;
#17226=ADVANCED_FACE ( 'NONE', ( #7473 ), #36444, .T. ) ;
#17227=CARTESIAN_POINT ( 'NONE',  ( -28.69846420587789737, 77.20784726182124302, 1.523999999999991806 ) ) ;
#17240=CARTESIAN_POINT ( 'NONE',  ( -54.02436534585504546, 7.965282956745534548, 1.622780670314668994 ) ) ;
#17244=EDGE_CURVE ( 'NONE', #28485, #2780, #36651, .T. ) ;
#17247=EDGE_LOOP ( 'NONE', ( #36053, #8824, #13882, #7628 ) ) ;
#17252=ADVANCED_FACE ( 'NONE', ( #17037 ), #10857, .T. ) ;
#17257=AXIS2_PLACEMENT_3D ( 'NONE', #19265, #38461, #12880 ) ;
#17263=CIRCLE ( 'NONE', #17924, 0.7620000000000000107 ) ;
#17272=AXIS2_PLACEMENT_3D ( 'NONE', #12959, #19142, #25953 ) ;
#17275=DIRECTION ( 'NONE',  ( -0.1906721105965031304, 0.9816537812491097359, -2.460754754889605160E-15 ) ) ;
#17276=CARTESIAN_POINT ( 'NONE',  ( -7.772068811996249771, 69.25462295839062676, -1.269999999999995577 ) ) ;
#17284=CARTESIAN_POINT ( 'NONE',  ( -26.51793118801306548, 72.98537704160715123, -1.524000000000006017 ) ) ;
#17285=ORIENTED_EDGE ( 'NONE', *, *, #1985, .T. ) ;
#17287=CIRCLE ( 'NONE', #35001, 0.2540000000000006142 ) ;
#17292=EDGE_LOOP ( 'NONE', ( #10646, #16662, #1556, #6374 ) ) ;
#17296=CARTESIAN_POINT ( 'NONE',  ( -18.19824605342069290, 84.09650579081264254, -1.270000000000003570 ) ) ;
#17299=DIRECTION ( 'NONE',  ( 0.7770581983690701966, -0.6294287539884197979, 8.537024980200731099E-16 ) ) ;
#17307=EDGE_CURVE ( 'NONE', #26127, #38326, #16036, .T. ) ;
#17308=CARTESIAN_POINT ( 'NONE',  ( -58.26714162322902979, -0.07371858623882177053, 0.4245910480440974188 ) ) ;
#17315=CARTESIAN_POINT ( 'NONE',  ( -56.40094345217906380, 3.567796355414390330, -1.062368598836910261 ) ) ;
#17317=DIRECTION ( 'NONE',  ( 5.188838149069472160E-16, -1.699382548006136559E-16, -1.000000000000000000 ) ) ;
#17320=CARTESIAN_POINT ( 'NONE',  ( -29.81988630937914309, 58.80898419542295130, -1.270000000000005347 ) ) ;
#17322=CARTESIAN_POINT ( 'NONE',  ( -46.91730334005650604, 25.06715201186495179, 1.923126375063701321 ) ) ;
#17323=FACE_OUTER_BOUND ( 'NONE', #38297, .T. ) ;
#17324=CARTESIAN_POINT ( 'NONE',  ( -58.57480556029605623, 0.6052348492003173375, 0.1017111358178618558 ) ) ;
#17327=ORIENTED_EDGE ( 'NONE', *, *, #4821, .F. ) ;
#17328=CARTESIAN_POINT ( 'NONE',  ( -57.90853684698416259, 2.514838786807804816, -1.057718660164803538E-14 ) ) ;
#17330=ORIENTED_EDGE ( 'NONE', *, *, #27271, .T. ) ;
#17337=CARTESIAN_POINT ( 'NONE',  ( -31.49167364583235695, 53.84208496817151968, 1.269999999999994245 ) ) ;
#17342=VERTEX_POINT ( 'NONE', #18387 ) ;
#17345=CARTESIAN_POINT ( 'NONE',  ( -57.75430734548803002, 1.036090420344400798, -1.147874199045983312 ) ) ;
#17350=CARTESIAN_POINT ( 'NONE',  ( -45.39816439898302036, 21.06106408185672763, -4.080402960186392036 ) ) ;
#17354=AXIS2_PLACEMENT_3D ( 'NONE', #1164, #27129, #20509 ) ;
#17355=ORIENTED_EDGE ( 'NONE', *, *, #21467, .F. ) ;
#17358=DIRECTION ( 'NONE',  ( -0.8745520943968241312, 0.4849315768086548406, -5.691349986800536046E-16 ) ) ;
#17361=CARTESIAN_POINT ( 'NONE',  ( -56.65231406860745977, 4.194353530936431262, -2.518504496425251205 ) ) ;
#17369=DIRECTION ( 'NONE',  ( -0.8745520943968240202, 0.4849315768086551737, -5.361993529360572958E-16 ) ) ;
#17371=CARTESIAN_POINT ( 'NONE',  ( -58.11144429832071268, 0.1746852717545849254, 0.04262357901407949623 ) ) ;
#17373=AXIS2_PLACEMENT_3D ( 'NONE', #2104, #21243, #14857 ) ;
#17374=ORIENTED_EDGE ( 'NONE', *, *, #20419, .T. ) ;
#17375=CARTESIAN_POINT ( 'NONE',  ( -47.08352113710599696, 24.38425570713750190, -2.219725161937593949 ) ) ;
#17377=CARTESIAN_POINT ( 'NONE',  ( -46.60530155212504866, 26.17382724835478314, -1.524000000000014454 ) ) ;
#17383=FACE_OUTER_BOUND ( 'NONE', #4370, .T. ) ;
#17394=CARTESIAN_POINT ( 'NONE',  ( -47.84756666395259117, 19.38928433903615911, -5.209054514891951371 ) ) ;
#17398=ORIENTED_EDGE ( 'NONE', *, *, #32894, .T. ) ;
#17401=CARTESIAN_POINT ( 'NONE',  ( -46.33290834485666920, 20.59977736898131440, 4.631597800898110684 ) ) ;
#17403=VECTOR ( 'NONE', #41857, 1000.000000000000227 ) ;
#17411=CARTESIAN_POINT ( 'NONE',  ( -25.97603047661466036, 74.27059221564131519, -1.270000000000005791 ) ) ;
#17413=CARTESIAN_POINT ( 'NONE',  ( -29.82321757229076908, 71.17901112636586447, 1.269999999999991802 ) ) ;
#17414=CARTESIAN_POINT ( 'NONE',  ( -57.16753566998470859, 2.297090730223299904, 1.678507472752695184 ) ) ;
#17416=CARTESIAN_POINT ( 'NONE',  ( -58.09657527255103560, 0.9821181129459344294, 1.359330230256424521 ) ) ;
#17417=CARTESIAN_POINT ( 'NONE',  ( -58.59008072161548597, -0.2123309539291723391, 0.4862672643680832629 ) ) ;
#17421=CARTESIAN_POINT ( 'NONE',  ( -47.16890147375937659, 22.20336809214646578, 4.187060126831876339 ) ) ;
#17432=CARTESIAN_POINT ( 'NONE',  ( -47.72737885966184024, 19.53144537861849273, 5.204668046378070123 ) ) ;
#17436=DIRECTION ( 'NONE',  ( 0.4849315768086535638, 0.8745520943968251304, 1.030032898892975065E-16 ) ) ;
#17445=CARTESIAN_POINT ( 'NONE',  ( -49.74050263075070433, 15.22813595918496432, 2.996737790144726965 ) ) ;
#17450=ORIENTED_EDGE ( 'NONE', *, *, #3677, .T. ) ;
#17456=ADVANCED_FACE ( 'NONE', ( #19445 ), #29276, .T. ) ;
#17462=AXIS2_PLACEMENT_3D ( 'NONE', #24629, #8040, #21013 ) ;
#17464=DIRECTION ( 'NONE',  ( 0.9998501190848635423, 0.01731298258487451447, 5.158639060800523934E-16 ) ) ;
#17471=VERTEX_POINT ( 'NONE', #10497 ) ;
#17478=CIRCLE ( 'NONE', #31753, 0.3810000000000000053 ) ;
#17480=DIRECTION ( 'NONE',  ( 5.188838149069472160E-16, -1.699382548006136559E-16, -1.000000000000000000 ) ) ;
#17486=DIRECTION ( 'NONE',  ( -0.6559537821943239866, 0.7548010569845283735, -4.686333752532408853E-16 ) ) ;
#17494=ORIENTED_EDGE ( 'NONE', *, *, #37363, .T. ) ;
#17498=CARTESIAN_POINT ( 'NONE',  ( -45.22172581742046304, 21.28617977371392200, 3.835562958556399504 ) ) ;
#17501=DIRECTION ( 'NONE',  ( -0.8745520943968235761, 0.4849315768086558953, -5.361993529360570985E-16 ) ) ;
#17507=DIRECTION ( 'NONE',  ( 0.7770581983690896255, -0.6294287539883961502, 6.584108293994711875E-16 ) ) ;
#17508=AXIS2_PLACEMENT_3D ( 'NONE', #8601, #21564, #34592 ) ;
#17509=CARTESIAN_POINT ( 'NONE',  ( -58.22800107110067103, 0.01111325675227925469, 0.5047451677687325722 ) ) ;
#17517=DIRECTION ( 'NONE',  ( -0.8745520943968241312, 0.4849315768086548406, -5.691349986800536046E-16 ) ) ;
#17518=CARTESIAN_POINT ( 'NONE',  ( -50.60903162571948855, 13.45680032611325849, -2.107060282091948622 ) ) ;
#17521=CARTESIAN_POINT ( 'NONE',  ( -46.90670141593995623, 25.33105981158402642, -1.751001814892826580 ) ) ;
#17523=CARTESIAN_POINT ( 'NONE',  ( -29.02482657614628536, 65.73348897311412031, -1.524000000000005350 ) ) ;
#17525=CARTESIAN_POINT ( 'NONE',  ( -17.14500000000466784, 71.11999999999886768, -1.270000000000000684 ) ) ;
#17527=CARTESIAN_POINT ( 'NONE',  ( -58.49256177947683000, 0.7572623586737103896, 0.8868308481463905713 ) ) ;
#17530=ORIENTED_EDGE ( 'NONE', *, *, #16245, .T. ) ;
#17531=CARTESIAN_POINT ( 'NONE',  ( -56.90441949580814196, 4.712873715160811550, -1.842411344577102206 ) ) ;
#17533=EDGE_CURVE ( 'NONE', #32851, #10071, #38134, .T. ) ;
#17535=CARTESIAN_POINT ( 'NONE',  ( -46.96000079187034970, 20.35382130790375044, -5.064780906956246831 ) ) ;
#17544=CARTESIAN_POINT ( 'NONE',  ( -49.66173528812303317, 16.83021509124200676, -4.995230413551627002 ) ) ;
#17545=CARTESIAN_POINT ( 'NONE',  ( -30.75918919842648336, 69.77432548395512413, -1.270000000000007567 ) ) ;
#17546=ORIENTED_EDGE ( 'NONE', *, *, #33664, .T. ) ;
#17549=CARTESIAN_POINT ( 'NONE',  ( -57.76679705834290246, 1.009099809236461587, -1.134662844628306910 ) ) ;
#17553=CARTESIAN_POINT ( 'NONE',  ( -48.16508968810062896, 19.01313136326716347, -5.219744232931991412 ) ) ;
#17562=CARTESIAN_POINT ( 'NONE',  ( -54.47970570282438274, 8.083255770631444292, -3.476097746275910172 ) ) ;
#17563=DIRECTION ( 'NONE',  ( -0.5149185422762211362, 0.8572391118119444542, 0.000000000000000000 ) ) ;
#17571=CARTESIAN_POINT ( 'NONE',  ( -44.77556674759998856, 21.10465188057014174, -3.405155276520980934 ) ) ;
#17573=CARTESIAN_POINT ( 'NONE',  ( -57.72731561024291125, 0.8685078910842247701, 0.07340608407945603542 ) ) ;
#17576=CARTESIAN_POINT ( 'NONE',  ( -47.05348687143031583, 24.98710001375500056, -1.566218509541823956 ) ) ;
#17579=ORIENTED_EDGE ( 'NONE', *, *, #17307, .F. ) ;
#17586=EDGE_CURVE ( 'NONE', #5717, #30054, #32021, .T. ) ;
#17591=DIRECTION ( 'NONE',  ( -0.7308269722843310223, 0.6825627711659330021, -4.952078135395968077E-16 ) ) ;
#17597=CARTESIAN_POINT ( 'NONE',  ( -52.86182053368817435, 11.13604294809218587, -4.079049242077941173 ) ) ;
#17602=ORIENTED_EDGE ( 'NONE', *, *, #38480, .T. ) ;
#17604=VECTOR ( 'NONE', #4419, 1000.000000000000000 ) ;
#17606=AXIS2_PLACEMENT_3D ( 'NONE', #41027, #5460, #18420 ) ;
#17607=FACE_OUTER_BOUND ( 'NONE', #19375, .T. ) ;
#17609=ORIENTED_EDGE ( 'NONE', *, *, #21467, .T. ) ;
#17618=FACE_OUTER_BOUND ( 'NONE', #31755, .T. ) ;
#17619=CARTESIAN_POINT ( 'NONE',  ( -53.64375852056468830, 9.525086444836489363, 3.607221310910125656 ) ) ;
#17622=CARTESIAN_POINT ( 'NONE',  ( -58.07447437077728125, 1.735896131820596766, 1.499107834811089113 ) ) ;
#17623=CARTESIAN_POINT ( 'NONE',  ( -58.65177056075324202, -0.3162497232223037136, 0.3274186093513313800 ) ) ;
#17626=EDGE_LOOP ( 'NONE', ( #12875, #40411, #28350, #12941 ) ) ;
#17627=CARTESIAN_POINT ( 'NONE',  ( -47.35944255389382818, 21.37623662739424191, 4.722871667523163453 ) ) ;
#17628=AXIS2_PLACEMENT_3D ( 'NONE', #34637, #25038, #38041 ) ;
#17639=CARTESIAN_POINT ( 'NONE',  ( -47.85244527695894590, 19.39403540832958583, 5.219971639306684175 ) ) ;
#17642=DIRECTION ( 'NONE',  ( 0.000000000000000000, 0.000000000000000000, -1.000000000000000000 ) ) ;
#17644=DIRECTION ( 'NONE',  ( -0.4849315768086480127, -0.8745520943968279060, -1.030032898892941415E-16 ) ) ;
#17651=ORIENTED_EDGE ( 'NONE', *, *, #5123, .T. ) ;
#17652=CARTESIAN_POINT ( 'NONE',  ( -49.01239152747368166, 15.29178156536908872, 1.600675721865261858 ) ) ;
#17657=ORIENTED_EDGE ( 'NONE', *, *, #9963, .T. ) ;
#17663=ORIENTED_EDGE ( 'NONE', *, *, #4277, .T. ) ;
#17670=DIRECTION ( 'NONE',  ( 5.188838149069472160E-16, -1.699382548006136559E-16, -1.000000000000000000 ) ) ;
#17683=DIRECTION ( 'NONE',  ( -0.8745520943968240202, 0.4849315768086553402, -5.361993529360572958E-16 ) ) ;
#17690=EDGE_LOOP ( 'NONE', ( #12683, #18050, #7715, #36547, #26073 ) ) ;
#17695=ORIENTED_EDGE ( 'NONE', *, *, #29205, .F. ) ;
#17714=CARTESIAN_POINT ( 'NONE',  ( -58.16644339752579640, 0.1874380212899332265, 0.9010643025995082045 ) ) ;
#17721=DIRECTION ( 'NONE',  ( 5.188838149069472160E-16, -1.699382548006136559E-16, -1.000000000000000000 ) ) ;
#17722=CARTESIAN_POINT ( 'NONE',  ( -57.74348367832291018, 0.8661236967133778553, -0.1780388485286305555 ) ) ;
#17725=CARTESIAN_POINT ( 'NONE',  ( -46.84474875364813329, 25.59693625086653412, -1.568125628604711608 ) ) ;
#17728=CIRCLE ( 'NONE', #28627, 0.2539999999999992264 ) ;
#17732=CARTESIAN_POINT ( 'NONE',  ( -58.08922378330620973, 1.909136410080003454, 0.4248916911265161467 ) ) ;
#17734=CARTESIAN_POINT ( 'NONE',  ( -58.87911280034276018, -0.2081424763510641984, -1.061797465414398100E-14 ) ) ;
#17736=ORIENTED_EDGE ( 'NONE', *, *, #37350, .F. ) ;
#17737=CARTESIAN_POINT ( 'NONE',  ( -57.71825614945207406, 2.868614883688350048, -0.7691332274306353911 ) ) ;
#17739=CARTESIAN_POINT ( 'NONE',  ( -44.18728704178806765, 21.36917510655693420, -3.097942224162511415 ) ) ;
#17747=CARTESIAN_POINT ( 'NONE',  ( -50.68868110200592980, 15.17409885929999902, -4.768265622168934570 ) ) ;
#17748=ADVANCED_FACE ( 'NONE', ( #18977 ), #9199, .T. ) ;
#17751=CARTESIAN_POINT ( 'NONE',  ( -54.28365971233007059, 8.261047645289938401, -3.332732081090967746 ) ) ;
#17754=CARTESIAN_POINT ( 'NONE',  ( -44.66298991629287940, 23.47648082339880915, -1.964675176939946644 ) ) ;
#17757=EDGE_CURVE ( 'NONE', #16319, #18538, #8202, .T. ) ;
#17763=ADVANCED_FACE ( 'NONE', ( #12180 ), #28785, .F. ) ;
#17764=CARTESIAN_POINT ( 'NONE',  ( -56.22331024217277928, 5.808995339285999648, -2.850545730341259798 ) ) ;
#17768=EDGE_CURVE ( 'NONE', #28485, #19344, #19085, .T. ) ;
#17769=CIRCLE ( 'NONE', #812, 0.3810000000000015041 ) ;
#17774=CARTESIAN_POINT ( 'NONE',  ( -8.336765840796966032, 73.19241104973453105, 1.270000000000001572 ) ) ;
#17775=CARTESIAN_POINT ( 'NONE',  ( -42.01646181069634878, 22.10209156318453694, -0.7046475714187767636 ) ) ;
#17776=VECTOR ( 'NONE', #29430, 1000.000000000000227 ) ;
#17778=CARTESIAN_POINT ( 'NONE',  ( -58.33591949829837375, -0.2304704932390572170, 0.1444701089452633536 ) ) ;
#17781=CARTESIAN_POINT ( 'NONE',  ( -47.14788814370446346, 23.76379789425250166, -2.690610990139723491 ) ) ;
#17791=AXIS2_PLACEMENT_3D ( 'NONE', #29901, #36509, #3298 ) ;
#17794=ORIENTED_EDGE ( 'NONE', *, *, #10577, .T. ) ;
#17798=CARTESIAN_POINT ( 'NONE',  ( -43.55282861522693594, 21.75186539808470698, -2.470256665153925724 ) ) ;
#17799=EDGE_LOOP ( 'NONE', ( #5645, #35695, #18483, #33085 ) ) ;
#17805=CARTESIAN_POINT ( 'NONE',  ( -58.63158931450414002, -0.2944865825844911189, -0.3706283016938188846 ) ) ;
#17815=DIRECTION ( 'NONE',  ( 5.188838149069472160E-16, -1.699382548006136559E-16, -1.000000000000000000 ) ) ;
#17819=CARTESIAN_POINT ( 'NONE',  ( -30.75918919842648336, 69.77432548395512413, -1.270000000000007567 ) ) ;
#17821=CARTESIAN_POINT ( 'NONE',  ( -29.24376532021898356, 65.27002024517358336, -1.270000000000005791 ) ) ;
#17822=AXIS2_PLACEMENT_3D ( 'NONE', #26657, #10468, #19207 ) ;
#17831=CARTESIAN_POINT ( 'NONE',  ( -56.09991784293080030, 4.552033362070804223, 2.401778663949239778 ) ) ;
#17832=CARTESIAN_POINT ( 'NONE',  ( -48.75791856165849936, 18.18949858612532466, 5.155209323065509608 ) ) ;
#17833=LINE ( 'NONE', #6281, #7603 ) ;
#17837=CARTESIAN_POINT ( 'NONE',  ( -51.34009458250667279, 14.66650723912346699, 4.800162786360129274 ) ) ;
#17842=CARTESIAN_POINT ( 'NONE',  ( -29.57045817531687959, 58.76046099849394011, 1.523999999999993138 ) ) ;
#17844=EDGE_LOOP ( 'NONE', ( #955, #21299 ) ) ;
#17847=DIRECTION ( 'NONE',  ( 0.8745520943968240202, -0.4849315768086553402, 6.829619984160650158E-16 ) ) ;
#17848=CARTESIAN_POINT ( 'NONE',  ( -47.59852559863926302, 19.66225068540052945, 5.176489187661841740 ) ) ;
#17849=LINE ( 'NONE', #24242, #40587 ) ;
#17859=CIRCLE ( 'NONE', #25346, 8.794750000000000512 ) ;
#17862=CARTESIAN_POINT ( 'NONE',  ( -48.90916507497669841, 16.41193755240580288, 3.099911505780750254 ) ) ;
#17866=VERTEX_POINT ( 'NONE', #6837 ) ;
#17872=ORIENTED_EDGE ( 'NONE', *, *, #12340, .F. ) ;
#17875=CARTESIAN_POINT ( 'NONE',  ( -18.58115504727956591, 80.30342350548193053, 1.523999999999996247 ) ) ;
#17876=EDGE_CURVE ( 'NONE', #40376, #37721, #34097, .T. ) ;
#17879=CARTESIAN_POINT ( 'NONE',  ( -29.89586364642803318, 71.55302121702176521, 1.269999999999991802 ) ) ;
#17880=AXIS2_PLACEMENT_3D ( 'NONE', #12717, #38712, #6339 ) ;
#17883=CARTESIAN_POINT ( 'NONE',  ( -24.26619908708081041, 81.70586579672512073, 1.523999999999993138 ) ) ;
#17886=ORIENTED_EDGE ( 'NONE', *, *, #17099, .T. ) ;
#17887=ORIENTED_EDGE ( 'NONE', *, *, #10758, .T. ) ;
#17894=VECTOR ( 'NONE', #4615, 1000.000000000000227 ) ;
#17916=AXIS2_PLACEMENT_3D ( 'NONE', #15014, #21391, #30998 ) ;
#17920=AXIS2_PLACEMENT_3D ( 'NONE', #23786, #4231, #7833 ) ;
#17922=ORIENTED_EDGE ( 'NONE', *, *, #10763, .T. ) ;
#17924=AXIS2_PLACEMENT_3D ( 'NONE', #18501, #2770, #2565 ) ;
#17925=CARTESIAN_POINT ( 'NONE',  ( -58.40429423216560423, -0.3346038877926625354, 0.4235997928849980498 ) ) ;
#17930=VECTOR ( 'NONE', #30107, 1000.000000000000000 ) ;
#17931=EDGE_CURVE ( 'NONE', #5200, #24894, #16407, .T. ) ;
#17935=CARTESIAN_POINT ( 'NONE',  ( -58.24002838079472610, 0.001074765447070524793, -0.6562585879479864159 ) ) ;
#17938=TOROIDAL_SURFACE ( 'NONE', #41788, 0.8889999999999989022, 0.2540000000000000036 ) ;
#17939=CYLINDRICAL_SURFACE ( 'NONE', #28036, 0.2539999999999937863 ) ;
#17941=DIRECTION ( 'NONE',  ( -5.188838149069472160E-16, 1.699382548006136559E-16, 1.000000000000000000 ) ) ;
#17946=CARTESIAN_POINT ( 'NONE',  ( -58.37241122568488549, -0.2962816677227753104, -1.034007718770489626E-14 ) ) ;
#17948=ORIENTED_EDGE ( 'NONE', *, *, #31348, .F. ) ;
#17949=CARTESIAN_POINT ( 'NONE',  ( -58.83227707057486811, -0.08366279997995551554, -5.952756869281050995E-15 ) ) ;
#17951=ORIENTED_EDGE ( 'NONE', *, *, #458, .F. ) ;
#17952=CARTESIAN_POINT ( 'NONE',  ( -46.53702275532300092, 20.69065974945478104, -4.840627275220472647 ) ) ;
#17960=CARTESIAN_POINT ( 'NONE',  ( -48.62040608122599394, 18.38533207009528070, -5.173709449133584215 ) ) ;
#17963=CARTESIAN_POINT ( 'NONE',  ( -20.21600168833980149, 80.16988503754176065, -1.270000000000003793 ) ) ;
#17965=CARTESIAN_POINT ( 'NONE',  ( -48.83525966142772745, 18.03881763506669955, -5.101163988045986031 ) ) ;
#17968=CIRCLE ( 'NONE', #41807, 0.2539999999999942859 ) ;
#17970=CARTESIAN_POINT ( 'NONE',  ( -48.53848336910535011, 19.22582880449973075, -5.323527254358048744 ) ) ;
#17972=ORIENTED_EDGE ( 'NONE', *, *, #6532, .T. ) ;
#17977=EDGE_CURVE ( 'NONE', #35748, #33508, #1449, .T. ) ;
#17978=CARTESIAN_POINT ( 'NONE',  ( -57.36719850051837000, 1.975114663830185302, -1.756955940785672077 ) ) ;
#17984=CARTESIAN_POINT ( 'NONE',  ( -58.50860430493789721, 0.7049166599848305514, -0.9756837515128595761 ) ) ;
#17985=CARTESIAN_POINT ( 'NONE',  ( -43.98989719630797168, 21.38545485255711398, -2.905481552205971596 ) ) ;
#17988=B_SPLINE_CURVE_WITH_KNOTS ( 'NONE', 3,
 ( #32555, #6371, #38747, #9972, #29789, #416, #23372, #26373, #19341, #32347, #41951, #39381, #26587, #3608, #10184, #39165, #16355, #29142, #23153, #42159, #3824, #36190, #13598, #12954, #9554, #35762, #3390, #22526, #29362, #36405, #19138, #32142, #2974, #36820, #4245, #4872, #37230, #7639, #14009, #10818, #7430, #4033, #17619, #27633, #17207, #30411, #11031, #8048, #20598, #4663, #833, #1259, #21021, #17831, #34044, #33629, #36611, #26806, #40236, #30828, #30621, #4457, #23801, #13808, #17414, #14213, #27223, #11235, #27430, #1676, #39814, #7848, #1045, #27016, #24012, #37032, #20809, #33835, #30205, #10607, #40024, #33208, #14631, #1464, #20388, #23588, #14422, #40644, #33413, #40443, #11438, #24219, #24426, #7222, #20183, #16994, #29993, #5713, #15683, #34458, #18454, #15049, #28051, #18669, #11653, #35096, #14839, #21224, #5493, #28267, #31459, #8887, #25068, #24638, #24860, #2303, #2516, #31676, #15263, #37856, #37649, #12079, #38071, #34880, #15480, #2725, #8679, #28481, #9105, #41274, #21641, #41060, #1877, #11870, #41486, #12506, #34665, #12293, #28687, #8474, #25281, #21852, #38285, #21430, #22069, #5084, #5291, #31889, #18036, #18240, #5918, #18880, #41695, #37431, #8252, #31242, #34255, #2086, #31037, #27844, #40851, #38913, #374, #19936, #22275, #6330, #16741, #15893 ),
 .UNSPECIFIED., .F., .F.,
 ( 4, 2, 2, 2, 2, 1, 1, 1, 2, 2, 2, 1, 1, 1, 1, 2, 2, 2, 1, 2, 2, 1, 1, 1, 1, 1, 1, 1, 1, 2, 2, 2, 2, 2, 1, 1, 1, 1, 1, 2, 2, 2, 2, 2, 2, 2, 2, 2, 2, 2, 1, 2, 2, 2, 2, 2, 1, 1, 1, 2, 2, 2, 2, 2, 2, 2, 2, 1, 2, 2, 2, 2, 1, 2, 2, 2, 2, 1, 1, 1, 2, 2, 2, 1, 1, 1, 2, 2, 2, 2, 1, 2, 2, 2, 1, 2, 2, 2, 1, 2, 2, 4 ),
 ( 0.000000000000000000, 0.03124999999999582972, 0.06249999999999165945, 0.07031249999999060474, 0.07226562499999056310, 0.07421874999999052147, 0.07812499999999043820, 0.09374999999998993860, 0.1249999999999889533, 0.1874999999999869826, 0.2187499999999860112, 0.2343749999999854006, 0.2421874999999849842, 0.2460937499999849842, 0.2480468749999849565, 0.2490234374999850675, 0.2499999999999851230, 0.3749999999999627520, 0.3906249999999598654, 0.3925781249999596989, 0.3945312499999595879, 0.3984374999999594769, 0.4062499999999596434, 0.4374999999999604761, 0.4687499999999613087, 0.4843749999999614753, 0.4921874999999617528, 0.4960937499999616418, 0.4980468749999616418, 0.4990234374999615863, 0.4999999999999615863, 0.6249999999999517053, 0.6874999999999467093, 0.7187499999999442668, 0.7343749999999431566, 0.7421874999999427125, 0.7460937499999424904, 0.7480468749999424904, 0.7490234374999424904, 0.7495117187499424904, 0.7499999999999424904, 0.8124999999999656941, 0.8437499999999771294, 0.8593749999999827915, 0.8671874999999856781, 0.8710937499999867883, 0.8749999999999878986, 0.8906249999999940048, 0.8984374999999971134, 0.9003906249999981126, 0.9023437499999990008, 0.9062500000000008882, 0.9140625000000045519, 0.9179687500000063283, 0.9218750000000079936, 0.9296875000000117684, 0.9335937500000134337, 0.9355468750000140998, 0.9365234375000144329, 0.9370117187500146549, 0.9375000000000147660, 0.9414062500000129896, 0.9433593750000121014, 0.9443359375000116573, 0.9453125000000112133, 0.9492187500000097700, 0.9511718750000092149, 0.9521484375000092149, 0.9526367187500092149, 0.9531250000000092149, 0.9609375000000078826, 0.9648437500000073275, 0.9667968750000069944, 0.9677734375000067724, 0.9687500000000065503, 0.9765625000000043299, 0.9804687500000031086, 0.9824218750000025535, 0.9833984375000022204, 0.9838867187500022204, 0.9841308593750023315, 0.9843750000000024425, 0.9882812500000022204, 0.9902343750000021094, 0.9912109375000021094, 0.9916992187500019984, 0.9919433593750019984, 0.9921875000000018874, 0.9941406250000014433, 0.9951171875000012212, 0.9956054687500011102, 0.9958496093750011102, 0.9960937500000011102, 0.9970703125000007772, 0.9975585937500005551, 0.9978027343750005551, 0.9980468750000004441, 0.9985351562500003331, 0.9987792968750002220, 0.9989013671875002220, 0.9990234375000002220, 1.000000000000000000 ),
 .UNSPECIFIED. ) ;
#17989=CARTESIAN_POINT ( 'NONE',  ( -57.57967628038989005, 1.451576601202167360, 1.494865757154131947 ) ) ;
#17990=CARTESIAN_POINT ( 'NONE',  ( -52.06588384925056801, 19.72955628943436679, -1.003574140810235308E-14 ) ) ;
#17992=ORIENTED_EDGE ( 'NONE', *, *, #32093, .F. ) ;
#17993=CARTESIAN_POINT ( 'NONE',  ( -49.37240900658670739, 23.24656341648388036, -0.6295958749597222459 ) ) ;
#18003=LINE ( 'NONE', #5887, #21669 ) ;
#18007=CARTESIAN_POINT ( 'NONE',  ( -45.22172561961857440, 21.28617983374608613, -3.835562791334466315 ) ) ;
#18012=DIRECTION ( 'NONE',  ( -0.8745520943968053684, 0.4849315768086885359, -5.691349986800504491E-16 ) ) ;
#18014=CARTESIAN_POINT ( 'NONE',  ( -52.79140191242705527, 11.19429870261168958, -3.959798436811984512 ) ) ;
#18022=DIRECTION ( 'NONE',  ( -0.8745520943968250194, 0.4849315768086532863, -5.361993529360574930E-16 ) ) ;
#18026=DIRECTION ( 'NONE',  ( -5.188838149069472160E-16, 1.699382548006136559E-16, 1.000000000000000000 ) ) ;
#18033=CIRCLE ( 'NONE', #18704, 0.5080000000000016724 ) ;
#18035=CARTESIAN_POINT ( 'NONE',  ( -24.26619908708080686, 81.70586579672512073, -1.270000000000006235 ) ) ;
#18036=CARTESIAN_POINT ( 'NONE',  ( -58.36351474529333672, -0.2784124508822488631, 0.09868539478380247698 ) ) ;
#18038=CARTESIAN_POINT ( 'NONE',  ( -51.05013135955051951, 14.56862583435632530, 4.678276857666586075 ) ) ;
#18044=CARTESIAN_POINT ( 'NONE',  ( -49.39021242113546606, 17.77731941784099234, 5.290631085210035778 ) ) ;
#18050=ORIENTED_EDGE ( 'NONE', *, *, #1565, .T. ) ;
#18053=CARTESIAN_POINT ( 'NONE',  ( -17.64290547347870941, 83.78857423953914463, 1.269999999999996021 ) ) ;
#18054=CARTESIAN_POINT ( 'NONE',  ( -46.78765925928225755, 20.34570826442007174, 4.900687844021624606 ) ) ;
#18055=DIRECTION ( 'NONE',  ( 5.188838149069472160E-16, -1.699382548006136559E-16, -1.000000000000000000 ) ) ;
#18060=FACE_OUTER_BOUND ( 'NONE', #12350, .T. ) ;
#18068=VERTEX_POINT ( 'NONE', #3655 ) ;
#18069=CARTESIAN_POINT ( 'NONE',  ( -52.82621711067185544, 9.762356329794503296, 1.302233150175811094 ) ) ;
#18070=AXIS2_PLACEMENT_3D ( 'NONE', #4216, #33381, #6979 ) ;
#18082=CARTESIAN_POINT ( 'NONE',  ( -35.99603394726484851, 64.04701136959550922, -1.270000000000009344 ) ) ;
#18088=CARTESIAN_POINT ( 'NONE',  ( -43.82859865241511699, 24.63416949198730421, 1.523999999999993138 ) ) ;
#18091=EDGE_CURVE ( 'NONE', #4125, #32297, #39216, .T. ) ;
#18093=VECTOR ( 'NONE', #5863, 1000.000000000000114 ) ;
#18104=CARTESIAN_POINT ( 'NONE',  ( -17.64290547347870941, 83.78857423953914463, -1.524000000000003130 ) ) ;
#18115=EDGE_CURVE ( 'NONE', #31840, #37188, #13439, .T. ) ;
#18117=ORIENTED_EDGE ( 'NONE', *, *, #2385, .T. ) ;
#18126=DIRECTION ( 'NONE',  ( 5.188838149069472160E-16, -1.699382548006136559E-16, -1.000000000000000000 ) ) ;
#18129=CIRCLE ( 'NONE', #21525, 0.2540000000000006142 ) ;
#18130=VERTEX_POINT ( 'NONE', #25998 ) ;
#18133=CARTESIAN_POINT ( 'NONE',  ( -57.50985127144491571, 1.621858126761932084, 1.632528232186438721 ) ) ;
#18142=CARTESIAN_POINT ( 'NONE',  ( -57.61542428582638564, 1.103772655929896596, -0.1998674755708677864 ) ) ;
#18145=DIRECTION ( 'NONE',  ( 5.188838149069472160E-16, -1.699382548006136559E-16, -1.000000000000000000 ) ) ;
#18146=DIRECTION ( 'NONE',  ( -0.9998501190848635423, -0.01731298258487451447, -5.158639060800523934E-16 ) ) ;
#18151=CARTESIAN_POINT ( 'NONE',  ( -58.83227707057488232, -0.08366279997998327111, -1.543674587295873857E-14 ) ) ;
#18154=VECTOR ( 'NONE', #5615, 1000.000000000000000 ) ;
#18156=CARTESIAN_POINT ( 'NONE',  ( -58.60381103753274346, 0.5214191424347813797, -0.2072982876684605347 ) ) ;
#18158=FACE_OUTER_BOUND ( 'NONE', #11905, .T. ) ;
#18165=CARTESIAN_POINT ( 'NONE',  ( -50.50202955377455538, 15.48282070406618338, -4.812845866082358981 ) ) ;
#18166=VERTEX_POINT ( 'NONE', #39007 ) ;
#18168=DIRECTION ( 'NONE',  ( 0.7548010569845216011, 0.6559537821943317581, 2.801824109679580762E-16 ) ) ;
#18170=CARTESIAN_POINT ( 'NONE',  ( -54.85593356636119466, 7.111675983978352100, -3.067722010356754403 ) ) ;
#18173=CARTESIAN_POINT ( 'NONE',  ( -55.11216289415786207, 6.786895728730008237, -3.177266426849177705 ) ) ;
#18176=ORIENTED_EDGE ( 'NONE', *, *, #36658, .T. ) ;
#18180=CARTESIAN_POINT ( 'NONE',  ( -57.43854689232674815, 1.757847328446624058, -1.624773336220253217 ) ) ;
#18182=DIRECTION ( 'NONE',  ( -0.8745520943968241312, 0.4849315768086548406, -5.691349986800536046E-16 ) ) ;
#18189=DIRECTION ( 'NONE',  ( -0.5149185422762213582, 0.8572391118119444542, 6.416759367969739335E-15 ) ) ;
#18191=CARTESIAN_POINT ( 'NONE',  ( -6.559134203278485842, 78.24119908707510263, 1.270000000000002682 ) ) ;
#18193=CARTESIAN_POINT ( 'NONE',  ( -57.80191396384030611, 0.8575073823135492823, 0.7186190270693690874 ) ) ;
#18194=CARTESIAN_POINT ( 'NONE',  ( -49.65119436432973998, 19.91503915004672720, 3.137105223390890263 ) ) ;
#18197=CARTESIAN_POINT ( 'NONE',  ( -51.02231935970569054, 20.76374992004582154, -0.7877321375940368187 ) ) ;
#18205=CARTESIAN_POINT ( 'NONE',  ( -8.216341275949833545, 69.50096819940942794, 1.270000000000003348 ) ) ;
#18211=CARTESIAN_POINT ( 'NONE',  ( -42.24009380985435058, 22.39526060921979678, -1.717801299055324415 ) ) ;
#18212=DIRECTION ( 'NONE',  ( -0.8572391118119510045, -0.5149185422762100339, -3.573031421855330583E-16 ) ) ;
#18215=DIRECTION ( 'NONE',  ( 0.6594218222380271444, 0.7517731442105921591, -2.068700233264622195E-15 ) ) ;
#18217=CARTESIAN_POINT ( 'NONE',  ( -58.41956937744169664, -0.3672969284050977001, -0.3776070891688105280 ) ) ;
#18227=DIRECTION ( 'NONE',  ( -0.8745520943968240202, 0.4849315768086551737, -5.361993529360572958E-16 ) ) ;
#18239=VECTOR ( 'NONE', #36039, 1000.000000000000000 ) ;
#18240=CARTESIAN_POINT ( 'NONE',  ( -58.36378379890241774, -0.2789760973723339754, 0.09651987913409887376 ) ) ;
#18241=CARTESIAN_POINT ( 'NONE',  ( -30.30981065340567682, 56.20484928103341815, -1.524000000000004462 ) ) ;
#18245=ORIENTED_EDGE ( 'NONE', *, *, #6574, .F. ) ;
#18246=CARTESIAN_POINT ( 'NONE',  ( -48.56815661899837977, 19.24492339269602681, 5.224590812749973168 ) ) ;
#18255=ORIENTED_EDGE ( 'NONE', *, *, #25087, .T. ) ;
#18257=CARTESIAN_POINT ( 'NONE',  ( -17.14500000000466784, 71.11999999999886768, -1.270000000000000684 ) ) ;
#18258=DIRECTION ( 'NONE',  ( 5.188838149069472160E-16, -1.699382548006136559E-16, -1.000000000000000000 ) ) ;
#18259=CYLINDRICAL_SURFACE ( 'NONE', #4749, 9.048749999999998295 ) ;
#18262=CIRCLE ( 'NONE', #22324, 0.3810000000000015041 ) ;
#18269=AXIS2_PLACEMENT_3D ( 'NONE', #20518, #11157, #36329 ) ;
#18274=EDGE_CURVE ( 'NONE', #32282, #19659, #23203, .T. ) ;
#18275=CARTESIAN_POINT ( 'NONE',  ( -56.88731995051697510, 2.378615435641926013, -9.753004163756391309E-15 ) ) ;
#18288=ADVANCED_FACE ( 'NONE', ( #35814 ), #17083, .T. ) ;
#18297=LINE ( 'NONE', #31296, #36862 ) ;
#18300=DIRECTION ( 'NONE',  ( 0.8745520943968235761, -0.4849315768086558398, 4.268512490100410909E-16 ) ) ;
#18306=CYLINDRICAL_SURFACE ( 'NONE', #9089, 9.048749999999998295 ) ;
#18307=CARTESIAN_POINT ( 'NONE',  ( -52.32205026661357294, 13.67230311332622072, 4.407798173677520914 ) ) ;
#18313=CARTESIAN_POINT ( 'NONE',  ( -17.64950171984354199, 84.16951713491046405, -1.270000000000003126 ) ) ;
#18318=ORIENTED_EDGE ( 'NONE', *, *, #564, .F. ) ;
#18324=VERTEX_POINT ( 'NONE', #30666 ) ;
#18325=TOROIDAL_SURFACE ( 'NONE', #19698, 0.7620000000000000107, 0.2540000000000000036 ) ;
#18341=CARTESIAN_POINT ( 'NONE',  ( -5.885917553499150578, 77.12042444889114279, 1.270000000000003348 ) ) ;
#18343=CARTESIAN_POINT ( 'NONE',  ( -48.99983924689409065, 17.84334367881407957, 5.121602422844266478 ) ) ;
#18352=CARTESIAN_POINT ( 'NONE',  ( -57.56998337575458891, 1.440017903778734176, -1.358936928125946242 ) ) ;
#18356=DIRECTION ( 'NONE',  ( -0.8745520943968229099, 0.4849315768086570055, -5.361993529360569999E-16 ) ) ;
#18360=FACE_OUTER_BOUND ( 'NONE', #39293, .T. ) ;
#18364=CARTESIAN_POINT ( 'NONE',  ( -58.55612285180489351, 0.6590214021355567109, -1.070617094346549358E-14 ) ) ;
#18366=CARTESIAN_POINT ( 'NONE',  ( -42.61647787783741137, 21.91010357080785198, -1.992259954791246956 ) ) ;
#18373=CARTESIAN_POINT ( 'NONE',  ( -48.70299960009106854, 18.26799440206204039, -5.162729530914248244 ) ) ;
#18374=ORIENTED_EDGE ( 'NONE', *, *, #16231, .T. ) ;
#18376=DIRECTION ( 'NONE',  ( -0.8745520943968240202, 0.4849315768086551737, -5.361993529360572958E-16 ) ) ;
#18378=CARTESIAN_POINT ( 'NONE',  ( -50.98289254807885129, 14.49328483455382788, -4.546320080528299279 ) ) ;
#18380=AXIS2_PLACEMENT_3D ( 'NONE', #2351, #15096, #31503 ) ;
#18382=CARTESIAN_POINT ( 'NONE',  ( -54.77668461537430034, 8.146287316968315650, -3.518595155146543529 ) ) ;
#18387=CARTESIAN_POINT ( 'NONE',  ( -46.60530155212503445, 26.17382724835477958, -1.270000000000008233 ) ) ;
#18388=AXIS2_PLACEMENT_3D ( 'NONE', #36972, #11177, #20755 ) ;
#18389=CARTESIAN_POINT ( 'NONE',  ( -58.30521585032268206, -0.1116666926106041347, -0.6575736669891941721 ) ) ;
#18392=CYLINDRICAL_SURFACE ( 'NONE', #16467, 0.2540000000000006142 ) ;
#18393=ADVANCED_FACE ( 'NONE', ( #21068 ), #27480, .F. ) ;
#18398=CARTESIAN_POINT ( 'NONE',  ( -8.270297712355500153, 69.35377921309405735, 1.270000000000002460 ) ) ;
#18399=CARTESIAN_POINT ( 'NONE',  ( -42.93826774478920072, 21.39662913260299959, -1.244340269653810394 ) ) ;
#18403=CARTESIAN_POINT ( 'NONE',  ( -58.87911280034276018, -0.2081424763510641984, -1.061797465414398100E-14 ) ) ;
#18404=DIRECTION ( 'NONE',  ( -0.8745520943968243532, 0.4849315768086547296, -5.361993529360573944E-16 ) ) ;
#18405=DIRECTION ( 'NONE',  ( -5.188838149069471174E-16, 1.699382548006136313E-16, 1.000000000000000000 ) ) ;
#18406=CARTESIAN_POINT ( 'NONE',  ( -48.20156657701304681, 19.76063879377972654, 5.201425424509390716 ) ) ;
#18408=ORIENTED_EDGE ( 'NONE', *, *, #13078, .T. ) ;
#18409=CARTESIAN_POINT ( 'NONE',  ( -48.69154271504742582, 20.42972839736894386, -3.938715850604340041 ) ) ;
#18412=ORIENTED_EDGE ( 'NONE', *, *, #6562, .T. ) ;
#18420=DIRECTION ( 'NONE',  ( -0.8745520943968253524, 0.4849315768086530087, -4.268512490100385764E-16 ) ) ;
#18423=CARTESIAN_POINT ( 'NONE',  ( -41.26650596300371632, 23.23696532716443741, -1.524000000000029775 ) ) ;
#18425=ORIENTED_EDGE ( 'NONE', *, *, #21856, .T. ) ;
#18427=DIRECTION ( 'NONE',  ( -0.4849315768086480127, -0.8745520943968279060, -1.030032898892941415E-16 ) ) ;
#18433=CIRCLE ( 'NONE', #5540, 0.3810000000000015041 ) ;
#18439=CIRCLE ( 'NONE', #22525, 0.5080000000000000071 ) ;
#18442=ORIENTED_EDGE ( 'NONE', *, *, #19832, .T. ) ;
#18445=TOROIDAL_SURFACE ( 'NONE', #23898, 0.3809999999999997278, 0.2540000000000000036 ) ;
#18454=CARTESIAN_POINT ( 'NONE',  ( -57.97322207812975137, 0.5626473900411875784, 0.8941911358200723692 ) ) ;
#18456=VECTOR ( 'NONE', #31246, 1000.000000000000000 ) ;
#18457=DIRECTION ( 'NONE',  ( 0.9807655518882848478, -0.1951894777626808908, 8.537024980200819846E-16 ) ) ;
#18460=EDGE_LOOP ( 'NONE', ( #36724, #3306, #41476, #24106 ) ) ;
#18461=CARTESIAN_POINT ( 'NONE',  ( -48.98489377192316852, 18.65252824715059177, 5.272350768541908650 ) ) ;
#18463=TOROIDAL_SURFACE ( 'NONE', #4130, 0.7620000000000000107, 0.2540000000000000036 ) ;
#18469=CARTESIAN_POINT ( 'NONE',  ( -28.99017888285159117, 62.64366196047017610, 1.523999999999993804 ) ) ;
#18470=DIRECTION ( 'NONE',  ( -0.8745520943968243532, 0.4849315768086547296, -5.361993529360573944E-16 ) ) ;
#18483=ORIENTED_EDGE ( 'NONE', *, *, #12274, .F. ) ;
#18484=CARTESIAN_POINT ( 'NONE',  ( -56.40799993875704388, 3.472264316502340797, 0.7602746155037158893 ) ) ;
#18488=VERTEX_POINT ( 'NONE', #17875 ) ;
#18494=ORIENTED_EDGE ( 'NONE', *, *, #11859, .F. ) ;
#18498=EDGE_CURVE ( 'NONE', #20056, #36001, #23857, .T. ) ;
#18501=CARTESIAN_POINT ( 'NONE',  ( -20.21600168833980149, 80.16988503754176065, 1.523999999999995580 ) ) ;
#18508=ORIENTED_EDGE ( 'NONE', *, *, #35252, .F. ) ;
#18518=CARTESIAN_POINT ( 'NONE',  ( -57.93941708942283952, 2.052042089854988483, 1.628789306319508023 ) ) ;
#18519=DIRECTION ( 'NONE',  ( 5.188838149069472160E-16, -1.699382548006136559E-16, -1.000000000000000000 ) ) ;
#18524=DIRECTION ( 'NONE',  ( -0.8745520943968246863, 0.4849315768086538414, -5.122214988120500191E-16 ) ) ;
#18537=AXIS2_PLACEMENT_3D ( 'NONE', #8409, #27993, #24796 ) ;
#18538=VERTEX_POINT ( 'NONE', #7895 ) ;
#18539=CARTESIAN_POINT ( 'NONE',  ( -41.05189575270516400, 23.09451173561988213, 0.9172222222222163879 ) ) ;
#18542=DIRECTION ( 'NONE',  ( 0.9998501190848636533, 0.01731298258487451447, 5.158639060800524920E-16 ) ) ;
#18555=CIRCLE ( 'NONE', #34239, 0.6350000000000027844 ) ;
#18556=CARTESIAN_POINT ( 'NONE',  ( -58.43299954449013001, -0.3955325680177061431, 0.3375922266957475104 ) ) ;
#18562=AXIS2_PLACEMENT_3D ( 'NONE', #40235, #37031, #24011 ) ;
#18567=CARTESIAN_POINT ( 'NONE',  ( -57.72731561024293967, 0.8685078910841970146, -1.009486960136972124E-14 ) ) ;
#18574=CYLINDRICAL_SURFACE ( 'NONE', #7632, 0.2539999999999998925 ) ;
#18579=ORIENTED_EDGE ( 'NONE', *, *, #31551, .F. ) ;
#18580=CARTESIAN_POINT ( 'NONE',  ( -58.16194989728258946, 1.772972946764553193, -1.069098630790430628E-14 ) ) ;
#18582=CARTESIAN_POINT ( 'NONE',  ( -42.47169588413672159, 21.98427696618753302, -1.915014136677441581 ) ) ;
#18583=AXIS2_PLACEMENT_3D ( 'NONE', #34162, #33745, #7756 ) ;
#18590=CARTESIAN_POINT ( 'NONE',  ( -58.23230438342547188, 0.5587453749347339738, -1.096084957074963340 ) ) ;
#18595=CARTESIAN_POINT ( 'NONE',  ( -57.21666742898756297, 2.192505647111198552, -1.643075081891994138 ) ) ;
#18599=CARTESIAN_POINT ( 'NONE',  ( -56.80697847991661575, 4.636179106009441497, -2.484889565616585472 ) ) ;
#18601=ADVANCED_FACE ( 'NONE', ( #12336 ), #29313, .T. ) ;
#18607=CARTESIAN_POINT ( 'NONE',  ( -58.37241122568488549, -0.2962816677227753104, -0.2416009568454014489 ) ) ;
#18615=TOROIDAL_SURFACE ( 'NONE', #24065, 0.8889999999999989022, 0.2540000000000000036 ) ;
#18616=CARTESIAN_POINT ( 'NONE',  ( -41.05189575270522795, 23.09451173561975779, -1.171222222222227272 ) ) ;
#18619=CARTESIAN_POINT ( 'NONE',  ( -58.24807683554808335, 1.288543178753334573, 1.357556113208942428 ) ) ;
#18621=CIRCLE ( 'NONE', #37678, 0.2540000000000067204 ) ;
#18623=CARTESIAN_POINT ( 'NONE',  ( -50.58128808078254934, 18.64259194233895656, 3.042287330737921902 ) ) ;
#18626=CARTESIAN_POINT ( 'NONE',  ( -50.42190507837991476, 20.37545339363690999, -1.629190407695439324 ) ) ;
#18629=ORIENTED_EDGE ( 'NONE', *, *, #36018, .F. ) ;
#18632=AXIS2_PLACEMENT_3D ( 'NONE', #22148, #35180, #41994 ) ;
#18662=FACE_OUTER_BOUND ( 'NONE', #37979, .T. ) ;
#18666=CARTESIAN_POINT ( 'NONE',  ( -43.82859865241511699, 24.63416949198730421, -1.524000000000007127 ) ) ;
#18669=CARTESIAN_POINT ( 'NONE',  ( -57.98746369505321496, 0.5317391348542490626, 0.8755459602923044704 ) ) ;
#18673=ORIENTED_EDGE ( 'NONE', *, *, #2127, .T. ) ;
#18674=CARTESIAN_POINT ( 'NONE',  ( -58.70413935429054675, 0.2332485698458008905, 0.6626129746612759996 ) ) ;
#18680=ORIENTED_EDGE ( 'NONE', *, *, #10292, .T. ) ;
#18682=CARTESIAN_POINT ( 'NONE',  ( -30.03238267955204677, 57.98137616130296834, 1.269999999999994023 ) ) ;
#18683=CARTESIAN_POINT ( 'NONE',  ( -43.04734275525326126, 21.71211564561782481, 2.244749861970594118 ) ) ;
#18684=DIRECTION ( 'NONE',  ( -0.5149185422762211362, 0.8572391118119444542, 0.000000000000000000 ) ) ;
#18688=CARTESIAN_POINT ( 'NONE',  ( -6.135835944515187101, 77.40800365160224317, 1.524000000000003130 ) ) ;
#18696=CARTESIAN_POINT ( 'NONE',  ( -55.75614604655159923, 4.795084387130554404, 1.238208353029749853 ) ) ;
#18704=AXIS2_PLACEMENT_3D ( 'NONE', #15481, #34881, #15264 ) ;
#18705=VERTEX_POINT ( 'NONE', #24687 ) ;
#18712=CARTESIAN_POINT ( 'NONE',  ( -46.90713744787128547, 25.32984766614545080, 1.752173880707143860 ) ) ;
#18716=CARTESIAN_POINT ( 'NONE',  ( -44.66298991629287940, 23.47648082339880915, 1.964675176939932655 ) ) ;
#18720=ORIENTED_EDGE ( 'NONE', *, *, #2932, .T. ) ;
#18734=AXIS2_PLACEMENT_3D ( 'NONE', #27861, #24657, #40663 ) ;
#18738=ORIENTED_EDGE ( 'NONE', *, *, #17768, .F. ) ;
#18744=EDGE_CURVE ( 'NONE', #38897, #22759, #37695, .T. ) ;
#18755=DIRECTION ( 'NONE',  ( -0.8745520943968240202, 0.4849315768086553402, -5.361993529360572958E-16 ) ) ;
#18759=VERTEX_POINT ( 'NONE', #5333 ) ;
#18762=CARTESIAN_POINT ( 'NONE',  ( -21.32888081312384898, 55.91420173801096638, -1.270000000000000240 ) ) ;
#18765=VECTOR ( 'NONE', #3507, 1000.000000000000114 ) ;
#18777=DIRECTION ( 'NONE',  ( -0.7770581983690878491, 0.6294287539883980376, -5.101669463485847584E-16 ) ) ;
#18778=CARTESIAN_POINT ( 'NONE',  ( -17.14500000000466784, 71.11999999999886768, 1.269999999999998241 ) ) ;
#18785=ORIENTED_EDGE ( 'NONE', *, *, #42044, .T. ) ;
#18786=CARTESIAN_POINT ( 'NONE',  ( -58.83227707057486811, -0.08366279997995551554, -5.898546760656774196E-15 ) ) ;
#18788=CARTESIAN_POINT ( 'NONE',  ( -42.07367843439164545, 22.17357734922909529, -1.489526742666034576 ) ) ;
#18795=EDGE_CURVE ( 'NONE', #23884, #35416, #21801, .T. ) ;
#18796=CARTESIAN_POINT ( 'NONE',  ( -53.83932746694286919, 9.555192732579641302, -3.787265504858273513 ) ) ;
#18797=ORIENTED_EDGE ( 'NONE', *, *, #5598, .T. ) ;
#18805=CARTESIAN_POINT ( 'NONE',  ( -53.68435271313694557, 11.12367579685427721, -3.945100831076026715 ) ) ;
#18809=ORIENTED_EDGE ( 'NONE', *, *, #18744, .F. ) ;
#18814=CARTESIAN_POINT ( 'NONE',  ( -47.85244527695891037, 19.39403540832952544, -5.219971639306605127 ) ) ;
#18823=CARTESIAN_POINT ( 'NONE',  ( -20.37123700195716225, 79.57406833244878896, 1.269999999999995355 ) ) ;
#18824=EDGE_CURVE ( 'NONE', #2670, #3374, #18919, .T. ) ;
#18825=CIRCLE ( 'NONE', #20189, 0.2540000000000000036 ) ;
#18827=CARTESIAN_POINT ( 'NONE',  ( -45.52520984822221095, 18.49555408152312452, -0.5880787195337440210 ) ) ;
#18828=DIRECTION ( 'NONE',  ( -0.4849315768086535083, -0.8745520943968250194, -1.030032898892974695E-16 ) ) ;
#18829=CARTESIAN_POINT ( 'NONE',  ( -57.24023649071029496, 3.661034843983918208, 2.195083147259549339 ) ) ;
#18830=CARTESIAN_POINT ( 'NONE',  ( -56.41464036832825713, 4.421983009390323183, 2.556334463401503054 ) ) ;
#18831=FACE_OUTER_BOUND ( 'NONE', #8038, .T. ) ;
#18833=CARTESIAN_POINT ( 'NONE',  ( -29.82321757229076908, 71.17901112636586447, -1.270000000000007123 ) ) ;
#18834=CARTESIAN_POINT ( 'NONE',  ( -52.19327494808134560, 16.79818233314609444, 2.080405417473075946 ) ) ;
#18837=CARTESIAN_POINT ( 'NONE',  ( -50.25741847910705928, 21.95975045971864503, -0.7628348698132428884 ) ) ;
#18845=LINE ( 'NONE', #29280, #24733 ) ;
#18847=VECTOR ( 'NONE', #11353, 1000.000000000000227 ) ;
#18853=ORIENTED_EDGE ( 'NONE', *, *, #2446, .F. ) ;
#18857=AXIS2_PLACEMENT_3D ( 'NONE', #32511, #6525, #25490 ) ;
#18863=VECTOR ( 'NONE', #19212, 1000.000000000000000 ) ;
#18869=EDGE_CURVE ( 'NONE', #7108, #39553, #21138, .T. ) ;
#18870=VERTEX_POINT ( 'NONE', #14886 ) ;
#18874=AXIS2_PLACEMENT_3D ( 'NONE', #21148, #32975, #29970 ) ;
#18880=CARTESIAN_POINT ( 'NONE',  ( -58.36517903063335666, -0.2819031691279192398, 0.08479348624783289434 ) ) ;
#18892=ORIENTED_EDGE ( 'NONE', *, *, #1368, .F. ) ;
#18894=CARTESIAN_POINT ( 'NONE',  ( -31.80708539008069735, 53.04900798501882520, 1.523999999999994914 ) ) ;
#18896=CARTESIAN_POINT ( 'NONE',  ( -10.23480564747663379, 76.83082906289159553, 1.270000000000000906 ) ) ;
#18897=FACE_OUTER_BOUND ( 'NONE', #33462, .T. ) ;
#18908=ORIENTED_EDGE ( 'NONE', *, *, #32116, .T. ) ;
#18909=CARTESIAN_POINT ( 'NONE',  ( -56.42856387642239469, 3.193865871111076338, -9.870345732644628497E-15 ) ) ;
#18918=DIRECTION ( 'NONE',  ( 0.01731298258488073519, -0.9998501190848635423, 1.788962107505278613E-16 ) ) ;
#18919=LINE ( 'NONE', #21899, #30006 ) ;
#18922=EDGE_CURVE ( 'NONE', #26382, #26813, #25231, .T. ) ;
#18928=EDGE_CURVE ( 'NONE', #4992, #19512, #4885, .T. ) ;
#18929=CARTESIAN_POINT ( 'NONE',  ( -46.67659519887701691, 22.71018310752411651, 3.598098858967599512 ) ) ;
#18933=EDGE_LOOP ( 'NONE', ( #8716, #8564, #2144, #28723, #3352 ) ) ;
#18974=CARTESIAN_POINT ( 'NONE',  ( -24.24876516830975248, 76.58816925568820011, 1.269999999999993801 ) ) ;
#18975=VECTOR ( 'NONE', #3354, 1000.000000000000000 ) ;
#18977=FACE_OUTER_BOUND ( 'NONE', #8080, .T. ) ;
#18986=DIRECTION ( 'NONE',  ( 0.1906721105965039909, -0.9816537812491094028, 2.657572025465702696E-16 ) ) ;
#19000=CARTESIAN_POINT ( 'NONE',  ( -14.38915334913366983, 80.27078028363496287, 1.269999999999998019 ) ) ;
#19008=CARTESIAN_POINT ( 'NONE',  ( -56.05195996919411527, 5.170694913744002363, -2.763834368020857468 ) ) ;
#19010=CARTESIAN_POINT ( 'NONE',  ( -58.01460528358209956, 0.4727233027800176179, -0.8404818439587155021 ) ) ;
#19017=CARTESIAN_POINT ( 'NONE',  ( -49.01671973967521012, 18.67808020721676954, -5.174630477995056488 ) ) ;
#19023=CARTESIAN_POINT ( 'NONE',  ( -55.14069116334859189, 5.401725095812784261, -9.794129604158680367E-15 ) ) ;
#19025=AXIS2_PLACEMENT_3D ( 'NONE', #5597, #31558, #41373 ) ;
#19028=CYLINDRICAL_SURFACE ( 'NONE', #23982, 9.048749999999998295 ) ;
#19029=EDGE_CURVE ( 'NONE', #18166, #15388, #18439, .T. ) ;
#19032=CARTESIAN_POINT ( 'NONE',  ( -30.28638171898572651, 70.19821000523995735, -1.524000000000007571 ) ) ;
#19033=CARTESIAN_POINT ( 'NONE',  ( -47.11704014324647005, 20.18577099567724886, -5.127035723291441194 ) ) ;
#19036=CARTESIAN_POINT ( 'NONE',  ( -8.313969523394650452, 67.96940778435646280, 1.524000000000002908 ) ) ;
#19037=CARTESIAN_POINT ( 'NONE',  ( -51.06915940311598234, 14.53650747930048581, 4.673419795157606416 ) ) ;
#19040=CARTESIAN_POINT ( 'NONE',  ( -54.80060171144386771, 10.20856468236482684, 2.175828276708562825 ) ) ;
#19043=EDGE_LOOP ( 'NONE', ( #34089, #34401, #9856, #39993 ) ) ;
#19044=CARTESIAN_POINT ( 'NONE',  ( -52.80069327121181288, 17.37962920081948681, -0.7126778406583914593 ) ) ;
#19064=CARTESIAN_POINT ( 'NONE',  ( -58.31778746384443224, -0.1819811653371645743, -0.2882286546613240796 ) ) ;
#19071=EDGE_CURVE ( 'NONE', #37655, #2940, #35549, .T. ) ;
#19080=CARTESIAN_POINT ( 'NONE',  ( -42.34481381083929818, 23.19759442052183473, -1.554397948409621755 ) ) ;
#19081=EDGE_LOOP ( 'NONE', ( #35520, #28213, #37680, #25724, #27923 ) ) ;
#19085=CIRCLE ( 'NONE', #6180, 0.2539999999999997260 ) ;
#19086=DIRECTION ( 'NONE',  ( 0.7517731442105912709, -0.6594218222380281436, 8.537024980200781389E-16 ) ) ;
#19091=CARTESIAN_POINT ( 'NONE',  ( -4.345705637489792217, 70.43763872253876457, -1.523999999999994026 ) ) ;
#19092=CARTESIAN_POINT ( 'NONE',  ( -17.08598887363762131, 83.79821757228496892, -1.524000000000002908 ) ) ;
#19096=DIRECTION ( 'NONE',  ( -0.8745520943968251304, 0.4849315768086532863, -5.424246918827961050E-16 ) ) ;
#19098=CARTESIAN_POINT ( 'NONE',  ( -30.59449053042481736, 55.40488188693900895, 1.523999999999993582 ) ) ;
#19103=CARTESIAN_POINT ( 'NONE',  ( -29.20589784622301011, 64.40785669711239336, 1.523999999999849253 ) ) ;
#19107=DIRECTION ( 'NONE',  ( -5.188838149069471174E-16, 1.699382548006136313E-16, 1.000000000000000000 ) ) ;
#19120=ADVANCED_FACE ( 'NONE', ( #12949 ), #38949, .T. ) ;
#19122=CARTESIAN_POINT ( 'NONE',  ( -23.91048590848665611, 81.84235438443283783, -1.270000000000006235 ) ) ;
#19126=EDGE_LOOP ( 'NONE', ( #22993, #31122, #24416, #13839 ) ) ;
#19138=CARTESIAN_POINT ( 'NONE',  ( -52.51450000281151631, 11.69565325325087102, 4.043231167555472183 ) ) ;
#19139=CARTESIAN_POINT ( 'NONE',  ( -46.94769949131580233, 25.36820868695422604, 1.370102228390891685 ) ) ;
#19140=CARTESIAN_POINT ( 'NONE',  ( -41.05189575270519242, 23.09451173561980042, 1.269999999999989582 ) ) ;
#19141=CARTESIAN_POINT ( 'NONE',  ( -46.31144060707497090, 24.05480373873685451, 2.308638262703916588 ) ) ;
#19142=DIRECTION ( 'NONE',  ( 5.188838149069472160E-16, -1.699382548006136559E-16, -1.000000000000000000 ) ) ;
#19144=ORIENTED_EDGE ( 'NONE', *, *, #34150, .T. ) ;
#19163=ORIENTED_EDGE ( 'NONE', *, *, #33484, .F. ) ;
#19169=TOROIDAL_SURFACE ( 'NONE', #6944, 0.3809999999999999498, 0.2540000000000000036 ) ;
#19172=ORIENTED_EDGE ( 'NONE', *, *, #2814, .F. ) ;
#19173=CARTESIAN_POINT ( 'NONE',  ( -41.05189575270522795, 23.09451173561975779, 1.171222222222216613 ) ) ;
#19181=DIRECTION ( 'NONE',  ( -0.8745520943968235761, 0.4849315768086558398, -4.268512490100410909E-16 ) ) ;
#19187=FACE_OUTER_BOUND ( 'NONE', #24499, .T. ) ;
#19191=DIRECTION ( 'NONE',  ( -0.8745520943968243532, 0.4849315768086546741, -5.271987356194192020E-16 ) ) ;
#19207=DIRECTION ( 'NONE',  ( 0.8745520943968235761, -0.4849315768086558398, 4.268512490100410909E-16 ) ) ;
#19211=ORIENTED_EDGE ( 'NONE', *, *, #26871, .T. ) ;
#19212=DIRECTION ( 'NONE',  ( -5.188838149069471174E-16, 1.699382548006136313E-16, 1.000000000000000000 ) ) ;
#19214=CARTESIAN_POINT ( 'NONE',  ( -41.60680704300455801, 22.55277366187442212, -1.574601807768128303 ) ) ;
#19219=CARTESIAN_POINT ( 'NONE',  ( -57.50370530912426403, 2.128377494375849555, -1.812018770838218718 ) ) ;
#19221=CARTESIAN_POINT ( 'NONE',  ( -57.16742739522069883, 2.298121588034024221, -1.685181603006209450 ) ) ;
#19223=DIRECTION ( 'NONE',  ( 0.000000000000000000, 0.000000000000000000, 1.000000000000000000 ) ) ;
#19237=AXIS2_PLACEMENT_3D ( 'NONE', #5712, #25066, #15048 ) ;
#19238=CARTESIAN_POINT ( 'NONE',  ( -56.88731995051697510, 2.378615435641926013, -1.029510524999914353E-14 ) ) ;
#19239=VECTOR ( 'NONE', #39811, 1000.000000000000000 ) ;
#19242=PLANE ( 'NONE',  #15130 ) ;
#19245=CARTESIAN_POINT ( 'NONE',  ( -17.31476582418722643, 62.07284264934779827, 1.269999999999998908 ) ) ;
#19246=CARTESIAN_POINT ( 'NONE',  ( -48.77973395026506864, 17.81645205181620639, -4.684626272830477056 ) ) ;
#19248=DIRECTION ( 'NONE',  ( -5.188838149069472160E-16, 1.699382548006136559E-16, 1.000000000000000000 ) ) ;
#19249=CARTESIAN_POINT ( 'NONE',  ( -49.53393612610801711, 17.02900530345541696, 5.020798260677888258 ) ) ;
#19250=CARTESIAN_POINT ( 'NONE',  ( -24.24369025645185260, 82.02711331519694227, 1.523999999999992916 ) ) ;
#19251=CIRCLE ( 'NONE', #30814, 0.2540000000000038338 ) ;
#19254=CARTESIAN_POINT ( 'NONE',  ( -56.22979136716762838, 7.596919248368375399, 0.4408371032392935929 ) ) ;
#19257=ORIENTED_EDGE ( 'NONE', *, *, #11328, .T. ) ;
#19258=CARTESIAN_POINT ( 'NONE',  ( -53.73190450750161773, 11.39902669490613896, -3.613030284815582860 ) ) ;
#19265=CARTESIAN_POINT ( 'NONE',  ( -5.924740142096584172, 65.21691166894066782, -1.523999999999994026 ) ) ;
#19272=CARTESIAN_POINT ( 'NONE',  ( -36.65473259702432784, 28.27472347546385123, -1.524000000000003574 ) ) ;
#19276=ORIENTED_EDGE ( 'NONE', *, *, #13059, .F. ) ;
#19290=DIRECTION ( 'NONE',  ( -0.8745520943968235761, 0.4849315768086558398, -5.691349986800547879E-16 ) ) ;
#19291=CARTESIAN_POINT ( 'NONE',  ( -47.65206802627297833, 20.46304711373551299, -5.210715034831075343 ) ) ;
#19299=FACE_OUTER_BOUND ( 'NONE', #4743, .T. ) ;
#19301=DIRECTION ( 'NONE',  ( -0.3256999990547775337, -0.9454731675810359448, 0.000000000000000000 ) ) ;
#19304=ORIENTED_EDGE ( 'NONE', *, *, #35773, .T. ) ;
#19312=ORIENTED_EDGE ( 'NONE', *, *, #29504, .T. ) ;
#19316=CARTESIAN_POINT ( 'NONE',  ( -4.345705637489792217, 70.43763872253877878, 1.270000000000005125 ) ) ;
#19319=( BOUNDED_SURFACE ( )  B_SPLINE_SURFACE ( 2, 3, ( 
 ( #36917, #7942, #26692, #23682, #935, #1139, #11125, #29885, #13905, #16670, #7524, #36702, #24112, #26478, #26895, #20701, #30507, #14305, #1348, #7735, #39482, #13492, #20485, #37120, #33726, #10288, #14106, #17509, #17308, #13698, #27317, #29676, #16884, #23258, #3712, #30296, #40331, #36292, #7112, #23900, #40117, #20071, #17091, #23468, #10910, #39909, #33093, #33512, #519, #10703 ),
 ( #7315, #39699, #4550, #10498, #20274, #4132, #30094, #4762, #11965, #40537, #11333, #21321, #34140, #34349, #8142, #24321, #30713, #18133, #8567, #21529, #15149, #21114, #4967, #1564, #1768, #17714, #24958, #2403, #14939, #31138, #17925, #11754, #1977, #18556, #40742, #20911, #37959, #25175, #24742, #14521, #27531, #15362, #27941, #30930, #14729, #5180, #40948, #37744, #34561, #28369 ),
 ( #38176, #27731, #5388, #18343, #31349, #41376, #11539, #2192, #37327, #28154, #41160, #12182, #24522, #8784, #21742, #31561, #33933, #37528, #34768, #8353, #5601, #12798, #29413, #13006, #28580, #19394, #35817, #22575, #31983, #19600, #5808, #22157, #31774, #253, #35606, #6633, #2615, #15575, #40, #32400, #41588, #12598, #25999, #26213, #39008, #13230, #2821, #9818, #22784, #8990 ) ),
 .UNSPECIFIED., .F., .F., .T. ) 
 B_SPLINE_SURFACE_WITH_KNOTS ( ( 3, 3 ),
 ( 4, 2, 2, 2, 2, 2, 2, 2, 2, 2, 2, 2, 2, 2, 2, 2, 2, 2, 2, 2, 2, 2, 2, 2, 4 ),
 ( 0.000000000000000000, 1.000000000000000000 ),
 ( 0.000000000000000000, 0.001458241944942368154, 0.002916483889884736308, 0.005832967779769472616, 0.01166593555953894523, 0.01458241944942368154, 0.01749890333930841785, 0.01895714528425078427, 0.02041538722919315416, 0.02114450820166433737, 0.02150906868789993071, 0.02187362917413552404, 0.02223818966037111738, 0.02260275014660670725, 0.02296731063284229712, 0.02305845075440119546, 0.02310402081518064463, 0.02312680584557037095, 0.02313250210316779992, 0.02313819836076523237, 0.02314959087596009379, 0.02319516093673954296, 0.02324073099751899213, 0.02328630105829844130, 0.02333187111907789046 ),
 .UNSPECIFIED. ) 
 GEOMETRIC_REPRESENTATION_ITEM ( )  RATIONAL_B_SPLINE_SURFACE ( (
 ( 1.000000000000000000, 1.000000000000000000, 1.000000000000000000, 1.000000000000000000, 1.000000000000000000, 1.000000000000000000, 1.000000000000000000, 1.000000000000000000, 1.000000000000000000, 1.000000000000000000, 1.000000000000000000, 1.000000000000000000, 1.000000000000000000, 1.000000000000000000, 1.000000000000000000, 1.000000000000000000, 1.000000000000000000, 1.000000000000000000, 1.000000000000000000, 1.000000000000000000, 1.000000000000000000, 1.000000000000000000, 1.000000000000000000, 1.000000000000000000, 1.000000000000000000, 1.000000000000000000, 1.000000000000000000, 1.000000000000000000, 1.000000000000000000, 1.000000000000000000, 1.000000000000000000, 1.000000000000000000, 1.000000000000000000, 1.000000000000000000, 1.000000000000000000, 1.000000000000000000, 1.000000000000000000, 1.000000000000000000, 1.000000000000000000, 1.000000000000000000, 1.000000000000000000, 1.000000000000000000, 1.000000000000000000, 1.000000000000000000, 1.000000000000000000, 1.000000000000000000, 1.000000000000000000, 1.000000000000000000, 1.000000000000000000, 1.000000000000000000),
 ( 0.9987193938133573923, 0.9996013059079669194, 0.9991963860900630046, 0.9949866313569200038, 0.9909603791773133885, 0.9774858857087078690, 0.9654485462739429424, 0.9208787474569170017, 0.8807605768912754041, 0.8373543814104991156, 0.8249666374385254963, 0.8044008243459336294, 0.7962249832271174332, 0.7861950991335926453, 0.7832680976431367625, 0.7777782220875287811, 0.7752303374714799578, 0.7716286403903510616, 0.7703172242827316385, 0.7685261186011436152, 0.7673635575496201566, 0.7657163664523159996, 0.7656514573011637959, 0.7645255059892569482, 0.7630494482540092216, 0.7607147317280203991, 0.7600215756489282493, 0.7585094466894809484, 0.7575231611504058549, 0.7546848085681980844, 0.7541407386780549782, 0.7516848864288520060, 0.7509064819841395622, 0.7462986158548496896, 0.7479156148892531775, 0.7339777749611771096, 0.7233604987256092578, 0.7138238211873346728, 0.7102391262371019476, 0.6994720207875538831, 0.6929862625710326851, 0.6601362149681273550, 0.6323867238837976856, 0.5714353381031282986, 0.5388352690740847439, 0.4817946329374578895, 0.4578268140822101540, 0.4260966422725533942, 0.4180307774937941923, 0.4190531958282215919),
 ( 1.000000000000000000, 1.000000000000000000, 1.000000000000000000, 1.000000000000000000, 1.000000000000000000, 1.000000000000000000, 1.000000000000000000, 1.000000000000000000, 1.000000000000000000, 1.000000000000000000, 1.000000000000000000, 1.000000000000000000, 1.000000000000000000, 1.000000000000000000, 1.000000000000000000, 1.000000000000000000, 1.000000000000000000, 1.000000000000000000, 1.000000000000000000, 1.000000000000000000, 1.000000000000000000, 1.000000000000000000, 1.000000000000000000, 1.000000000000000000, 1.000000000000000000, 1.000000000000000000, 1.000000000000000000, 1.000000000000000000, 1.000000000000000000, 1.000000000000000000, 1.000000000000000000, 1.000000000000000000, 1.000000000000000000, 1.000000000000000000, 1.000000000000000000, 1.000000000000000000, 1.000000000000000000, 1.000000000000000000, 1.000000000000000000, 1.000000000000000000, 1.000000000000000000, 1.000000000000000000, 1.000000000000000000, 1.000000000000000000, 1.000000000000000000, 1.000000000000000000, 1.000000000000000000, 1.000000000000000000, 1.000000000000000000, 1.000000000000000000) ) ) 
 REPRESENTATION_ITEM ( '' )  SURFACE ( )  );
#19327=EDGE_LOOP ( 'NONE', ( #26474, #1762, #7822, #34706 ) ) ;
#19331=ADVANCED_FACE ( 'NONE', ( #14207 ), #33620, .F. ) ;
#19339=EDGE_CURVE ( 'NONE', #15671, #2842, #17150, .T. ) ;
#19341=CARTESIAN_POINT ( 'NONE',  ( -48.82359235824656452, 18.05626978637514313, 5.103416509772343623 ) ) ;
#19342=CARTESIAN_POINT ( 'NONE',  ( -46.95726096424718321, 25.94444535518948669, 0.08936005021614831789 ) ) ;
#19344=VERTEX_POINT ( 'NONE', #1037 ) ;
#19345=CARTESIAN_POINT ( 'NONE',  ( -44.55074271434504851, 21.27721161058206789, 3.389857510897057224 ) ) ;
#19349=VERTEX_POINT ( 'NONE', #4027 ) ;
#19350=ORIENTED_EDGE ( 'NONE', *, *, #8135, .F. ) ;
#19356=CARTESIAN_POINT ( 'NONE',  ( -58.83227707057486811, -0.08366279997995551554, -1.529465441686574059E-14 ) ) ;
#19369=CARTESIAN_POINT ( 'NONE',  ( -19.64403260974359355, 72.50569198072959409, -1.524000000000002242 ) ) ;
#19375=EDGE_LOOP ( 'NONE', ( #37165, #40522, #27086, #21784 ) ) ;
#19377=CARTESIAN_POINT ( 'NONE',  ( -43.98989719630797168, 21.38545485255711398, 2.905481552205958717 ) ) ;
#19381=CIRCLE ( 'NONE', #3783, 0.2540000000000012248 ) ;
#19390=VERTEX_POINT ( 'NONE', #13591 ) ;
#19391=DIRECTION ( 'NONE',  ( -0.8745520943968235761, 0.4849315768086558398, -4.268512490100410909E-16 ) ) ;
#19392=DIRECTION ( 'NONE',  ( 5.188838149069472160E-16, -1.699382548006136559E-16, -1.000000000000000000 ) ) ;
#19393=EDGE_CURVE ( 'NONE', #2940, #23452, #17198, .T. ) ;
#19394=CARTESIAN_POINT ( 'NONE',  ( -58.36601048454566154, 0.2708230323985594268, 0.9148880203688037893 ) ) ;
#19395=EDGE_CURVE ( 'NONE', #3974, #34427, #35413, .T. ) ;
#19414=CARTESIAN_POINT ( 'NONE',  ( -47.00787117332040310, 24.49876931072293829, -2.333946431867834015 ) ) ;
#19415=PLANE ( 'NONE',  #12402 ) ;
#19427=CARTESIAN_POINT ( 'NONE',  ( -58.01740762695335718, 1.024996124235854955, -1.342718164770963840 ) ) ;
#19428=ORIENTED_EDGE ( 'NONE', *, *, #28421, .F. ) ;
#19429=CARTESIAN_POINT ( 'NONE',  ( -51.89660998226970889, 12.88425699701367577, -4.274492870977415038 ) ) ;
#19437=CARTESIAN_POINT ( 'NONE',  ( -57.00508801794419611, 2.691366720778187727, -1.977812201481553567 ) ) ;
#19442=ORIENTED_EDGE ( 'NONE', *, *, #27160, .T. ) ;
#19445=FACE_OUTER_BOUND ( 'NONE', #41399, .T. ) ;
#19453=CARTESIAN_POINT ( 'NONE',  ( -46.25688858429103334, 20.73875112231585760, -4.700046123029353318 ) ) ;
#19458=FACE_OUTER_BOUND ( 'NONE', #1849, .T. ) ;
#19460=CARTESIAN_POINT ( 'NONE',  ( -55.52324119379100864, 8.418761648454426094, 1.955819887484142372 ) ) ;
#19462=CARTESIAN_POINT ( 'NONE',  ( -57.07867440696631434, 2.606095844753547830, 1.988717289889800677 ) ) ;
#19464=CIRCLE ( 'NONE', #8599, 0.6350000000000014522 ) ;
#19465=ORIENTED_EDGE ( 'NONE', *, *, #18922, .F. ) ;
#19466=CARTESIAN_POINT ( 'NONE',  ( -50.45326722236683281, 19.63324548489221044, -2.269669894115913689 ) ) ;
#19467=CIRCLE ( 'NONE', #24916, 0.3809999999999984510 ) ;
#19477=CARTESIAN_POINT ( 'NONE',  ( -8.438477507926629428, 69.62414081991882142, 1.524000000000003130 ) ) ;
#19480=CARTESIAN_POINT ( 'NONE',  ( -28.42835727709238114, 77.69497285144578314, 1.269999999999991358 ) ) ;
#19481=EDGE_LOOP ( 'NONE', ( #13268, #14499, #5129, #36881 ) ) ;
#19484=CARTESIAN_POINT ( 'NONE',  ( -58.35647611463063100, -0.2636741081728710134, -0.1439816294147371889 ) ) ;
#19496=LINE ( 'NONE', #3124, #38075 ) ;
#19497=CARTESIAN_POINT ( 'NONE',  ( -46.20552558087364758, 24.41938074005533466, -2.020549794458512682 ) ) ;
#19498=VECTOR ( 'NONE', #7531, 1000.000000000000227 ) ;
#19499=EDGE_LOOP ( 'NONE', ( #32150, #28490, #7042, #26234 ) ) ;
#19507=DIRECTION ( 'NONE',  ( -0.8745520943968249084, 0.4849315768086536194, -5.575199987069925217E-16 ) ) ;
#19508=DIRECTION ( 'NONE',  ( 0.9454731675810332803, -0.3256999990547855828, 8.537024980200802097E-16 ) ) ;
#19512=VERTEX_POINT ( 'NONE', #11431 ) ;
#19525=AXIS2_PLACEMENT_3D ( 'NONE', #13021, #12815, #12612 ) ;
#19529=DIRECTION ( 'NONE',  ( -0.8745520943968235761, 0.4849315768086558398, -4.268512490100410909E-16 ) ) ;
#19537=DIRECTION ( 'NONE',  ( -0.01731298258488073519, 0.9998501190848635423, -1.788962107505278613E-16 ) ) ;
#19538=AXIS2_PLACEMENT_3D ( 'NONE', #10163, #32756, #810 ) ;
#19539=ORIENTED_EDGE ( 'NONE', *, *, #34244, .T. ) ;
#19545=CARTESIAN_POINT ( 'NONE',  ( -46.72105977771763463, 25.94162485481863456, 1.365922269189760563 ) ) ;
#19546=CARTESIAN_POINT ( 'NONE',  ( -46.93527007713159804, 25.91000514300129254, 0.2210822239326031835 ) ) ;
#19548=CARTESIAN_POINT ( 'NONE',  ( -44.36446822842629700, 21.81554158013422651, 2.896954608336737014 ) ) ;
#19552=CARTESIAN_POINT ( 'NONE',  ( -58.31320831016853390, -0.1895118959954616988, -0.07592354283883193111 ) ) ;
#19562=( GEOMETRIC_REPRESENTATION_CONTEXT ( 3 ) GLOBAL_UNCERTAINTY_ASSIGNED_CONTEXT ( ( #32100 ) ) GLOBAL_UNIT_ASSIGNED_CONTEXT ( ( #40319, #11317, #33713 ) ) REPRESENTATION_CONTEXT ( 'NONE', 'WORKASPACE' ) );
#19564=CARTESIAN_POINT ( 'NONE',  ( -23.21760062652228385, 78.26400813401573942, 1.269999999999993801 ) ) ;
#19565=DIRECTION ( 'NONE',  ( 0.9816537812491090698, 0.1906721105965065721, 4.769617732184476148E-16 ) ) ;
#19583=CARTESIAN_POINT ( 'NONE',  ( -47.34044527953909665, 17.31523404052589399, 1.593293138114921792 ) ) ;
#19590=CARTESIAN_POINT ( 'NONE',  ( -6.194847070882102180, 64.72978607931611350, 1.270000000000006013 ) ) ;
#19595=ORIENTED_EDGE ( 'NONE', *, *, #35747, .T. ) ;
#19597=ADVANCED_FACE ( 'NONE', ( #1667 ), #41479, .F. ) ;
#19600=CARTESIAN_POINT ( 'NONE',  ( -58.59897934080984783, -0.2308949485120836975, 0.4634499375557190048 ) ) ;
#19613=CARTESIAN_POINT ( 'NONE',  ( -11.53797084252497207, 82.58007221317646440, -1.269999999999999796 ) ) ;
#19616=CARTESIAN_POINT ( 'NONE',  ( -46.95911617132933458, 24.98948415085536823, -1.986615011824472088 ) ) ;
#19621=EDGE_LOOP ( 'NONE', ( #408, #28008, #39738, #2399, #2844 ) ) ;
#19629=CARTESIAN_POINT ( 'NONE',  ( -58.52079444616499870, -0.06495539389881313519, -0.6452041206688503561 ) ) ;
#19631=ORIENTED_EDGE ( 'NONE', *, *, #5496, .T. ) ;
#19639=CIRCLE ( 'NONE', #20302, 0.5080000000000010063 ) ;
#19641=CARTESIAN_POINT ( 'NONE',  ( -58.73801720703743001, -0.4998429216807459552, -0.2437502737749605297 ) ) ;
#19642=ORIENTED_EDGE ( 'NONE', *, *, #2183, .T. ) ;
#19649=EDGE_CURVE ( 'NONE', #17215, #26023, #40247, .T. ) ;
#19650=CARTESIAN_POINT ( 'NONE',  ( -41.41491986784954804, 22.70581808553406233, -6.121743196690467558E-15 ) ) ;
#19657=AXIS2_PLACEMENT_3D ( 'NONE', #25555, #31530, #21927 ) ;
#19658=CARTESIAN_POINT ( 'NONE',  ( -45.58494389689084869, 18.10922195552001313, -7.361215080689235889E-15 ) ) ;
#19659=VERTEX_POINT ( 'NONE', #34871 ) ;
#19663=CARTESIAN_POINT ( 'NONE',  ( -46.75016890987451035, 25.87258681965687757, -1.401816643053204414 ) ) ;
#19664=CARTESIAN_POINT ( 'NONE',  ( -36.98328822617348521, 27.82293856516311692, 1.523999999999995580 ) ) ;
#19665=FACE_OUTER_BOUND ( 'NONE', #2343, .T. ) ;
#19668=DIRECTION ( 'NONE',  ( 0.6825627711659328911, 0.7308269722843309113, 2.299753143848213649E-16 ) ) ;
#19669=CARTESIAN_POINT ( 'NONE',  ( -54.68578128245503223, 13.03233524004687638, -1.048863621890573067E-14 ) ) ;
#19670=CARTESIAN_POINT ( 'NONE',  ( -57.50953982388014651, 1.662011999372992044, 1.631050346940570384 ) ) ;
#19672=ORIENTED_EDGE ( 'NONE', *, *, #8114, .T. ) ;
#19673=CARTESIAN_POINT ( 'NONE',  ( -50.58128808078254934, 18.64259194233895656, -3.042287330737940110 ) ) ;
#19675=EDGE_LOOP ( 'NONE', ( #3438, #12530, #20853, #7964 ) ) ;
#19686=CARTESIAN_POINT ( 'NONE',  ( -48.10788822079490501, 19.08060971762839486, -5.220410434069243877 ) ) ;
#19691=CARTESIAN_POINT ( 'NONE',  ( -58.37015987205347045, -0.2922188715788874291, -0.003179148003318876120 ) ) ;
#19698=AXIS2_PLACEMENT_3D ( 'NONE', #7369, #20538, #39965 ) ;
#19703=ADVANCED_FACE ( 'NONE', ( #18662 ), #36171, .T. ) ;
#19708=CARTESIAN_POINT ( 'NONE',  ( -48.59875010875282442, 18.41211343146811785, -5.165832069028398088 ) ) ;
#19709=ORIENTED_EDGE ( 'NONE', *, *, #13629, .T. ) ;
#19716=CYLINDRICAL_SURFACE ( 'NONE', #12442, 9.048749999999998295 ) ;
#19720=ORIENTED_EDGE ( 'NONE', *, *, #27160, .F. ) ;
#19734=CARTESIAN_POINT ( 'NONE',  ( -48.99983924688925185, 17.84334367881515604, -5.121602422839403701 ) ) ;
#19735=FACE_OUTER_BOUND ( 'NONE', #5743, .T. ) ;
#19740=VERTEX_POINT ( 'NONE', #41904 ) ;
#19744=TOROIDAL_SURFACE ( 'NONE', #44, 0.3809999999999993947, 0.2540000000000000036 ) ;
#19745=DIRECTION ( 'NONE',  ( 5.188838149069472160E-16, -1.699382548006136559E-16, -1.000000000000000000 ) ) ;
#19756=CARTESIAN_POINT ( 'NONE',  ( -47.16890147375944764, 22.20336809214633433, 4.187060126831872786 ) ) ;
#19759=CARTESIAN_POINT ( 'NONE',  ( -54.47970570282438274, 8.083255770631444292, 3.476097746275891076 ) ) ;
#19762=CARTESIAN_POINT ( 'NONE',  ( -58.37241122568489970, -0.2962816677228030660, -1.024972700666444124E-14 ) ) ;
#19763=B_SPLINE_SURFACE_WITH_KNOTS ( 'NONE', 3, 3, ( 
 ( #28769, #41781, #19173, #18539, #32179, #15346, #25157, #12784, #38158 ),
 ( #3011, #15970, #5372, #7254, #3856, #38993, #6823, #35801, #6408 ),
 ( #20010, #33240, #23405, #29179, #22769, #6615, #3427, #39845, #7043 ),
 ( #16392, #29398, #33027, #13214, #26838, #237, #20214, #19792, #26196 ),
 ( #19377, #17028, #867, #4069, #16176, #32383, #13630, #32812, #39201 ),
 ( #36009, #10009, #22982, #26620, #661, #36435, #26, #23187, #3643 ),
 ( #16607, #29615, #36222, #451, #32593, #12990, #13422, #26410, #25985 ),
 ( #39415, #13840, #10217, #30027, #16821, #19583, #22561, #10434, #29823 ),
 ( #39629, #35591, #3214, #9802, #1708, #40678, #23834, #34288, #30444 ),
 ( #21054, #27047, #8288, #30235, #36641, #20843, #1498, #33868, #24254 ),
 ( #40055, #40269, #4698, #17862, #34080, #17652, #11065, #1074, #30862 ),
 ( #30654, #20632, #14043, #17445, #24048, #10848, #33449, #14246, #1911 ),
 ( #11470, #37063, #7673, #21258, #24459, #7880, #1288, #27253, #36855 ),
 ( #14455, #14662, #37464, #33660, #5116, #27467, #40477, #4907, #4485 ),
 ( #11269, #7463, #37262, #8081, #27667, #18069, #31071, #14873, #27875 ),
 ( #10641, #23621, #20422, #4278, #17240, #12324, #31706, #21885, #25312 ),
 ( #11686, #34491, #41726, #38317, #8920, #5527, #34913, #9136, #8712 ),
 ( #28510, #41518, #12531, #21674, #18696, #5744, #31490, #12111, #41094 ),
 ( #37681, #15082, #2755, #8503, #11901, #18484, #2548, #40884, #18909 ),
 ( #28083, #41306, #24890, #21460, #37887, #22095, #15712, #35122, #18275 ),
 ( #34698, #2335, #24672, #5949, #15509, #15294, #28299, #31920, #25101 ),
 ( #28715, #5322, #31276, #38104, #2119, #37182, #23965, #14170, #27586 ),
 ( #17989, #28001, #30986, #36984, #7803, #4414, #14791, #2037, #37387 ),
 ( #30776, #33996, #20765, #40595, #10982, #37594, #4826, #14581, #5238 ),
 ( #20552, #33790, #34204, #18193, #8420, #1211, #4618, #17573, #30577 ),
 ( #21176, #20975, #1416, #14372, #5031, #27383, #41010, #40393, #21378 ),
 ( #11187, #34404, #33581, #31194, #15002, #11818, #30362, #17371, #27794 ),
 ( #24171, #27174, #8004, #17778, #1626, #40802, #11603, #36773, #40187 ),
 ( #11395, #24381, #8204, #1827, #24587, #7590, #34831, #15216, #31627 ) ),
 .UNSPECIFIED., .F., .F., .F.,
 ( 4, 1, 1, 1, 1, 1, 1, 2, 1, 1, 1, 1, 1, 1, 1, 1, 1, 1, 1, 1, 1, 1, 1, 1, 1, 4 ),
 ( 4, 1, 1, 1, 1, 1, 4 ),
 ( 0.000000000000000000, 0.03307066603948304734, 0.06614133207896609468, 0.09921199811844919059, 0.1653533301974152714, 0.1984239962368983812, 0.2314946622763813522, 0.2645653283158643787, 0.3105299952961229071, 0.3564946622763812689, 0.4024593292566397418, 0.4484239962368982702, 0.5403533301974150493, 0.6322826641579321061, 0.7242119981184491628, 0.7701766650987074136, 0.8161413320789658865, 0.8850883325493537068, 0.8965794992944182695, 0.9080706660394826102, 0.9195618327845473949, 0.9310529995296121797, 0.9425441662746769644, 0.9540353330197415271, 0.9770176665098706525, 1.000000000000000000 ),
 ( 0.000000000000000000, 0.2500000000000000000, 0.4444444444444445308, 0.5000000000000000000, 0.7500000000000000000, 0.8333333333333333703, 1.000000000000000000 ),
 .UNSPECIFIED. ) ;
#19769=AXIS2_PLACEMENT_3D ( 'NONE', #40895, #15307, #2766 ) ;
#19771=CARTESIAN_POINT ( 'NONE',  ( -46.67763236942723637, 26.04755295256607539, -0.6632588273528947642 ) ) ;
#19773=DIRECTION ( 'NONE',  ( -6.829619984160660610E-15, 0.000000000000000000, -1.000000000000000000 ) ) ;
#19774=DIRECTION ( 'NONE',  ( -0.8745520943968241312, 0.4849315768086548406, -5.691349986800536046E-16 ) ) ;
#19790=ORIENTED_EDGE ( 'NONE', *, *, #25853, .T. ) ;
#19792=CARTESIAN_POINT ( 'NONE',  ( -43.13073682054399427, 20.84535665847942454, 0.1327613832363976898 ) ) ;
#19799=DIRECTION ( 'NONE',  ( 0.000000000000000000, 0.000000000000000000, 1.000000000000000000 ) ) ;
#19806=CARTESIAN_POINT ( 'NONE',  ( -6.135835944515187101, 77.40800365160224317, -1.523999999999996247 ) ) ;
#19808=AXIS2_PLACEMENT_3D ( 'NONE', #28680, #6743, #10135 ) ;
#19811=EDGE_CURVE ( 'NONE', #37552, #15033, #3562, .T. ) ;
#19814=AXIS2_PLACEMENT_3D ( 'NONE', #26495, #8891, #25071 ) ;
#19816=DIRECTION ( 'NONE',  ( -5.188838149069471174E-16, 1.699382548006136313E-16, 1.000000000000000000 ) ) ;
#19823=CARTESIAN_POINT ( 'NONE',  ( -27.88833342972739615, 78.11058938209563962, -1.524000000000007571 ) ) ;
#19825=FACE_OUTER_BOUND ( 'NONE', #39004, .T. ) ;
#19827=VECTOR ( 'NONE', #26496, 1000.000000000000227 ) ;
#19832=EDGE_CURVE ( 'NONE', #22759, #30779, #38201, .T. ) ;
#19834=CIRCLE ( 'NONE', #3551, 0.2539999999999998925 ) ;
#19836=CYLINDRICAL_SURFACE ( 'NONE', #10826, 0.2539999999999967839 ) ;
#19837=VERTEX_POINT ( 'NONE', #23107 ) ;
#19838=LINE ( 'NONE', #32426, #27059 ) ;
#19839=VERTEX_POINT ( 'NONE', #6120 ) ;
#19840=LINE ( 'NONE', #16219, #2253 ) ;
#19846=CARTESIAN_POINT ( 'NONE',  ( -58.64513978733522492, -0.3133698122888631810, -0.3358519082774775733 ) ) ;
#19847=ORIENTED_EDGE ( 'NONE', *, *, #42058, .F. ) ;
#19855=CARTESIAN_POINT ( 'NONE',  ( -58.24002838079472610, 0.001074765447070524793, -0.6562585879479864159 ) ) ;
#19859=ORIENTED_EDGE ( 'NONE', *, *, #852, .F. ) ;
#19873=EDGE_CURVE ( 'NONE', #10519, #34270, #17769, .T. ) ;
#19874=CARTESIAN_POINT ( 'NONE',  ( -51.26804087848103819, 14.04722136430348201, -4.535752393750718703 ) ) ;
#19877=CARTESIAN_POINT ( 'NONE',  ( -46.63124922200988465, 26.12666050884489977, -1.285908859455852316 ) ) ;
#19878=CARTESIAN_POINT ( 'NONE',  ( -29.16381924947294024, 66.91553870234344004, -1.270000000000006013 ) ) ;
#19882=DIRECTION ( 'NONE',  ( 0.2290273297124658103, -0.9734199927291290466, 2.580167833703409551E-15 ) ) ;
#19883=CARTESIAN_POINT ( 'NONE',  ( -57.38748718130355542, 3.645894598607590797, 1.236217348619458090 ) ) ;
#19884=CARTESIAN_POINT ( 'NONE',  ( -57.36719850051837000, 1.975114663830185302, 1.756955940785651871 ) ) ;
#19887=CARTESIAN_POINT ( 'NONE',  ( -52.19327494808134560, 16.79818233314609444, -2.080405417473095930 ) ) ;
#19889=EDGE_CURVE ( 'NONE', #16174, #30132, #26637, .T. ) ;
#19890=ORIENTED_EDGE ( 'NONE', *, *, #34191, .F. ) ;
#19891=CARTESIAN_POINT ( 'NONE',  ( -17.14500000000466784, 71.11999999999886768, 1.523999999999998689 ) ) ;
#19897=EDGE_CURVE ( 'NONE', #17342, #34427, #38698, .T. ) ;
#19906=ORIENTED_EDGE ( 'NONE', *, *, #14373, .T. ) ;
#19908=CARTESIAN_POINT ( 'NONE',  ( -57.92645925829798159, 0.6640176851100348943, -0.9534638877764777254 ) ) ;
#19915=VECTOR ( 'NONE', #23796, 1000.000000000000000 ) ;
#19921=CARTESIAN_POINT ( 'NONE',  ( -10.18297664959815663, 77.66688486464208552, 1.524000000000001354 ) ) ;
#19923=CARTESIAN_POINT ( 'NONE',  ( -47.35944255389382107, 21.37623662739424191, -4.722871667523179440 ) ) ;
#19927=CIRCLE ( 'NONE', #28100, 0.2539999999999966729 ) ;
#19929=VECTOR ( 'NONE', #23396, 1000.000000000000000 ) ;
#19933=EDGE_CURVE ( 'NONE', #40718, #30484, #42114, .T. ) ;
#19935=CYLINDRICAL_SURFACE ( 'NONE', #28764, 0.6350000000000014522 ) ;
#19936=CARTESIAN_POINT ( 'NONE',  ( -58.36937220204561072, -0.2906615202371656270, 0.02563298686227328746 ) ) ;
#19937=CIRCLE ( 'NONE', #4972, 0.3809999999999977849 ) ;
#19945=CARTESIAN_POINT ( 'NONE',  ( -41.26650596300343921, 23.23696532716408925, 1.523999999999985366 ) ) ;
#19947=EDGE_CURVE ( 'NONE', #21011, #15945, #21662, .T. ) ;
#19958=AXIS2_PLACEMENT_3D ( 'NONE', #16802, #25755, #19773 ) ;
#19961=VERTEX_POINT ( 'NONE', #32089 ) ;
#19966=DIRECTION ( 'NONE',  ( 0.9454731675810359448, -0.3256999990547780333, 5.459396135145339171E-16 ) ) ;
#19967=AXIS2_PLACEMENT_3D ( 'NONE', #5295, #8892, #34885 ) ;
#19972=CIRCLE ( 'NONE', #9104, 0.2539999999999991709 ) ;
#19978=AXIS2_PLACEMENT_3D ( 'NONE', #9279, #22237, #35265 ) ;
#19979=CARTESIAN_POINT ( 'NONE',  ( -46.72764730961441160, 25.92641697299453440, 1.373594020054483167 ) ) ;
#19980=CARTESIAN_POINT ( 'NONE',  ( -48.34142060212426628, 20.97662605846759831, 3.847193496378342736 ) ) ;
#19982=CARTESIAN_POINT ( 'NONE',  ( -54.77668461537430034, 8.146287316968315650, 3.518595155146524434 ) ) ;
#19983=CARTESIAN_POINT ( 'NONE',  ( -58.69929992858412504, -0.3146504455105202935, 0.2902061446857141513 ) ) ;
#19987=CARTESIAN_POINT ( 'NONE',  ( -43.87210973174860129, 22.05421410453335795, 2.454571855453426377 ) ) ;
#19992=CIRCLE ( 'NONE', #25451, 0.8889999999999984581 ) ;
#20004=CIRCLE ( 'NONE', #25462, 0.3810000000000015041 ) ;
#20010=CARTESIAN_POINT ( 'NONE',  ( -41.87797633265722652, 22.30863410810708558, 1.617563149257729815 ) ) ;
#20015=CIRCLE ( 'NONE', #8447, 0.2540000000000023350 ) ;
#20021=EDGE_LOOP ( 'NONE', ( #35424, #15424, #9736, #12734 ) ) ;
#20024=DIRECTION ( 'NONE',  ( 5.188838149069472160E-16, -1.699382548006136559E-16, -1.000000000000000000 ) ) ;
#20025=CARTESIAN_POINT ( 'NONE',  ( -23.16987411132078734, 77.52691185402750307, 1.523999999999994470 ) ) ;
#20043=EDGE_CURVE ( 'NONE', #25505, #18759, #9507, .T. ) ;
#20047=ORIENTED_EDGE ( 'NONE', *, *, #3768, .F. ) ;
#20048=CARTESIAN_POINT ( 'NONE',  ( -11.43668055974971587, 78.14103736854400495, -1.523999999999999133 ) ) ;
#20049=EDGE_LOOP ( 'NONE', ( #28692, #20637, #29346, #26461 ) ) ;
#20055=CARTESIAN_POINT ( 'NONE',  ( -58.68693696493448186, -0.3142683078187059609, -0.3029362029564767189 ) ) ;
#20056=VERTEX_POINT ( 'NONE', #6526 ) ;
#20057=CARTESIAN_POINT ( 'NONE',  ( -58.36720124622751626, -0.2861505079054943446, -0.06388190288962447561 ) ) ;
#20060=CARTESIAN_POINT ( 'NONE',  ( -28.36525985791271154, 77.02308833105713859, 1.523999999999992028 ) ) ;
#20063=CARTESIAN_POINT ( 'NONE',  ( -58.40597088826705630, 0.2738206778524349128, -0.9753506901443967925 ) ) ;
#20071=CARTESIAN_POINT ( 'NONE',  ( -58.35171525856283381, -0.2536858515840151318, 0.1680674994488967344 ) ) ;
#20078=CARTESIAN_POINT ( 'NONE',  ( -54.82379132704179625, 7.242239488055856711, -3.238872252923487682 ) ) ;
#20081=CARTESIAN_POINT ( 'NONE',  ( -46.84768978681289298, 25.58645032415531517, -1.575055156418467162 ) ) ;
#20082=LINE ( 'NONE', #735, #17930 ) ;
#20083=CARTESIAN_POINT ( 'NONE',  ( -29.67105550538132519, 68.29201113456635142, -1.524000000002203814 ) ) ;
#20084=DIRECTION ( 'NONE',  ( 5.188838149069472160E-16, -1.699382548006136559E-16, -1.000000000000000000 ) ) ;
#20087=CARTESIAN_POINT ( 'NONE',  ( -58.50860430493788300, 0.7049166599848583070, 0.9756837515128382599 ) ) ;
#20089=CARTESIAN_POINT ( 'NONE',  ( -56.34046819891496938, 4.202508019718290022, 2.501728563949842776 ) ) ;
#20091=VERTEX_POINT ( 'NONE', #10734 ) ;
#20092=CARTESIAN_POINT ( 'NONE',  ( -57.34105142390577470, 4.241571993195747403, -0.1395372036360086054 ) ) ;
#20095=DIRECTION ( 'NONE',  ( 0.7770581983690815209, -0.6294287539884060312, 5.101669463485828849E-16 ) ) ;
#20105=FACE_OUTER_BOUND ( 'NONE', #1333, .T. ) ;
#20108=VERTEX_POINT ( 'NONE', #39515 ) ;
#20112=CARTESIAN_POINT ( 'NONE',  ( -57.39693641392964452, 1.805818221422732961, -1.488717331793851795 ) ) ;
#20124=DIRECTION ( 'NONE',  ( 5.188838149069472160E-16, -1.699382548006136559E-16, -1.000000000000000000 ) ) ;
#20127=CARTESIAN_POINT ( 'NONE',  ( -51.34009458250667279, 14.66650723912346699, -4.800162786360146150 ) ) ;
#20134=EDGE_CURVE ( 'NONE', #30025, #37691, #10802, .T. ) ;
#20137=CIRCLE ( 'NONE', #31025, 0.2539999999999993929 ) ;
#20139=CARTESIAN_POINT ( 'NONE',  ( -42.48565245465144358, 21.90714463913272780, -1.692305106577525198 ) ) ;
#20140=ORIENTED_EDGE ( 'NONE', *, *, #15680, .F. ) ;
#20146=CARTESIAN_POINT ( 'NONE',  ( -46.48504882799048232, 25.86691234155827246, -1.524000000000011346 ) ) ;
#20156=DIRECTION ( 'NONE',  ( 0.6825627711659328911, 0.7308269722843309113, 2.299753143848213649E-16 ) ) ;
#20160=CARTESIAN_POINT ( 'NONE',  ( -57.21909960282354035, 2.250382150496072597, -1.879871960369849271 ) ) ;
#20161=DIRECTION ( 'NONE',  ( 5.188838149069472160E-16, -1.699382548006136559E-16, -1.000000000000000000 ) ) ;
#20165=VERTEX_POINT ( 'NONE', #39383 ) ;
#20172=VERTEX_POINT ( 'NONE', #19140 ) ;
#20174=DIRECTION ( 'NONE',  ( -0.8745520943968249084, 0.4849315768086533418, -5.311926654347176508E-16 ) ) ;
#20176=AXIS2_PLACEMENT_3D ( 'NONE', #8774, #12387, #21314 ) ;
#20183=CARTESIAN_POINT ( 'NONE',  ( -57.92213827294109763, 0.6733716272070394693, 0.9587715765150526259 ) ) ;
#20184=CARTESIAN_POINT ( 'NONE',  ( -48.05879467440716013, 25.10120116127142964, 0.1605504162684488478 ) ) ;
#20185=CARTESIAN_POINT ( 'NONE',  ( -56.04137470801128273, 5.508142037592367757, 2.879222540163115074 ) ) ;
#20186=CARTESIAN_POINT ( 'NONE',  ( -57.60563996024792743, 1.910284663404326233, 1.727869274997176907 ) ) ;
#20188=CARTESIAN_POINT ( 'NONE',  ( -58.37241122568488549, -0.2962816677227753104, -1.028586707908062104E-14 ) ) ;
#20189=AXIS2_PLACEMENT_3D ( 'NONE', #15378, #15163, #28170 ) ;
#20191=CARTESIAN_POINT ( 'NONE',  ( -45.45367893016184979, 22.54667639846615046, 3.012003376585078662 ) ) ;
#20201=CARTESIAN_POINT ( 'NONE',  ( -17.14500000000466784, 71.11999999999886768, -1.270000000000000684 ) ) ;
#20213=EDGE_LOOP ( 'NONE', ( #33351, #18797, #11045, #17972 ) ) ;
#20214=CARTESIAN_POINT ( 'NONE',  ( -43.08902205111511563, 20.96483665317663991, 0.2987222196696301402 ) ) ;
#20224=CIRCLE ( 'NONE', #25684, 0.2539999999999973390 ) ;
#20225=ORIENTED_EDGE ( 'NONE', *, *, #22058, .T. ) ;
#20246=DIRECTION ( 'NONE',  ( 5.188838149069472160E-16, -1.699382548006136559E-16, -1.000000000000000000 ) ) ;
#20251=FACE_OUTER_BOUND ( 'NONE', #36804, .T. ) ;
#20252=FACE_OUTER_BOUND ( 'NONE', #8103, .T. ) ;
#20253=ORIENTED_EDGE ( 'NONE', *, *, #26109, .F. ) ;
#20258=CARTESIAN_POINT ( 'NONE',  ( -58.68158197657997022, -0.3140746753423795390, -0.3081004635821821824 ) ) ;
#20259=ORIENTED_EDGE ( 'NONE', *, *, #40422, .T. ) ;
#20260=CARTESIAN_POINT ( 'NONE',  ( -58.36222274556654099, -0.2757005147482338714, -0.1096927518867439194 ) ) ;
#20264=DIRECTION ( 'NONE',  ( 0.8745520943968240202, -0.4849315768086553402, 6.829619984160650158E-16 ) ) ;
#20271=ORIENTED_EDGE ( 'NONE', *, *, #7752, .T. ) ;
#20274=CARTESIAN_POINT ( 'NONE',  ( -49.24775882308124864, 17.43196194296904267, 5.046047204421642007 ) ) ;
#20275=ADVANCED_FACE ( 'NONE', ( #20390 ), #27788, .T. ) ;
#20282=CARTESIAN_POINT ( 'NONE',  ( -55.83515739322315596, 4.224161455597911008, -0.1887094293950861423 ) ) ;
#20285=CARTESIAN_POINT ( 'NONE',  ( -30.50798996576767763, 65.61473877417354572, -1.270000000000006901 ) ) ;
#20287=CARTESIAN_POINT ( 'NONE',  ( -30.03903471085840238, 57.95649848198893750, -1.523999999999813282 ) ) ;
#20290=FACE_OUTER_BOUND ( 'NONE', #35709, .T. ) ;
#20291=CARTESIAN_POINT ( 'NONE',  ( -58.69054519303719530, 0.2722345423086247607, 0.6021937201626180736 ) ) ;
#20295=CARTESIAN_POINT ( 'NONE',  ( -56.07077906059188166, 6.725046902222183931, -2.233835758070444655 ) ) ;
#20297=AXIS2_PLACEMENT_3D ( 'NONE', #32890, #318, #7326 ) ;
#20299=CARTESIAN_POINT ( 'NONE',  ( -17.14500000000466784, 71.11999999999886768, -1.270000000000000684 ) ) ;
#20302=AXIS2_PLACEMENT_3D ( 'NONE', #15445, #28448, #12258 ) ;
#20310=DIRECTION ( 'NONE',  ( 0.1906721105965039909, -0.9816537812491094028, 2.657572025465702696E-16 ) ) ;
#20311=DIRECTION ( 'NONE',  ( 5.188838149069472160E-16, -1.699382548006136559E-16, -1.000000000000000000 ) ) ;
#20314=CARTESIAN_POINT ( 'NONE',  ( -58.09428082180522779, 0.3001999070928298430, -0.7274870244324989077 ) ) ;
#20319=CARTESIAN_POINT ( 'NONE',  ( -46.07906060731711761, 24.80782705053048076, -1.769089518196001798 ) ) ;
#20329=EDGE_CURVE ( 'NONE', #26503, #2001, #4021, .T. ) ;
#20330=CARTESIAN_POINT ( 'NONE',  ( -54.98111839650035648, 8.542840639972862249, -3.427624633821342304 ) ) ;
#20334=CIRCLE ( 'NONE', #23744, 0.7620000000000000107 ) ;
#20338=EDGE_CURVE ( 'NONE', #27342, #19390, #18262, .T. ) ;
#20340=DIRECTION ( 'NONE',  ( 5.188838149069472160E-16, -1.699382548006136559E-16, -1.000000000000000000 ) ) ;
#20341=CARTESIAN_POINT ( 'NONE',  ( -33.20758249455312239, 49.81222039523557044, -1.524000000000005572 ) ) ;
#20344=EDGE_CURVE ( 'NONE', #30637, #34369, #38014, .T. ) ;
#20346=CARTESIAN_POINT ( 'NONE',  ( -47.16908398257407953, 25.15707121737368013, -1.640988021986792500 ) ) ;
#20354=ORIENTED_EDGE ( 'NONE', *, *, #37346, .F. ) ;
#20359=AXIS2_PLACEMENT_3D ( 'NONE', #27368, #5806, #34764 ) ;
#20360=CARTESIAN_POINT ( 'NONE',  ( -4.466782427718574588, 71.06098887363195615, -1.523999999999994248 ) ) ;
#20361=ORIENTED_EDGE ( 'NONE', *, *, #8325, .F. ) ;
#20363=AXIS2_PLACEMENT_3D ( 'NONE', #24877, #15281, #22083 ) ;
#20366=CARTESIAN_POINT ( 'NONE',  ( -57.50985127144645048, 1.621858126758690455, -1.632528232182590466 ) ) ;
#20367=DIRECTION ( 'NONE',  ( 0.4849315768086389089, 0.8745520943968330130, 4.371515779989697137E-15 ) ) ;
#20371=EDGE_CURVE ( 'NONE', #27023, #12982, #23707, .T. ) ;
#20372=VERTEX_POINT ( 'NONE', #22016 ) ;
#20375=DIRECTION ( 'NONE',  ( 5.188838149069472160E-16, -1.699382548006136559E-16, -1.000000000000000000 ) ) ;
#20377=EDGE_LOOP ( 'NONE', ( #26971, #32427, #26577, #28941 ) ) ;
#20384=LINE ( 'NONE', #7843, #19915 ) ;
#20387=CARTESIAN_POINT ( 'NONE',  ( -26.51793118801306548, 72.98537704160715123, -1.270000000000006013 ) ) ;
#20388=CARTESIAN_POINT ( 'NONE',  ( -57.73720092555902283, 1.073063965931175145, 1.165893645650359911 ) ) ;
#20389=CARTESIAN_POINT ( 'NONE',  ( -48.33886291794431145, 23.55519408767752054, 1.110521498696428910 ) ) ;
#20390=FACE_OUTER_BOUND ( 'NONE', #6658, .T. ) ;
#20391=CARTESIAN_POINT ( 'NONE',  ( -52.97391985390434144, 12.30611266682019789, 4.247241762254901687 ) ) ;
#20392=CARTESIAN_POINT ( 'NONE',  ( -58.18395191960946278, 0.6639886956250335981, 1.155333695069822975 ) ) ;
#20397=CARTESIAN_POINT ( 'NONE',  ( -45.76673701974917208, 25.51931200435043934, 1.523999999999991806 ) ) ;
#20407=CARTESIAN_POINT ( 'NONE',  ( -46.48963984823834039, 20.58996865087918238, 4.821990630911828113 ) ) ;
#20419=EDGE_CURVE ( 'NONE', #1859, #34293, #31833, .T. ) ;
#20421=VERTEX_POINT ( 'NONE', #35249 ) ;
#20422=CARTESIAN_POINT ( 'NONE',  ( -53.87733401397680666, 8.744676589845553849, 2.811092830483123084 ) ) ;
#20428=EDGE_LOOP ( 'NONE', ( #5580, #14828, #26300 ) ) ;
#20439=AXIS2_PLACEMENT_3D ( 'NONE', #38044, #5687, #31009 ) ;
#20440=CARTESIAN_POINT ( 'NONE',  ( -9.960492004070044203, 64.81807050032566053, 1.270000000000003126 ) ) ;
#20443=AXIS2_PLACEMENT_3D ( 'NONE', #3441, #20024, #16836 ) ;
#20448=ORIENTED_EDGE ( 'NONE', *, *, #12552, .F. ) ;
#20452=DIRECTION ( 'NONE',  ( 0.7770581983690701966, -0.6294287539884197979, 8.537024980200731099E-16 ) ) ;
#20456=CARTESIAN_POINT ( 'NONE',  ( -11.24191166894635074, 82.34025985790688651, -1.269999999999999574 ) ) ;
#20462=CYLINDRICAL_SURFACE ( 'NONE', #10021, 0.2539999999999998925 ) ;
#20468=EDGE_CURVE ( 'NONE', #20372, #26546, #1306, .T. ) ;
#20471=CARTESIAN_POINT ( 'NONE',  ( -58.36582417653014687, -0.2832568706219312782, -0.07935633695538733823 ) ) ;
#20477=VECTOR ( 'NONE', #13169, 1000.000000000000000 ) ;
#20482=EDGE_LOOP ( 'NONE', ( #39031, #24548, #26105, #23754 ) ) ;
#20485=CARTESIAN_POINT ( 'NONE',  ( -57.87993506102255736, 0.7648122704443233166, 1.011066771891486749 ) ) ;
#20493=CARTESIAN_POINT ( 'NONE',  ( -56.38098843839168950, 3.837951075127326916, -1.838241461164923596 ) ) ;
#20495=FACE_OUTER_BOUND ( 'NONE', #16165, .T. ) ;
#20496=VECTOR ( 'NONE', #17464, 1000.000000000000114 ) ;
#20498=CARTESIAN_POINT ( 'NONE',  ( -46.84878041887307631, 25.58252992934718861, -1.577652289021667986 ) ) ;
#20499=DIRECTION ( 'NONE',  ( 0.9998239923360758841, -0.01876124593811817620, 2.121609341712732885E-15 ) ) ;
#20500=CARTESIAN_POINT ( 'NONE',  ( -30.30981065304866107, 56.20484928089094012, -1.524000000000004240 ) ) ;
#20504=CARTESIAN_POINT ( 'NONE',  ( -58.35673254475433680, 1.205555466438051893, 0.1480423017862440571 ) ) ;
#20505=CARTESIAN_POINT ( 'NONE',  ( -58.73801720703743001, -0.4998429216807459552, -1.049519136981926467E-14 ) ) ;
#20508=CARTESIAN_POINT ( 'NONE',  ( -57.92935616279446265, 2.416188466839983118, -0.2259612492382147286 ) ) ;
#20509=DIRECTION ( 'NONE',  ( -0.8745520943968249084, 0.4849315768086533418, -5.271987356194193006E-16 ) ) ;
#20511=CARTESIAN_POINT ( 'NONE',  ( -45.67969256299926428, 21.13156854447444744, -4.214927840907465750 ) ) ;
#20518=CARTESIAN_POINT ( 'NONE',  ( -6.422645615570758970, 77.88548590848095898, -1.269999999999996465 ) ) ;
#20522=DIRECTION ( 'NONE',  ( -0.8745520943968240202, 0.4849315768086551737, -5.361993529360572958E-16 ) ) ;
#20525=CARTESIAN_POINT ( 'NONE',  ( -58.06686319096232296, 0.3595372361034740449, -0.7669821491821283699 ) ) ;
#20531=CARTESIAN_POINT ( 'NONE',  ( -45.45367893016184979, 22.54667639846615046, -3.012003376585093317 ) ) ;
#20538=DIRECTION ( 'NONE',  ( 5.188838149069472160E-16, -1.699382548006136559E-16, -1.000000000000000000 ) ) ;
#20540=CARTESIAN_POINT ( 'NONE',  ( -56.34046819891496938, 4.202508019718290022, -2.501728563949862760 ) ) ;
#20544=AXIS2_PLACEMENT_3D ( 'NONE', #34780, #37338, #40549 ) ;
#20552=CARTESIAN_POINT ( 'NONE',  ( -57.85534701229749999, 0.8496279762696401505, 1.203237356453207063 ) ) ;
#20555=CARTESIAN_POINT ( 'NONE',  ( -47.09845139715251605, 25.49303147219070098, -0.5484243623142366353 ) ) ;
#20558=ORIENTED_EDGE ( 'NONE', *, *, #1925, .F. ) ;
#20559=CARTESIAN_POINT ( 'NONE',  ( -9.712308604790303335, 65.53852105402241079, -1.269999999999996021 ) ) ;
#20565=EDGE_CURVE ( 'NONE', #4600, #11324, #28473, .T. ) ;
#20566=VERTEX_POINT ( 'NONE', #29260 ) ;
#20568=ADVANCED_FACE ( 'NONE', ( #33103 ), #3293, .F. ) ;
#20570=DIRECTION ( 'NONE',  ( 0.01731298258487879230, -0.9998501190848636533, 2.678710623147156226E-15 ) ) ;
#20573=ORIENTED_EDGE ( 'NONE', *, *, #40422, .F. ) ;
#20577=CARTESIAN_POINT ( 'NONE',  ( -58.64342337385304660, -0.3142157529030242813, -0.3359497956441734878 ) ) ;
#20584=CARTESIAN_POINT ( 'NONE',  ( -45.61851195612215548, 20.88128798641532313, 4.109017096223889887 ) ) ;
#20590=AXIS2_PLACEMENT_3D ( 'NONE', #11184, #30574, #17369 ) ;
#20598=CARTESIAN_POINT ( 'NONE',  ( -55.46911355273442013, 5.859935818251603479, 2.757237622174628644 ) ) ;
#20599=CARTESIAN_POINT ( 'NONE',  ( -47.66286930719412851, 20.62480072838431155, 5.054501799269492501 ) ) ;
#20600=CARTESIAN_POINT ( 'NONE',  ( -50.36516092884956208, 15.79195539882771726, 4.916963016749596349 ) ) ;
#20601=CARTESIAN_POINT ( 'NONE',  ( -58.46107188299979640, 0.06432868000574894218, 0.7596429210606043814 ) ) ;
#20604=ORIENTED_EDGE ( 'NONE', *, *, #15331, .F. ) ;
#20605=CARTESIAN_POINT ( 'NONE',  ( -42.79661761208809168, 21.81806929429799879, 2.089873509012810882 ) ) ;
#20608=AXIS2_PLACEMENT_3D ( 'NONE', #37661, #8690, #8898 ) ;
#20616=CARTESIAN_POINT ( 'NONE',  ( -20.21600168833980149, 80.16988503754176065, 1.269999999999995355 ) ) ;
#20617=AXIS2_PLACEMENT_3D ( 'NONE', #26575, #39802, #23574 ) ;
#20618=CARTESIAN_POINT ( 'NONE',  ( -45.89458612274084714, 20.88821703128090235, 4.453918368558905883 ) ) ;
#20628=AXIS2_PLACEMENT_3D ( 'NONE', #35872, #10076, #9657 ) ;
#20630=ORIENTED_EDGE ( 'NONE', *, *, #26749, .T. ) ;
#20632=CARTESIAN_POINT ( 'NONE',  ( -49.58053446479453186, 16.59387910164543456, 4.528212452174703806 ) ) ;
#20637=ORIENTED_EDGE ( 'NONE', *, *, #10507, .T. ) ;
#20644=EDGE_CURVE ( 'NONE', #42027, #38617, #1974, .T. ) ;
#20648=CARTESIAN_POINT ( 'NONE',  ( -17.32429653712378936, 61.56493206124108042, -1.523999999999999355 ) ) ;
#20650=AXIS2_PLACEMENT_3D ( 'NONE', #6074, #13502, #3513 ) ;
#20654=AXIS2_PLACEMENT_3D ( 'NONE', #3550, #26309, #355 ) ;
#20658=CARTESIAN_POINT ( 'NONE',  ( -8.095114962461808616, 74.19100168833409725, -1.269999999999996687 ) ) ;
#20664=AXIS2_PLACEMENT_3D ( 'NONE', #36716, #24124, #37544 ) ;
#20667=DIRECTION ( 'NONE',  ( -0.8745520943968243532, 0.4849315768086547296, -6.829619984160642269E-16 ) ) ;
#20670=CARTESIAN_POINT ( 'NONE',  ( -46.95911617132933458, 24.98948415085536823, -1.986615011824472088 ) ) ;
#20677=DIRECTION ( 'NONE',  ( 0.7548010569845196027, 0.6559537821943342006, 6.697925912855741462E-15 ) ) ;
#20680=AXIS2_PLACEMENT_3D ( 'NONE', #40155, #13527, #20522 ) ;
#20686=CARTESIAN_POINT ( 'NONE',  ( -10.44685452804831804, 82.62549350906336088, -1.523999999999999355 ) ) ;
#20688=FILL_AREA_STYLE ('',( #23455 ) ) ;
#20690=CARTESIAN_POINT ( 'NONE',  ( -46.44929277073200069, 20.74717582246854874, 4.783910118526112143 ) ) ;
#20698=ORIENTED_EDGE ( 'NONE', *, *, #40520, .T. ) ;
#20701=CARTESIAN_POINT ( 'NONE',  ( -56.97096143714178140, 2.717004285893040549, 1.832255202882757450 ) ) ;
#20710=EDGE_CURVE ( 'NONE', #15145, #4252, #22633, .T. ) ;
#20711=CARTESIAN_POINT ( 'NONE',  ( -51.86985193027732066, 10.34936321858913999, -0.3560079035465085751 ) ) ;
#20714=FACE_OUTER_BOUND ( 'NONE', #23115, .T. ) ;
#20719=DIRECTION ( 'NONE',  ( -0.8745520943968243532, 0.4849315768086547296, -5.361993529360573944E-16 ) ) ;
#20720=CARTESIAN_POINT ( 'NONE',  ( -58.79341205368594814, 0.01963237121659078266, 0.1476394306258261846 ) ) ;
#20723=ORIENTED_EDGE ( 'NONE', *, *, #29039, .F. ) ;
#20724=CARTESIAN_POINT ( 'NONE',  ( -57.40598286442868670, 3.481741809872221260, -1.566274799519931760 ) ) ;
#20735=CARTESIAN_POINT ( 'NONE',  ( -51.03866287897986354, 14.58798107696808444, -4.681202568652266471 ) ) ;
#20740=CARTESIAN_POINT ( 'NONE',  ( -57.37058287830014791, 1.862367624825627788, -1.511443718440989459 ) ) ;
#20744=CARTESIAN_POINT ( 'NONE',  ( -44.13308345971568514, 24.21351174012166396, -1.567149544246662973 ) ) ;
#20745=CARTESIAN_POINT ( 'NONE',  ( -8.584014518950164430, 73.13423810798757074, -1.269999999999996687 ) ) ;
#20752=DIRECTION ( 'NONE',  ( -0.9816537812491126225, -0.1906721105964872265, -8.537024980200846470E-16 ) ) ;
#20754=CARTESIAN_POINT ( 'NONE',  ( -49.59816314059867182, 17.91649583374774224, -5.069000701391666475 ) ) ;
#20755=DIRECTION ( 'NONE',  ( -0.8745520943968225769, 0.4849315768086578382, -5.691349986800571545E-16 ) ) ;
#20757=DIRECTION ( 'NONE',  ( 0.01731298258488073172, -0.9998501190848634312, 1.788962107505278366E-16 ) ) ;
#20759=B_SPLINE_CURVE_WITH_KNOTS ( 'NONE', 3,
 ( #41114, #34310, #5548, #35142 ),
 .UNSPECIFIED., .F., .F.,
 ( 4, 4 ),
 ( 0.000000000000000000, 6.355780391027510178E-05 ),
 .UNSPECIFIED. ) ;
#20763=LINE ( 'NONE', #33788, #17894 ) ;
#20765=CARTESIAN_POINT ( 'NONE',  ( -57.68935019796909813, 1.134378438699040759, 1.023808352551137890 ) ) ;
#20769=CARTESIAN_POINT ( 'NONE',  ( -46.91604881613258016, 25.30076613767155180, -1.786867259277526543 ) ) ;
#20771=CARTESIAN_POINT ( 'NONE',  ( -46.38316532014823679, 26.05065462784537900, -1.524000000000008459 ) ) ;
#20777=DIRECTION ( 'NONE',  ( -0.9454731675810331692, 0.3256999990547864154, 8.329459401252003088E-15 ) ) ;
#20782=CARTESIAN_POINT ( 'NONE',  ( -41.06677624517580227, 23.07857903943744304, -1.269999999997401652 ) ) ;
#20783=PLANE ( 'NONE',  #6787 ) ;
#20788=CARTESIAN_POINT ( 'NONE',  ( -58.82782897837071800, -0.2608788304223202958, -0.04583423360434937810 ) ) ;
#20796=LINE ( 'NONE', #33821, #7729 ) ;
#20798=CIRCLE ( 'NONE', #30331, 0.2540000000000010583 ) ;
#20802=CARTESIAN_POINT ( 'NONE',  ( -46.87509351769019617, 25.14555728883381391, -1.859034946739896776 ) ) ;
#20809=CARTESIAN_POINT ( 'NONE',  ( -57.57924614125985840, 1.413868729064180707, 1.323882363220449054 ) ) ;
#20810=DIRECTION ( 'NONE',  ( -0.9454731675810336133, 0.3256999990547843615, -5.459396135145337199E-16 ) ) ;
#20811=CARTESIAN_POINT ( 'NONE',  ( -57.69570286664291103, 2.558035660193719529, 1.875687456014364152 ) ) ;
#20812=CARTESIAN_POINT ( 'NONE',  ( -58.49135324493490629, -0.001359889153940653820, 0.7038351056170361053 ) ) ;
#20817=CARTESIAN_POINT ( 'NONE',  ( -47.20791569504335428, 21.28685671521062517, 4.803936552638831792 ) ) ;
#20828=CARTESIAN_POINT ( 'NONE',  ( -29.81357423954495189, 70.62209452652477637, -1.524000000000007349 ) ) ;
#20829=CARTESIAN_POINT ( 'NONE',  ( -44.83891394770468963, 21.39113109692259940, 3.507332325251830252 ) ) ;
#20831=CARTESIAN_POINT ( 'NONE',  ( -41.05190940396061450, 23.09449711908037983, 1.270000000023963960 ) ) ;
#20842=ORIENTED_EDGE ( 'NONE', *, *, #40560, .F. ) ;
#20843=CARTESIAN_POINT ( 'NONE',  ( -48.39470387610976587, 16.07729130905085313, 1.622931888101216691 ) ) ;
#20848=ORIENTED_EDGE ( 'NONE', *, *, #38908, .F. ) ;
#20853=ORIENTED_EDGE ( 'NONE', *, *, #9662, .F. ) ;
#20858=EDGE_CURVE ( 'NONE', #36274, #26682, #9437, .T. ) ;
#20866=EDGE_CURVE ( 'NONE', #4252, #31622, #31879, .T. ) ;
#20872=FACE_OUTER_BOUND ( 'NONE', #22102, .T. ) ;
#20873=DIRECTION ( 'NONE',  ( -0.8745520943968220218, 0.4849315768086588374, -4.268512490100437040E-16 ) ) ;
#20875=CIRCLE ( 'NONE', #13443, 0.2540000000000022795 ) ;
#20877=PLANE ( 'NONE',  #23057 ) ;
#20883=DIRECTION ( 'NONE',  ( -0.9454731675810330582, 0.3256999990547864710, -3.976957304636361482E-16 ) ) ;
#20890=EDGE_CURVE ( 'NONE', #26382, #5685, #33257, .T. ) ;
#20891=ORIENTED_EDGE ( 'NONE', *, *, #691, .T. ) ;
#20894=AXIS2_PLACEMENT_3D ( 'NONE', #2843, #3053, #9632 ) ;
#20902=DIRECTION ( 'NONE',  ( -0.8745520943968245753, 0.4849315768086539524, -5.691349986800526185E-16 ) ) ;
#20904=ORIENTED_EDGE ( 'NONE', *, *, #28211, .T. ) ;
#20911=CARTESIAN_POINT ( 'NONE',  ( -58.44182880578495087, -0.4131463110825606133, 0.3217794782789726860 ) ) ;
#20919=CARTESIAN_POINT ( 'NONE',  ( -57.76865908382304582, 0.8624112519253351872, -0.3783812474403069337 ) ) ;
#20921=DIRECTION ( 'NONE',  ( -0.8745520943968235761, 0.4849315768086558398, -4.268512490100410909E-16 ) ) ;
#20922=CARTESIAN_POINT ( 'NONE',  ( -46.95911617132933458, 24.98948415085536823, -1.986615011824472088 ) ) ;
#20924=LINE ( 'NONE', #4778, #27022 ) ;
#20926=DIRECTION ( 'NONE',  ( -0.8745520943968243532, 0.4849315768086547296, -5.361993529360573944E-16 ) ) ;
#20928=CARTESIAN_POINT ( 'NONE',  ( -57.89852354142710311, 2.261894840748110536, 1.235920526244124851 ) ) ;
#20931=ORIENTED_EDGE ( 'NONE', *, *, #30286, .T. ) ;
#20932=CARTESIAN_POINT ( 'NONE',  ( -56.17386367503594613, 7.314326147911789811, -0.9214986423944944161 ) ) ;
#20933=ADVANCED_FACE ( 'NONE', ( #7746 ), #16907, .T. ) ;
#20935=FACE_OUTER_BOUND ( 'NONE', #2124, .T. ) ;
#20939=( GEOMETRIC_REPRESENTATION_CONTEXT ( 3 ) GLOBAL_UNCERTAINTY_ASSIGNED_CONTEXT ( ( #26548 ) ) GLOBAL_UNIT_ASSIGNED_CONTEXT ( ( #7512, #1549, #17079 ) ) REPRESENTATION_CONTEXT ( 'NONE', 'WORKASPACE' ) );
#20941=CARTESIAN_POINT ( 'NONE',  ( -33.00685850039228342, 50.69800224577189596, 1.270000000006296537 ) ) ;
#20943=CARTESIAN_POINT ( 'NONE',  ( -50.91190571670057352, 14.80147821656241369, -4.713324810010480981 ) ) ;
#20947=CARTESIAN_POINT ( 'NONE',  ( -48.87447604115916988, 17.97958907615011981, -5.093074433551099567 ) ) ;
#20948=ADVANCED_FACE ( 'NONE', ( #20495 ), #41430, .T. ) ;
#20951=CARTESIAN_POINT ( 'NONE',  ( -48.98489377192316852, 18.65252824715059177, -5.272350768541925525 ) ) ;
#20959=ADVANCED_FACE ( 'NONE', ( #33944 ), #1989, .T. ) ;
#20962=CARTESIAN_POINT ( 'NONE',  ( -55.65298819915649631, 5.540485941798511504, -2.823722248809264368 ) ) ;
#20965=CARTESIAN_POINT ( 'NONE',  ( -23.75665686005077504, 76.91945007112674659, -1.270000000000005125 ) ) ;
#20967=B_SPLINE_CURVE_WITH_KNOTS ( 'NONE', 3,
 ( #39095, #6717, #19686, #32917, #16920, #29920, #32702, #17960, #24775, #8388, #18373, #21352, #27351, #14341, #36952, #5002, #11159, #40983, #27562, #37359, #24144, #27973, #33968, #40569, #8178, #40775, #34174, #37152, #17544, #4796, #27764, #2009, #1597, #7772, #40154, #5418, #5210, #40364, #7975, #37773, #14972, #31168, #1383, #31381, #14763, #23935, #18165, #17747, #21145, #20943, #30960, #11785, #11367, #24558, #20735, #1800, #8598, #21561, #34589, #30747, #11572, #33759, #37562, #2224, #27141, #34377, #10946, #4585, #30545, #14554, #24354, #2851, #12628, #25616, #22607, #2644, #21988, #18796, #15397, #38420, #29017, #5842, #9232, #2436, #19008, #16018, #15604, #38627, #8814, #22191, #3061, #12833, #42037, #41407, #35221, #28609, #37990, #32012, #35639, #19219, #6046, #21773, #12214, #28402, #25204, #41618, #22399, #6250, #38208, #41192, #34799, #19427, #32230, #15812, #31807, #28819, #25821, #35021, #9025, #5632, #6454, #38829, #18590, #35423, #9639, #12427, #25419, #41834, #24990, #9430, #32433, #15184, #28188, #11996, #31599, #39251, #19629, #39679, #6874, #23451, #26031, #16224, #32644, #7094, #36478, #13679, #73, #6666, #7298, #4115, #708, #26242, #23239, #33285, #285, #36273, #10058, #17075, #13258, #10481, #19846, #13041, #3480, #36059, #16440, #39040, #499, #20258, #20055, #3264, #16868, #29446, #23029, #9847, #26460, #32860, #29231, #13472, #10266, #3691, #39464, #16652, #33074 ),
 .UNSPECIFIED., .F., .F.,
 ( 4, 2, 2, 2, 1, 1, 2, 2, 2, 2, 1, 1, 1, 1, 1, 2, 2, 2, 2, 1, 1, 1, 1, 2, 2, 2, 1, 2, 2, 2, 1, 1, 1, 1, 2, 2, 2, 1, 1, 1, 1, 2, 2, 2, 2, 1, 1, 1, 1, 1, 2, 2, 2, 2, 2, 2, 1, 1, 1, 2, 2, 2, 2, 2, 1, 2, 1, 2, 2, 2, 2, 2, 2, 2, 1, 2, 2, 2, 2, 2, 2, 2, 1, 1, 2, 2, 2, 2, 2, 2, 1, 1, 2, 2, 2, 2, 2, 2, 2, 2, 2, 2, 2, 2, 2, 2, 2, 2, 4 ),
 ( 0.000000000000000000, 0.03125000000131424038, 0.04687500000197108996, 0.05468750000229992414, 0.05859375000246411225, 0.06054687500254619936, 0.06152343750258739558, 0.06250000000262859179, 0.09375000000393932109, 0.1093750000045946719, 0.1171875000049223542, 0.1210937500050864452, 0.1230468750051682963, 0.1240234375052087917, 0.1245117187552288313, 0.1247558593802386151, 0.1250000000052483851, 0.1406250000051884608, 0.1484375000051583182, 0.1523437500051430804, 0.1542968750051351978, 0.1552734375051311733, 0.1557617187551290361, 0.1560058593801280924, 0.1562500000051271210, 0.1718750000050420779, 0.1796875000049995841, 0.1835937500049780735, 0.1875000000049565629, 0.2187500000047861992, 0.2343750000047007953, 0.2421875000046579685, 0.2460937500046365689, 0.2480468750046257720, 0.2490234375046203597, 0.2500000000046149751, 0.3125000000042688630, 0.3437500000040961678, 0.3593750000040099035, 0.3671875000039666603, 0.3710937500039451775, 0.3730468750039344084, 0.3750000000039236947, 0.4375000000035705328, 0.4687500000033941183, 0.4843750000033057446, 0.4921875000032616687, 0.4960937500032398528, 0.4980468750032286951, 0.4990234375032232550, 0.4995117187532203684, 0.5000000000032174263, 0.6250000000024309443, 0.6875000000020378144, 0.7187500000018411939, 0.7343750000017429391, 0.7421875000016938673, 0.7460937500016691093, 0.7480468750016567858, 0.7490234375016504575, 0.7500000000016441293, 0.8125000000012420065, 0.8437500000010410561, 0.8593750000009408030, 0.8671875000008907319, 0.8710937500008657519, 0.8730468750008532064, 0.8740234375008467671, 0.8750000000008402168, 0.9062500000006236123, 0.9218750000005151435, 0.9296875000004609646, 0.9335937500004340972, 0.9355468750004206635, 0.9365234375004140022, 0.9370117187504105605, 0.9375000000004071188, 0.9531250000003018696, 0.9609375000002491340, 0.9648437500002227107, 0.9687500000001961764, 0.9726562500001697531, 0.9746093750001566525, 0.9755859375001501022, 0.9760742187501468825, 0.9765625000001436629, 0.9804687500001181277, 0.9824218750001054712, 0.9843750000000928146, 0.9863281250000801581, 0.9873046875000739409, 0.9877929687500708322, 0.9880371093750691669, 0.9882812500000676126, 0.9892578125000615064, 0.9897460937500585088, 0.9902343750000555112, 0.9907226562500525135, 0.9912109375000495159, 0.9914550781250479616, 0.9916992187500465183, 0.9919433593750449640, 0.9921875000000435207, 0.9941406250000325295, 0.9951171875000270894, 0.9960937500000216493, 0.9970703125000162093, 0.9980468750000107692, 1.000000000000000000 ),
 .UNSPECIFIED. ) ;
#20970=CARTESIAN_POINT ( 'NONE',  ( -4.085839532347240066, 71.06758511999679229, -1.269999999999994023 ) ) ;
#20975=CARTESIAN_POINT ( 'NONE',  ( -58.02159823468433331, 0.4660483771539991604, 0.8824573672536664137 ) ) ;
#20978=CARTESIAN_POINT ( 'NONE',  ( -47.59483747600737047, 24.73124547893296921, -0.7500189231788918498 ) ) ;
#20981=ORIENTED_EDGE ( 'NONE', *, *, #17060, .F. ) ;
#20989=EDGE_LOOP ( 'NONE', ( #19539, #801, #38778, #18494 ) ) ;
#20992=CARTESIAN_POINT ( 'NONE',  ( -43.26072192867658117, 21.85338993931741669, -2.263361967372762074 ) ) ;
#20993=ORIENTED_EDGE ( 'NONE', *, *, #34710, .F. ) ;
#20999=CARTESIAN_POINT ( 'NONE',  ( -57.40739589891802552, 2.334961046654995709, -1.895125133214725199 ) ) ;
#21007=EDGE_CURVE ( 'NONE', #2275, #4943, #14951, .T. ) ;
#21011=VERTEX_POINT ( 'NONE', #8365 ) ;
#21013=DIRECTION ( 'NONE',  ( -0.8745520943968247973, 0.4849315768086537304, -5.361993529360573944E-16 ) ) ;
#21014=CARTESIAN_POINT ( 'NONE',  ( -33.42971872652992005, 49.93539301574497102, -1.270000000000005569 ) ) ;
#21021=CARTESIAN_POINT ( 'NONE',  ( -56.02760103399240421, 4.702919582132905951, 2.444615905383621168 ) ) ;
#21023=CARTESIAN_POINT ( 'NONE',  ( -58.37934292759150168, 0.9822739792931106662, 1.208960021102198246 ) ) ;
#21024=CARTESIAN_POINT ( 'NONE',  ( -58.06568617868830984, 0.9193849054837686108, 1.293020708047914802 ) ) ;
#21029=CARTESIAN_POINT ( 'NONE',  ( -54.47970570282438274, 8.083255770631444292, 3.476097746275891076 ) ) ;
#21030=VECTOR ( 'NONE', #11004, 1000.000000000000000 ) ;
#21032=AXIS2_PLACEMENT_3D ( 'NONE', #20456, #17480, #14278 ) ;
#21040=FACE_OUTER_BOUND ( 'NONE', #20213, .T. ) ;
#21042=CARTESIAN_POINT ( 'NONE',  ( -48.28978369826177186, 19.63653578263565436, 5.206999999995388428 ) ) ;
#21046=DIRECTION ( 'NONE',  ( -0.1906721105965186736, 0.9816537812491066273, 0.000000000000000000 ) ) ;
#21054=CARTESIAN_POINT ( 'NONE',  ( -48.16508968810064317, 19.01313136326714925, 5.219744232931978978 ) ) ;
#21063=AXIS2_PLACEMENT_3D ( 'NONE', #35386, #39005, #6836 ) ;
#21068=FACE_OUTER_BOUND ( 'NONE', #3279, .T. ) ;
#21076=ORIENTED_EDGE ( 'NONE', *, *, #72, .T. ) ;
#21078=EDGE_CURVE ( 'NONE', #27616, #38171, #12860, .T. ) ;
#21085=CARTESIAN_POINT ( 'NONE',  ( -49.01671973967525275, 18.67808020721671625, 5.174630477995037836 ) ) ;
#21093=CARTESIAN_POINT ( 'NONE',  ( -17.32429653712378936, 61.56493206124108042, 1.269999999999999796 ) ) ;
#21098=EDGE_LOOP ( 'NONE', ( #17609, #27715, #1332, #19144 ) ) ;
#21099=ORIENTED_EDGE ( 'NONE', *, *, #21410, .T. ) ;
#21108=AXIS2_PLACEMENT_3D ( 'NONE', #36846, #8072, #21046 ) ;
#21111=EDGE_LOOP ( 'NONE', ( #35959, #7611, #37184, #5551 ) ) ;
#21114=CARTESIAN_POINT ( 'NONE',  ( -57.89036626108653394, 0.7933261799628198441, 1.256022413937592175 ) ) ;
#21123=CARTESIAN_POINT ( 'NONE',  ( -57.55293229875817218, 1.419684655164468623, -1.132508401016395716 ) ) ;
#21125=DIRECTION ( 'NONE',  ( -0.7770581983690864059, 0.6294287539884000360, -8.537024980200833651E-16 ) ) ;
#21126=DIRECTION ( 'NONE',  ( -0.1906721105965186736, 0.9816537812491066273, 0.000000000000000000 ) ) ;
#21130=CARTESIAN_POINT ( 'NONE',  ( -24.49496359545907964, 76.94162913054094588, 1.269999999999993578 ) ) ;
#21136=ORIENTED_EDGE ( 'NONE', *, *, #36077, .T. ) ;
#21137=CARTESIAN_POINT ( 'NONE',  ( -45.93641268020883928, 20.77718376653855614, -4.359287402722206828 ) ) ;
#21138=CIRCLE ( 'NONE', #19769, 0.6350000000000006750 ) ;
#21145=CARTESIAN_POINT ( 'NONE',  ( -50.78742080704162731, 15.01002293501888118, -4.744323022696246284 ) ) ;
#21148=CARTESIAN_POINT ( 'NONE',  ( -23.91048590848665611, 81.84235438443283783, -1.524000000000006239 ) ) ;
#21153=CARTESIAN_POINT ( 'NONE',  ( -46.89970385779243855, 22.02655025333852379, -4.237790764466935478 ) ) ;
#21160=CARTESIAN_POINT ( 'NONE',  ( -57.50953982388014651, 1.662011999372992044, -1.631050346940590812 ) ) ;
#21169=DIRECTION ( 'NONE',  ( -0.01731298258487590572, 0.9998501190848636533, -3.136208412989023577E-15 ) ) ;
#21171=CARTESIAN_POINT ( 'NONE',  ( -42.88395384449221126, 21.55219572468337219, -1.583305067638075769 ) ) ;
#21173=TOROIDAL_SURFACE ( 'NONE', #21032, 0.3810000000000001719, 0.2540000000000000036 ) ;
#21176=CARTESIAN_POINT ( 'NONE',  ( -58.03414100541873211, 0.4564111095344824953, 0.9708715263941498641 ) ) ;
#21177=CARTESIAN_POINT ( 'NONE',  ( -53.84631020981186822, 15.55534180636754193, -1.017045832751381207E-14 ) ) ;
#21180=CARTESIAN_POINT ( 'NONE',  ( -49.23607562092252721, 19.66429951101446960, -3.974467759520302401 ) ) ;
#21186=CIRCLE ( 'NONE', #2867, 0.7620000000000015650 ) ;
#21195=CARTESIAN_POINT ( 'NONE',  ( -47.85244527695891037, 19.39403540832952544, -5.219971639306605127 ) ) ;
#21196=ORIENTED_EDGE ( 'NONE', *, *, #17162, .T. ) ;
#21203=CARTESIAN_POINT ( 'NONE',  ( -56.37342374758011232, 3.980281407817629180, -2.237022232195863936 ) ) ;
#21208=ORIENTED_EDGE ( 'NONE', *, *, #13651, .F. ) ;
#21212=ADVANCED_FACE ( 'NONE', ( #24437 ), #8263, .F. ) ;
#21213=DIRECTION ( 'NONE',  ( -0.8745520943968250194, 0.4849315768086535083, -5.361993529360574930E-16 ) ) ;
#21216=DIRECTION ( 'NONE',  ( -0.8745520943967910465, 0.4849315768087146816, -5.424246918827960064E-16 ) ) ;
#21223=CARTESIAN_POINT ( 'NONE',  ( -17.97610982144389524, 83.97333317030323485, -1.270000000000003348 ) ) ;
#21224=CARTESIAN_POINT ( 'NONE',  ( -58.04761505321778259, 0.4012412707330069161, 0.7940720734374372425 ) ) ;
#21225=CARTESIAN_POINT ( 'NONE',  ( -33.20758249455312239, 49.81222039523557044, -1.524000000000005572 ) ) ;
#21227=CARTESIAN_POINT ( 'NONE',  ( -49.39499541695917628, 17.24413359080933006, 5.048280001787422755 ) ) ;
#21231=CARTESIAN_POINT ( 'NONE',  ( -4.476425760464393555, 71.61790547347303004, -1.269999999999994245 ) ) ;
#21233=CARTESIAN_POINT ( 'NONE',  ( -54.77668461537430034, 8.146287316968315650, 3.518595155146524434 ) ) ;
#21235=CARTESIAN_POINT ( 'NONE',  ( -23.69188486464780752, 78.08202335040543574, -1.524000000000005350 ) ) ;
#21243=DIRECTION ( 'NONE',  ( 0.3256999990547865265, 0.9454731675810330582, 7.920142172900908730E-15 ) ) ;
#21244=FACE_OUTER_BOUND ( 'NONE', #41182, .T. ) ;
#21245=CARTESIAN_POINT ( 'NONE',  ( -48.12235166104741779, 19.54369616526484776, 5.380337212813706138 ) ) ;
#21255=CIRCLE ( 'NONE', #31452, 0.2539999999999992819 ) ;
#21258=CARTESIAN_POINT ( 'NONE',  ( -50.52646075385809610, 14.05410990099204049, 2.888145277534006627 ) ) ;
#21262=VERTEX_POINT ( 'NONE', #9731 ) ;
#21269=VECTOR ( 'NONE', #30825, 1000.000000000000227 ) ;
#21270=ORIENTED_EDGE ( 'NONE', *, *, #31562, .T. ) ;
#21272=CYLINDRICAL_SURFACE ( 'NONE', #32665, 0.2540000000000030012 ) ;
#21276=CARTESIAN_POINT ( 'NONE',  ( -10.93398011767285283, 82.89560043784887000, -1.523999999999999577 ) ) ;
#21284=FACE_OUTER_BOUND ( 'NONE', #8169, .T. ) ;
#21290=AXIS2_PLACEMENT_3D ( 'NONE', #2503, #21213, #15039 ) ;
#21293=DIRECTION ( 'NONE',  ( -0.8745520943968235761, 0.4849315768086558398, -4.268512490100410909E-16 ) ) ;
#21299=ORIENTED_EDGE ( 'NONE', *, *, #11563, .T. ) ;
#21306=ORIENTED_EDGE ( 'NONE', *, *, #38625, .T. ) ;
#21309=CARTESIAN_POINT ( 'NONE',  ( -30.37855815223275258, 71.48694267763936239, -1.270000000000007567 ) ) ;
#21312=AXIS2_PLACEMENT_3D ( 'NONE', #12255, #25248, #22034 ) ;
#21314=DIRECTION ( 'NONE',  ( 0.9876665170007974393, -0.1565721916417901483, 8.537024980200831679E-16 ) ) ;
#21318=ORIENTED_EDGE ( 'NONE', *, *, #27411, .F. ) ;
#21321=CARTESIAN_POINT ( 'NONE',  ( -55.40724689662754088, 6.067898552042457538, 3.000206617154345778 ) ) ;
#21326=AXIS2_PLACEMENT_3D ( 'NONE', #33000, #29146, #22735 ) ;
#21330=CARTESIAN_POINT ( 'NONE',  ( -57.57967628038989005, 1.451576601202167360, -1.494865757154152153 ) ) ;
#21332=DIRECTION ( 'NONE',  ( 5.188838149069472160E-16, -1.699382548006136559E-16, -1.000000000000000000 ) ) ;
#21333=DIRECTION ( 'NONE',  ( -0.8745520943968235761, 0.4849315768086558953, -5.361993529360570985E-16 ) ) ;
#21338=CARTESIAN_POINT ( 'NONE',  ( -58.83227707057485389, -0.08366279997994163775, -1.543118586181777983E-14 ) ) ;
#21344=CARTESIAN_POINT ( 'NONE',  ( -47.22690022493117112, 20.09066223305544341, -5.151063612126583813 ) ) ;
#21352=CARTESIAN_POINT ( 'NONE',  ( -48.71344905023164529, 18.25307053356915787, -5.161295349598031379 ) ) ;
#21356=DIRECTION ( 'NONE',  ( -0.9469626219732538708, -0.3213437296502617002, -2.048706518008236507E-16 ) ) ;
#21359=CARTESIAN_POINT ( 'NONE',  ( -54.12303657725384198, 9.464413707472848714, -3.807237671326768602 ) ) ;
#21364=CIRCLE ( 'NONE', #27440, 0.3810000000000015041 ) ;
#21366=CARTESIAN_POINT ( 'NONE',  ( -58.23017998949752183, 0.6774554162835566551, -1.209604144815722426 ) ) ;
#21369=CARTESIAN_POINT ( 'NONE',  ( -17.08598887363762131, 83.79821757228496892, 1.269999999999997131 ) ) ;
#21370=EDGE_CURVE ( 'NONE', #16441, #31622, #24412, .T. ) ;
#21374=CARTESIAN_POINT ( 'NONE',  ( -41.87797633265722652, 22.30863410810708558, -1.617563149257741140 ) ) ;
#21375=VERTEX_POINT ( 'NONE', #25501 ) ;
#21378=CARTESIAN_POINT ( 'NONE',  ( -57.89731077922513691, 0.5615449381113218896, -1.013091259465030497E-14 ) ) ;
#21379=CARTESIAN_POINT ( 'NONE',  ( -51.68405183839315242, 20.46365084185837446, 0.3671080129528856428 ) ) ;
#21383=CARTESIAN_POINT ( 'NONE',  ( -49.54051387650593341, 20.87470723125096228, -2.270501476849551725 ) ) ;
#21391=DIRECTION ( 'NONE',  ( -0.1565721916418034709, -0.9876665170007954409, 8.659954811667512579E-17 ) ) ;
#21397=CARTESIAN_POINT ( 'NONE',  ( -41.23752580366542020, 23.26788267949596190, -1.523999999999987587 ) ) ;
#21398=LINE ( 'NONE', #28658, #23101 ) ;
#21403=CARTESIAN_POINT ( 'NONE',  ( -50.47813777547885650, 15.38220854283423122, -4.696510882186583302 ) ) ;
#21410=EDGE_CURVE ( 'NONE', #36274, #7253, #16103, .T. ) ;
#21414=EDGE_CURVE ( 'NONE', #5996, #18324, #38921, .T. ) ;
#21419=ORIENTED_EDGE ( 'NONE', *, *, #36060, .T. ) ;
#21428=B_SPLINE_CURVE_WITH_KNOTS ( 'NONE', 3,
 ( #15773, #22356, #41790, #22777, #12588, #28974, #12790, #35808, #6623, #3433 ),
 .UNSPECIFIED., .F., .F.,
 ( 4, 2, 2, 2, 4 ),
 ( 0.000000000000000000, 0.0001574456952392459016, 0.0003148913904784918032, 0.0004723370857177376777, 0.0006297827809569836064 ),
 .UNSPECIFIED. ) ;
#21429=DIRECTION ( 'NONE',  ( -0.8745520943968256855, 0.4849315768086519540, -5.691349986800502519E-16 ) ) ;
#21430=CARTESIAN_POINT ( 'NONE',  ( -58.35670767547218674, -0.2641613275777771053, 0.1431915459989163142 ) ) ;
#21431=CARTESIAN_POINT ( 'NONE',  ( -31.58045816419041074, 52.93464387131874815, -1.524000000000004684 ) ) ;
#21432=CARTESIAN_POINT ( 'NONE',  ( -43.82859865241511699, 24.63416949198730421, 1.523999999999992916 ) ) ;
#21435=ORIENTED_EDGE ( 'NONE', *, *, #32887, .T. ) ;
#21436=CARTESIAN_POINT ( 'NONE',  ( -48.04822308881583126, 19.89521662531995005, 5.294633059834397137 ) ) ;
#21443=ORIENTED_EDGE ( 'NONE', *, *, #31856, .T. ) ;
#21445=DIRECTION ( 'NONE',  ( 5.188838149069472160E-16, -1.699382548006136559E-16, -1.000000000000000000 ) ) ;
#21450=DIRECTION ( 'NONE',  ( 0.6294287539884133587, 0.7770581983690755257, 0.000000000000000000 ) ) ;
#21460=CARTESIAN_POINT ( 'NONE',  ( -56.90063064090522715, 2.680628813859151194, 1.231466298089183953 ) ) ;
#21461=CIRCLE ( 'NONE', #18734, 0.6350000000000014522 ) ;
#21467=EDGE_CURVE ( 'NONE', #34241, #26546, #7809, .T. ) ;
#21468=VERTEX_POINT ( 'NONE', #14378 ) ;
#21472=ORIENTED_EDGE ( 'NONE', *, *, #27686, .F. ) ;
#21474=CARTESIAN_POINT ( 'NONE',  ( -26.42106975583004314, 72.48669692073261217, -1.524000000000005794 ) ) ;
#21475=DIRECTION ( 'NONE',  ( 5.188838149069472160E-16, -1.699382548006136559E-16, -1.000000000000000000 ) ) ;
#21478=CARTESIAN_POINT ( 'NONE',  ( -46.60530155212503445, 26.17382724835477958, -1.524000000000008459 ) ) ;
#21481=CARTESIAN_POINT ( 'NONE',  ( -11.73534362491072258, 82.73994711668952107, 1.269999999999998241 ) ) ;
#21488=VECTOR ( 'NONE', #19816, 1000.000000000000000 ) ;
#21494=DIRECTION ( 'NONE',  ( -5.188838149069471174E-16, 1.699382548006136313E-16, 1.000000000000000000 ) ) ;
#21495=CARTESIAN_POINT ( 'NONE',  ( -58.83227707057483968, -0.08366279997992775996, 0.2458995907044888019 ) ) ;
#21504=EDGE_LOOP ( 'NONE', ( #17579, #19595, #9980, #11019 ) ) ;
#21512=DIRECTION ( 'NONE',  ( 0.8745520943968249084, -0.4849315768086533418, 5.311926654347176508E-16 ) ) ;
#21516=FACE_OUTER_BOUND ( 'NONE', #29797, .T. ) ;
#21521=DIRECTION ( 'NONE',  ( 0.6559537821943282054, -0.7548010569845248208, 8.537024980200704475E-16 ) ) ;
#21522=EDGE_CURVE ( 'NONE', #6398, #27753, #1421, .T. ) ;
#21525=AXIS2_PLACEMENT_3D ( 'NONE', #29320, #25908, #19508 ) ;
#21529=CARTESIAN_POINT ( 'NONE',  ( -57.74919803515417271, 1.101601998901911683, 1.404840701338397002 ) ) ;
#21535=AXIS2_PLACEMENT_3D ( 'NONE', #38194, #11557, #31155 ) ;
#21539=CARTESIAN_POINT ( 'NONE',  ( -57.84361080044246251, 0.8513586351276830611, -1.093731309501911886 ) ) ;
#21543=DIRECTION ( 'NONE',  ( 0.8745520943968472238, -0.4849315768086133738, 2.585085348184235087E-15 ) ) ;
#21550=VECTOR ( 'NONE', #6030, 1000.000000000000000 ) ;
#21552=CARTESIAN_POINT ( 'NONE',  ( -58.77954282417582732, 0.05649391281087323691, -0.1080441935232595435 ) ) ;
#21553=ORIENTED_EDGE ( 'NONE', *, *, #25593, .F. ) ;
#21561=CARTESIAN_POINT ( 'NONE',  ( -51.88968468915965104, 13.12277401453617820, -4.448989927898648666 ) ) ;
#21564=DIRECTION ( 'NONE',  ( -5.188838149069471174E-16, 1.699382548006136313E-16, 1.000000000000000000 ) ) ;
#21566=CARTESIAN_POINT ( 'NONE',  ( -53.67394638921515337, 9.465966177595170450, -3.594732514767734255 ) ) ;
#21569=CARTESIAN_POINT ( 'NONE',  ( -54.47970570282438274, 8.083255770631444292, -3.476097746275910172 ) ) ;
#21571=ADVANCED_FACE ( 'NONE', ( #27388 ), #30582, .F. ) ;
#21577=CARTESIAN_POINT ( 'NONE',  ( -58.55221842960730783, 0.5754175076986972615, -0.9757793345693789311 ) ) ;
#21578=DIRECTION ( 'NONE',  ( -5.188838149069472160E-16, 1.699382548006136559E-16, 1.000000000000000000 ) ) ;
#21580=CARTESIAN_POINT ( 'NONE',  ( -10.18297664959815663, 77.66688486464208552, -1.523999999999998245 ) ) ;
#21583=CARTESIAN_POINT ( 'NONE',  ( -58.70413935429054675, 0.2332485698458008905, -0.6626129746612972049 ) ) ;
#21584=CARTESIAN_POINT ( 'NONE',  ( -41.05189575270517821, 23.09451173561983950, -1.524000000000004462 ) ) ;
#21585=ORIENTED_EDGE ( 'NONE', *, *, #991, .F. ) ;
#21590=CARTESIAN_POINT ( 'NONE',  ( -51.08083271936510528, 17.88738476406025057, 2.973263991802279183 ) ) ;
#21592=VERTEX_POINT ( 'NONE', #36370 ) ;
#21593=CARTESIAN_POINT ( 'NONE',  ( -48.34142060212425207, 20.97662605846759831, -3.847193496378360056 ) ) ;
#21595=ADVANCED_FACE ( 'NONE', ( #1006 ), #13117, .T. ) ;
#21597=VERTEX_POINT ( 'NONE', #26766 ) ;
#21602=CARTESIAN_POINT ( 'NONE',  ( -29.91360363449003756, 70.04874496952835727, 1.269999999999992468 ) ) ;
#21605=DIRECTION ( 'NONE',  ( -0.8745520943968243532, 0.4849315768086547296, -5.361993529360573944E-16 ) ) ;
#21608=CARTESIAN_POINT ( 'NONE',  ( -42.67774629359277583, 22.12976331235084970, -1.921043605742120519 ) ) ;
#21609=ADVANCED_FACE ( 'NONE', ( #33370 ), #33169, .T. ) ;
#21621=ORIENTED_EDGE ( 'NONE', *, *, #1928, .T. ) ;
#21625=DIRECTION ( 'NONE',  ( -0.8745520943968241312, 0.4849315768086548406, -5.691349986800536046E-16 ) ) ;
#21626=COLOUR_RGB ( '', 0.40784314, 0.44705882, 0.49803922) ;
#21627=CARTESIAN_POINT ( 'NONE',  ( -11.43668055974971764, 78.14103736854400495, 1.270000000000000018 ) ) ;
#21629=ORIENTED_EDGE ( 'NONE', *, *, #12063, .T. ) ;
#21631=DIRECTION ( 'NONE',  ( -0.6294287539884133587, -0.7770581983690755257, 0.000000000000000000 ) ) ;
#21640=AXIS2_PLACEMENT_3D ( 'NONE', #9412, #6854, #32840 ) ;
#21641=CARTESIAN_POINT ( 'NONE',  ( -58.30092733718098685, -0.1459886894293531967, 0.3347744076924483725 ) ) ;
#21648=CARTESIAN_POINT ( 'NONE',  ( -51.81113891419111894, 13.24950054771400332, 4.495723625053109629 ) ) ;
#21654=EDGE_CURVE ( 'NONE', #25, #38897, #8804, .T. ) ;
#21655=ORIENTED_EDGE ( 'NONE', *, *, #14924, .T. ) ;
#21658=CARTESIAN_POINT ( 'NONE',  ( -41.09670346151854403, 23.04688172093030829, -1.270085369932534958 ) ) ;
#21660=CARTESIAN_POINT ( 'NONE',  ( -48.27156028472870020, 19.62643105735276450, 5.256042649956950363 ) ) ;
#21662=CIRCLE ( 'NONE', #12840, 0.2540000000000012248 ) ;
#21669=VECTOR ( 'NONE', #37817, 1000.000000000000227 ) ;
#21673=ORIENTED_EDGE ( 'NONE', *, *, #31398, .T. ) ;
#21674=CARTESIAN_POINT ( 'NONE',  ( -55.72901529264892417, 4.991126730481368234, 1.691135755076699665 ) ) ;
#21682=EDGE_LOOP ( 'NONE', ( #19790, #2597, #6505, #39158 ) ) ;
#21684=DIRECTION ( 'NONE',  ( 5.188838149069472160E-16, -1.699382548006136559E-16, -1.000000000000000000 ) ) ;
#21696=ORIENTED_EDGE ( 'NONE', *, *, #36960, .T. ) ;
#21698=EDGE_CURVE ( 'NONE', #4116, #6518, #5671, .T. ) ;
#21716=ORIENTED_EDGE ( 'NONE', *, *, #39652, .F. ) ;
#21722=ORIENTED_EDGE ( 'NONE', *, *, #13329, .T. ) ;
#21724=ORIENTED_EDGE ( 'NONE', *, *, #37282, .T. ) ;
#21730=AXIS2_PLACEMENT_3D ( 'NONE', #23343, #25713, #3150 ) ;
#21738=EDGE_LOOP ( 'NONE', ( #21931, #14822, #40893, #13084 ) ) ;
#21742=CARTESIAN_POINT ( 'NONE',  ( -56.80696390458998479, 3.604343092604281207, 2.316781442554533665 ) ) ;
#21745=CYLINDRICAL_SURFACE ( 'NONE', #4289, 0.5080000000000000071 ) ;
#21750=CARTESIAN_POINT ( 'NONE',  ( -57.60038635073813396, 1.097546858218847898, -0.08229580080366473427 ) ) ;
#21753=DIRECTION ( 'NONE',  ( -0.7308269722843147020, 0.6825627711659504326, -8.537024980200894788E-16 ) ) ;
#21756=ADVANCED_FACE ( 'NONE', ( #13462 ), #32051, .F. ) ;
#21758=CARTESIAN_POINT ( 'NONE',  ( -41.23752580366542730, 23.26788267949596190, 1.523999999999994248 ) ) ;
#21763=CARTESIAN_POINT ( 'NONE',  ( -58.32144855246983184, 1.173557705256414341, -1.098103182356013230 ) ) ;
#21765=DIRECTION ( 'NONE',  ( -0.1906721105965052399, 0.9816537812491094028, 7.161032787277034991E-15 ) ) ;
#21773=CARTESIAN_POINT ( 'NONE',  ( -57.56413824804958068, 1.999148952895605014, -1.762603608441677183 ) ) ;
#21774=ORIENTED_EDGE ( 'NONE', *, *, #24468, .T. ) ;
#21780=AXIS2_PLACEMENT_3D ( 'NONE', #13697, #26688, #40116 ) ;
#21782=CARTESIAN_POINT ( 'NONE',  ( -49.59816314059867182, 17.91649583374774224, -5.069000701391666475 ) ) ;
#21784=ORIENTED_EDGE ( 'NONE', *, *, #34150, .F. ) ;
#21789=CARTESIAN_POINT ( 'NONE',  ( -58.37241122568488549, -0.2962816677227753104, -1.034007718770489626E-14 ) ) ;
#21792=DIRECTION ( 'NONE',  ( -0.7517731442105912709, 0.6594218222380281436, -8.537024980200781389E-16 ) ) ;
#21799=ORIENTED_EDGE ( 'NONE', *, *, #8325, .T. ) ;
#21801=CIRCLE ( 'NONE', #6217, 0.2540000000000000036 ) ;
#21802=CARTESIAN_POINT ( 'NONE',  ( -58.37241122568488549, -0.2962816677227753104, -1.034007718770489626E-14 ) ) ;
#21805=CARTESIAN_POINT ( 'NONE',  ( -49.29989578322635424, 20.38947471906982756, 3.123819567266189257 ) ) ;
#21809=CARTESIAN_POINT ( 'NONE',  ( -51.10637697011796377, 21.44594517096482633, -1.085271236684668311E-14 ) ) ;
#21812=VERTEX_POINT ( 'NONE', #699 ) ;
#21820=DIRECTION ( 'NONE',  ( 5.188838149069472160E-16, -1.699382548006136559E-16, -1.000000000000000000 ) ) ;
#21832=CIRCLE ( 'NONE', #34120, 0.8889999999999977920 ) ;
#21842=DIRECTION ( 'NONE',  ( 0.7770581983690854067, -0.6294287539884012572, 5.101669463485840682E-16 ) ) ;
#21843=AXIS2_PLACEMENT_3D ( 'NONE', #41490, #36309, #2519 ) ;
#21850=DIRECTION ( 'NONE',  ( -0.9336303900108928744, -0.3582377630123714241, 0.000000000000000000 ) ) ;
#21852=CARTESIAN_POINT ( 'NONE',  ( -58.34786123531646496, -0.2455935055575208803, 0.1844583020148576336 ) ) ;
#21856=EDGE_CURVE ( 'NONE', #27727, #8502, #20334, .T. ) ;
#21857=AXIS2_PLACEMENT_3D ( 'NONE', #38096, #38514, #8911 ) ;
#21862=CARTESIAN_POINT ( 'NONE',  ( -48.59875010875282442, 18.41211343146811785, 5.165832069028382101 ) ) ;
#21866=CARTESIAN_POINT ( 'NONE',  ( -29.91360363449004822, 70.04874496952839991, 1.523999999999992250 ) ) ;
#21868=EDGE_LOOP ( 'NONE', ( #15009, #18176, #39692, #3098 ) ) ;
#21870=CARTESIAN_POINT ( 'NONE',  ( -29.22735587859570927, 60.46978361834971594, 1.523999999999994026 ) ) ;
#21871=DIRECTION ( 'NONE',  ( -5.188838149069471174E-16, 1.699382548006136313E-16, 1.000000000000000000 ) ) ;
#21873=DIRECTION ( 'NONE',  ( -0.9807655518882886225, 0.1951894777626621558, -5.420735302995426205E-16 ) ) ;
#21875=CARTESIAN_POINT ( 'NONE',  ( -17.31476582418722643, 62.07284264934779827, -1.269999999999999130 ) ) ;
#21885=CARTESIAN_POINT ( 'NONE',  ( -54.22787649382022579, 6.886497292746652121, 0.2709450413640898669 ) ) ;
#21894=ADVANCED_FACE ( 'NONE', ( #20251 ), #19836, .T. ) ;
#21899=CARTESIAN_POINT ( 'NONE',  ( -8.594951744493886991, 74.76616009375631222, -1.523999999999996913 ) ) ;
#21901=CIRCLE ( 'NONE', #5651, 0.6349999999999984546 ) ;
#21904=CARTESIAN_POINT ( 'NONE',  ( -46.92969783022256536, 25.19817632415814046, 1.844736899205347891 ) ) ;
#21905=CARTESIAN_POINT ( 'NONE',  ( -46.97515415817102280, 24.89137758704634962, 2.045406795549888468 ) ) ;
#21907=CARTESIAN_POINT ( 'NONE',  ( -46.97515415817095175, 24.89137758704647396, 2.045406795549891577 ) ) ;
#21919=CIRCLE ( 'NONE', #3598, 0.6350000000000014522 ) ;
#21920=CARTESIAN_POINT ( 'NONE',  ( -23.14542444889682216, 82.37908244650444090, 1.523999999999993582 ) ) ;
#21921=CARTESIAN_POINT ( 'NONE',  ( -17.64290547347870941, 83.78857423953914463, 1.269999999999996909 ) ) ;
#21922=DIRECTION ( 'NONE',  ( 5.188838149069472160E-16, -1.699382548006136559E-16, -1.000000000000000000 ) ) ;
#21925=EDGE_CURVE ( 'NONE', #4212, #11474, #23020, .T. ) ;
#21927=DIRECTION ( 'NONE',  ( -0.9876665170007974393, 0.1565721916417901483, -8.537024980200831679E-16 ) ) ;
#21931=ORIENTED_EDGE ( 'NONE', *, *, #27889, .T. ) ;
#21937=EDGE_LOOP ( 'NONE', ( #365, #40481, #39724, #3002 ) ) ;
#21940=DIRECTION ( 'NONE',  ( -0.8745520943968240202, 0.4849315768086551737, -5.361993529360572958E-16 ) ) ;
#21952=ORIENTED_EDGE ( 'NONE', *, *, #12295, .F. ) ;
#21964=AXIS2_PLACEMENT_3D ( 'NONE', #30827, #30409, #7429 ) ;
#21971=CARTESIAN_POINT ( 'NONE',  ( -16.02764313970815735, 80.34763903973272647, -1.524000000000002020 ) ) ;
#21974=DIRECTION ( 'NONE',  ( -5.188838149069472160E-16, 1.699382548006136559E-16, 1.000000000000000000 ) ) ;
#21975=CARTESIAN_POINT ( 'NONE',  ( -17.14500000000466784, 71.11999999999886768, -1.270000000000000684 ) ) ;
#21978=ORIENTED_EDGE ( 'NONE', *, *, #34186, .T. ) ;
#21979=CARTESIAN_POINT ( 'NONE',  ( -58.39046968809522298, 1.092456688167306567, -0.3056578461530352064 ) ) ;
#21981=CARTESIAN_POINT ( 'NONE',  ( -42.52099730114249354, 21.88661877469185413, -1.711735796961263656 ) ) ;
#21988=CARTESIAN_POINT ( 'NONE',  ( -53.83641692055964256, 9.560737412489993758, -3.788401990392710861 ) ) ;
#21989=AXIS2_PLACEMENT_3D ( 'NONE', #26108, #22262, #28886 ) ;
#21998=CARTESIAN_POINT ( 'NONE',  ( -49.66210360255988832, 16.76989353321783227, -4.946330335750499962 ) ) ;
#21999=CIRCLE ( 'NONE', #36291, 9.048749999999998295 ) ;
#22005=ADVANCED_FACE ( 'NONE', ( #12569 ), #14222, .T. ) ;
#22006=EDGE_CURVE ( 'NONE', #4510, #6464, #38054, .T. ) ;
#22013=DIRECTION ( 'NONE',  ( -0.9454731675810326141, 0.3256999990547876922, -8.537024980200857317E-16 ) ) ;
#22015=CARTESIAN_POINT ( 'NONE',  ( -41.98003980773050614, 22.15641273310255954, -0.9734550245785090761 ) ) ;
#22016=CARTESIAN_POINT ( 'NONE',  ( -17.76856900107737403, 61.81127730225986738, -1.269999999999999130 ) ) ;
#22017=CARTESIAN_POINT ( 'NONE',  ( -57.55343345497419705, 2.880119995625998630, 1.988856187846569146 ) ) ;
#22018=CARTESIAN_POINT ( 'NONE',  ( -50.74065386479207262, 15.09046855081605898, 4.756941196807721539 ) ) ;
#22020=AXIS2_PLACEMENT_3D ( 'NONE', #29084, #10124, #15663 ) ;
#22022=CARTESIAN_POINT ( 'NONE',  ( -52.32205026661357294, 13.67230311332622072, 4.407798173677520914 ) ) ;
#22025=CARTESIAN_POINT ( 'NONE',  ( -50.22242345129090779, 22.76272812237061771, -1.055084478852267100E-14 ) ) ;
#22028=ORIENTED_EDGE ( 'NONE', *, *, #6636, .T. ) ;
#22031=TOROIDAL_SURFACE ( 'NONE', #3709, 0.7620000000000000107, 0.2540000000000000036 ) ;
#22034=DIRECTION ( 'NONE',  ( 0.6294287539883864913, 0.7770581983690970640, 0.000000000000000000 ) ) ;
#22037=CARTESIAN_POINT ( 'NONE',  ( -29.89586364642802963, 71.55302121702176521, 1.523999999999992028 ) ) ;
#22041=CARTESIAN_POINT ( 'NONE',  ( -41.05189575270517821, 23.09451173561986792, -5.652993304041789371E-15 ) ) ;
#22054=EDGE_CURVE ( 'NONE', #35654, #30808, #39391, .T. ) ;
#22056=SHAPE_REPRESENTATION ( 'Wing Lever', ( #3275 ), #20939 ) ;
#22058=EDGE_CURVE ( 'NONE', #32447, #514, #1338, .T. ) ;
#22059=FACE_OUTER_BOUND ( 'NONE', #4807, .T. ) ;
#22060=ORIENTED_EDGE ( 'NONE', *, *, #30810, .T. ) ;
#22062=CARTESIAN_POINT ( 'NONE',  ( -17.64950171984354199, 84.16951713491046405, -1.524000000000003130 ) ) ;
#22069=CARTESIAN_POINT ( 'NONE',  ( -58.36037295411833981, -0.2718383842223853208, 0.1210796893238285932 ) ) ;
#22077=CARTESIAN_POINT ( 'NONE',  ( -29.10098582503172082, 61.33321833264426459, 1.523999999999993582 ) ) ;
#22079=ORIENTED_EDGE ( 'NONE', *, *, #37129, .F. ) ;
#22082=CYLINDRICAL_SURFACE ( 'NONE', #16032, 0.2539999999999989488 ) ;
#22083=DIRECTION ( 'NONE',  ( -0.8745520943968244643, 0.4849315768086544520, -4.268512490100399076E-16 ) ) ;
#22086=FACE_OUTER_BOUND ( 'NONE', #34225, .T. ) ;
#22095=CARTESIAN_POINT ( 'NONE',  ( -56.89469692534096623, 2.545995565645275960, 0.6470027801917009880 ) ) ;
#22102=EDGE_LOOP ( 'NONE', ( #6773, #12135, #31287, #23840 ) ) ;
#22108=DIRECTION ( 'NONE',  ( -5.188838149069471174E-16, 1.699382548006136313E-16, 1.000000000000000000 ) ) ;
#22109=CARTESIAN_POINT ( 'NONE',  ( -6.422645615570758970, 77.88548590848095898, 1.270000000000003570 ) ) ;
#22110=CARTESIAN_POINT ( 'NONE',  ( -46.60530155212501313, 26.17382724835480445, 0.08466666666665845220 ) ) ;
#22112=CARTESIAN_POINT ( 'NONE',  ( -48.08949201794742834, 19.91830422262442468, 5.194343260851632671 ) ) ;
#22113=DIRECTION ( 'NONE',  ( 0.6294287539884059202, 0.7770581983690814099, 1.945484789722797322E-16 ) ) ;
#22116=ORIENTED_EDGE ( 'NONE', *, *, #18922, .T. ) ;
#22125=DIRECTION ( 'NONE',  ( -5.188838149069472160E-16, 1.699382548006136559E-16, 1.000000000000000000 ) ) ;
#22130=CIRCLE ( 'NONE', #40538, 0.3810000000000000053 ) ;
#22141=CARTESIAN_POINT ( 'NONE',  ( -47.85244527695891037, 19.39403540832952544, -5.219971639306605127 ) ) ;
#22148=CARTESIAN_POINT ( 'NONE',  ( -17.14500000000466784, 71.11999999999886768, 1.269999999999998241 ) ) ;
#22153=VERTEX_POINT ( 'NONE', #7241 ) ;
#22155=DIRECTION ( 'NONE',  ( -0.7548010569845247097, -0.6559537821943284275, -7.865859715776929025E-15 ) ) ;
#22156=DIRECTION ( 'NONE',  ( -0.1565721916418019999, -0.9876665170007956629, 8.659954811667593930E-17 ) ) ;
#22157=CARTESIAN_POINT ( 'NONE',  ( -58.62613161866106282, -0.2841797903858078733, 0.3870556671707012786 ) ) ;
#22159=VECTOR ( 'NONE', #28210, 1000.000000000000114 ) ;
#22162=DIRECTION ( 'NONE',  ( -5.188838149069472160E-16, 1.699382548006136559E-16, 1.000000000000000000 ) ) ;
#22165=FACE_OUTER_BOUND ( 'NONE', #8815, .T. ) ;
#22166=CARTESIAN_POINT ( 'NONE',  ( -16.02764313970815735, 80.34763903973272647, -1.524000000000002020 ) ) ;
#22172=LINE ( 'NONE', #19823, #10780 ) ;
#22176=DIRECTION ( 'NONE',  ( -0.8745520943968235761, 0.4849315768086558398, -4.268512490100410909E-16 ) ) ;
#22178=EDGE_CURVE ( 'NONE', #41065, #36274, #9499, .T. ) ;
#22182=DIRECTION ( 'NONE',  ( 0.01731298258488817021, -0.9998501190848633202, -2.778415991487942562E-15 ) ) ;
#22190=CIRCLE ( 'NONE', #34443, 3.111499999999999932 ) ;
#22191=CARTESIAN_POINT ( 'NONE',  ( -56.36817218596900148, 4.518355621917047316, -2.583766698011176199 ) ) ;
#22193=CARTESIAN_POINT ( 'NONE',  ( -58.44182880578510009, -0.4131463110827765517, -0.3217794782792326447 ) ) ;
#22198=DIRECTION ( 'NONE',  ( -5.188838149069472160E-16, 1.699382548006136559E-16, 1.000000000000000000 ) ) ;
#22201=CARTESIAN_POINT ( 'NONE',  ( -52.06546789126484498, 13.38259882428268632, -4.575081192416392106 ) ) ;
#22203=ORIENTED_EDGE ( 'NONE', *, *, #23185, .T. ) ;
#22207=AXIS2_PLACEMENT_3D ( 'NONE', #40732, #18126, #41151 ) ;
#22215=CARTESIAN_POINT ( 'NONE',  ( -25.70569512491730180, 74.05161654054386133, 1.269999999999993356 ) ) ;
#22217=CARTESIAN_POINT ( 'NONE',  ( -47.34044527953909665, 17.31523404052589399, -1.593293138114936891 ) ) ;
#22218=ORIENTED_EDGE ( 'NONE', *, *, #26331, .T. ) ;
#22221=PLANE ( 'NONE',  #33610 ) ;
#22222=CARTESIAN_POINT ( 'NONE',  ( -53.41021539168369969, 10.36760520877136038, 3.951087388861569405 ) ) ;
#22223=CARTESIAN_POINT ( 'NONE',  ( -29.88458269572754133, 69.13647124298606172, -1.523999999995101273 ) ) ;
#22225=CARTESIAN_POINT ( 'NONE',  ( -57.43227285409300009, 3.226759729073131133, 2.064049688025078488 ) ) ;
#22227=VERTEX_POINT ( 'NONE', #14234 ) ;
#22228=CARTESIAN_POINT ( 'NONE',  ( -53.04800011033383811, 17.61732480341419915, -0.3294858417196845357 ) ) ;
#22230=ADVANCED_FACE ( 'NONE', ( #21244 ), #4474, .T. ) ;
#22237=DIRECTION ( 'NONE',  ( -0.9336303900108801068, -0.3582377630124047307, 1.771430154111087713E-15 ) ) ;
#22240=ADVANCED_FACE ( 'NONE', ( #30223 ), #7165, .T. ) ;
#22250=CARTESIAN_POINT ( 'NONE',  ( -58.36579948110144045, -0.2832072201896413954, -0.07825354645670587472 ) ) ;
#22262=DIRECTION ( 'NONE',  ( -5.188838149069472160E-16, 1.699382548006136559E-16, 1.000000000000000000 ) ) ;
#22263=CARTESIAN_POINT ( 'NONE',  ( -45.14658554404967106, 22.88857079803865346, -2.562886992506571371 ) ) ;
#22268=DIRECTION ( 'NONE',  ( -0.8745520943968243532, 0.4849315768086547296, -6.829619984160642269E-16 ) ) ;
#22274=LINE ( 'NONE', #42121, #9069 ) ;
#22275=CARTESIAN_POINT ( 'NONE',  ( -58.36935479428260010, -0.2906258791830944599, 0.02610806206428318774 ) ) ;
#22279=CARTESIAN_POINT ( 'NONE',  ( -23.94760723868026631, 77.08694321397520355, -1.524000000000005350 ) ) ;
#22286=CARTESIAN_POINT ( 'NONE',  ( -29.20122892428398487, 63.96733531828105157, 1.523999999999130495 ) ) ;
#22288=CARTESIAN_POINT ( 'NONE',  ( -43.16005656664477641, 21.89413631511959579, 2.197846903551415654 ) ) ;
#22291=( BOUNDED_CURVE ( )  B_SPLINE_CURVE ( 2, ( #18814, #31823, #27575 ),
 .UNSPECIFIED., .F., .T. ) 
 B_SPLINE_CURVE_WITH_KNOTS ( ( 3, 3 ),
 ( 0.000000000000000000, 1.000000000000000000 ),
 .UNSPECIFIED. ) 
 CURVE ( )  GEOMETRIC_REPRESENTATION_ITEM ( )  RATIONAL_B_SPLINE_CURVE ( ( 1.000000000000000000, 0.9987193938133603899, 1.000000000000000000 ) ) 
 REPRESENTATION_ITEM ( '' )  );
#22294=CARTESIAN_POINT ( 'NONE',  ( -52.02227077090995522, 12.92666902011463392, -4.429676403366612725 ) ) ;
#22300=MECHANICAL_DESIGN_GEOMETRIC_PRESENTATION_REPRESENTATION('',(#28430),#19562);
#22307=ORIENTED_EDGE ( 'NONE', *, *, #34392, .F. ) ;
#22315=CARTESIAN_POINT ( 'NONE',  ( -42.72397600927682504, 22.83316142988638831, 1.683267422954620063 ) ) ;
#22316=CARTESIAN_POINT ( 'NONE',  ( -46.81005371095113077, 25.73327194510126859, 1.583310528698469222 ) ) ;
#22318=CARTESIAN_POINT ( 'NONE',  ( -48.53848336910535011, 19.22582880449973075, 5.323527254358031868 ) ) ;
#22319=CARTESIAN_POINT ( 'NONE',  ( -58.67289155984229865, -0.3138610667730852843, 0.3158150924223985800 ) ) ;
#22324=AXIS2_PLACEMENT_3D ( 'NONE', #38017, #28426, #28847 ) ;
#22336=DIRECTION ( 'NONE',  ( 0.3582377630123966261, -0.9336303900108832154, 0.000000000000000000 ) ) ;
#22356=CARTESIAN_POINT ( 'NONE',  ( -48.27157819694446061, 19.62644098948943494, -5.255994444853051561 ) ) ;
#22360=ORIENTED_EDGE ( 'NONE', *, *, #41501, .T. ) ;
#22362=AXIS2_PLACEMENT_3D ( 'NONE', #33587, #39558, #794 ) ;
#22363=DIRECTION ( 'NONE',  ( -0.2883665106726556182, -0.9575201071113218498, -1.655452583021194521E-15 ) ) ;
#22371=CARTESIAN_POINT ( 'NONE',  ( -15.27962295839633811, 80.49293118800726177, 1.269999999999997797 ) ) ;
#22378=DIRECTION ( 'NONE',  ( 5.188838149069472160E-16, -1.699382548006136559E-16, -1.000000000000000000 ) ) ;
#22389=CIRCLE ( 'NONE', #23096, 0.5080000000000000071 ) ;
#22391=DIRECTION ( 'NONE',  ( -5.188838149069472160E-16, 1.699382548006136559E-16, 1.000000000000000000 ) ) ;
#22392=VECTOR ( 'NONE', #2944, 1000.000000000000000 ) ;
#22399=CARTESIAN_POINT ( 'NONE',  ( -57.60174957807323892, 1.918618717652168737, -1.731152311951061229 ) ) ;
#22401=CARTESIAN_POINT ( 'NONE',  ( -58.34279097978634354, -0.2008976519087390666, -0.5874393231861719800 ) ) ;
#22405=DIRECTION ( 'NONE',  ( -0.8745520943968240202, 0.4849315768086553402, -5.361993529360572958E-16 ) ) ;
#22409=ORIENTED_EDGE ( 'NONE', *, *, #17977, .T. ) ;
#22415=ADVANCED_FACE ( 'NONE', ( #5729 ), #18259, .T. ) ;
#22420=CARTESIAN_POINT ( 'NONE',  ( -46.72577905453591285, 25.95655153957432049, 1.270000040520065099 ) ) ;
#22423=DIRECTION ( 'NONE',  ( -0.9336303900108815501, -0.3582377630124009560, -4.235673982319039874E-16 ) ) ;
#22424=CARTESIAN_POINT ( 'NONE',  ( -49.96466797210978683, 13.31430344189337589, -0.7651684107025076287 ) ) ;
#22428=CARTESIAN_POINT ( 'NONE',  ( -55.32540223338650520, 6.651447249606684764, 3.145907943678666996 ) ) ;
#22430=CARTESIAN_POINT ( 'NONE',  ( -26.07365872405947727, 72.73903180058835005, 1.269999999999993356 ) ) ;
#22431=CARTESIAN_POINT ( 'NONE',  ( -54.68491514712287227, 9.937145987696780480, 2.757516356780029820 ) ) ;
#22433=VERTEX_POINT ( 'NONE', #28069 ) ;
#22434=CARTESIAN_POINT ( 'NONE',  ( -51.68405183839315242, 20.46365084185837446, -0.3671080129529064595 ) ) ;
#22436=VERTEX_POINT ( 'NONE', #2320 ) ;
#22438=VECTOR ( 'NONE', #30244, 1000.000000000000000 ) ;
#22453=ORIENTED_EDGE ( 'NONE', *, *, #6035, .F. ) ;
#22454=CARTESIAN_POINT ( 'NONE',  ( -58.33566222542154378, -0.2199106620376253540, -0.2319731289860410273 ) ) ;
#22460=DIRECTION ( 'NONE',  ( -5.188838149069472160E-16, 1.699382548006136559E-16, 1.000000000000000000 ) ) ;
#22462=EDGE_CURVE ( 'NONE', #25690, #33817, #5437, .T. ) ;
#22463=ADVANCED_FACE ( 'NONE', ( #35110 ), #34898, .T. ) ;
#22466=CARTESIAN_POINT ( 'NONE',  ( -4.476425760464393555, 71.61790547347303004, 1.524000000000005128 ) ) ;
#22468=CARTESIAN_POINT ( 'NONE',  ( -46.89970385779243855, 22.02655025333852379, -4.237790764466935478 ) ) ;
#22469=VERTEX_POINT ( 'NONE', #28908 ) ;
#22473=EDGE_CURVE ( 'NONE', #41900, #39553, #22918, .T. ) ;
#22477=EDGE_CURVE ( 'NONE', #23676, #24684, #16303, .T. ) ;
#22484=ADVANCED_FACE ( 'NONE', ( #29336 ), #2029, .T. ) ;
#22485=ORIENTED_EDGE ( 'NONE', *, *, #38388, .T. ) ;
#22490=FACE_OUTER_BOUND ( 'NONE', #21111, .T. ) ;
#22491=VECTOR ( 'NONE', #24224, 1000.000000000000114 ) ;
#22505=VECTOR ( 'NONE', #15985, 1000.000000000000227 ) ;
#22515=VERTEX_POINT ( 'NONE', #19316 ) ;
#22519=CIRCLE ( 'NONE', #35489, 0.2539999999999942859 ) ;
#22521=EDGE_CURVE ( 'NONE', #41900, #10652, #42157, .T. ) ;
#22525=AXIS2_PLACEMENT_3D ( 'NONE', #41945, #16779, #15931 ) ;
#22526=CARTESIAN_POINT ( 'NONE',  ( -51.80188483046436687, 13.03002009012210927, 4.294765137396908017 ) ) ;
#22527=CARTESIAN_POINT ( 'NONE',  ( -46.98785713747574277, 25.41845405000909253, 0.7790854875835052651 ) ) ;
#22530=CARTESIAN_POINT ( 'NONE',  ( -48.59875010875282442, 18.41211343146811785, 5.165832069028382101 ) ) ;
#22531=CARTESIAN_POINT ( 'NONE',  ( -10.84307050033138431, 78.30450799593342026, -1.523999999999998911 ) ) ;
#22533=CARTESIAN_POINT ( 'NONE',  ( -58.20750686534850615, 0.04498437427168100466, -0.4973296020553497065 ) ) ;
#22536=CARTESIAN_POINT ( 'NONE',  ( -41.23752580366542020, 23.26788267949596190, -1.524000000000005128 ) ) ;
#22549=DIRECTION ( 'NONE',  ( 0.8745520943968236871, -0.4849315768086559508, 6.829619984160659032E-16 ) ) ;
#22553=LINE ( 'NONE', #35583, #12457 ) ;
#22557=CIRCLE ( 'NONE', #8968, 0.2539999999999966729 ) ;
#22560=ORIENTED_EDGE ( 'NONE', *, *, #7974, .F. ) ;
#22561=CARTESIAN_POINT ( 'NONE',  ( -47.40532530373579334, 16.48158934372809270, 0.7854836779715855810 ) ) ;
#22575=CARTESIAN_POINT ( 'NONE',  ( -58.50248613193047476, -0.02569321026645032813, 0.6864972099047519372 ) ) ;
#22599=VERTEX_POINT ( 'NONE', #32970 ) ;
#22607=CARTESIAN_POINT ( 'NONE',  ( -53.82649921536103221, 9.579626810350022836, -3.792271429080182887 ) ) ;
#22609=CARTESIAN_POINT ( 'NONE',  ( -58.45963793110830409, -0.4469582673305985687, -0.3141006534898306835 ) ) ;
#22612=DIRECTION ( 'NONE',  ( 0.6294287539884133587, 0.7770581983690755257, 0.000000000000000000 ) ) ;
#22615=CARTESIAN_POINT ( 'NONE',  ( -58.70413935429054675, 0.2332485698458008905, -0.6626129746612972049 ) ) ;
#22616=CIRCLE ( 'NONE', #28080, 0.2540000000000000036 ) ;
#22620=ORIENTED_EDGE ( 'NONE', *, *, #36960, .F. ) ;
#22625=CARTESIAN_POINT ( 'NONE',  ( -55.83515739322318439, 4.224161455597882586, -1.000857388952954637E-14 ) ) ;
#22628=CARTESIAN_POINT ( 'NONE',  ( -46.60530155212504155, 26.17382724835478314, 1.523999999999996913 ) ) ;
#22631=CARTESIAN_POINT ( 'NONE',  ( -50.15972161391664486, 17.13814111569220699, -4.955022299345085202 ) ) ;
#22632=CARTESIAN_POINT ( 'NONE',  ( -48.16508968810063607, 19.01313136326714925, -5.219744232931994965 ) ) ;
#22633=LINE ( 'NONE', #35670, #2650 ) ;
#22635=CARTESIAN_POINT ( 'NONE',  ( -46.65118376738641359, 26.08833806145381473, -1.300560147374372866 ) ) ;
#22636=CARTESIAN_POINT ( 'NONE',  ( -48.78337893976456030, 18.15300145085139860, 5.151671844828033642 ) ) ;
#22639=LINE ( 'NONE', #35675, #5577 ) ;
#22640=CARTESIAN_POINT ( 'NONE',  ( -55.45615287082594591, 8.171946630687445534, 2.478682617993481774 ) ) ;
#22641=CARTESIAN_POINT ( 'NONE',  ( -57.81953393267934160, 1.609514594907199392, 1.636666387507130782 ) ) ;
#22644=VERTEX_POINT ( 'NONE', #15908 ) ;
#22646=CARTESIAN_POINT ( 'NONE',  ( -55.24575511360421842, 11.19612964283526324, -0.2458718103055786974 ) ) ;
#22665=CARTESIAN_POINT ( 'NONE',  ( -58.31002553906358798, -0.1654322197361378644, -0.3101674830710153818 ) ) ;
#22677=CIRCLE ( 'NONE', #21312, 0.2540000000000051106 ) ;
#22680=CARTESIAN_POINT ( 'NONE',  ( -44.55074271434504851, 21.27721161058206789, -3.389857510897070547 ) ) ;
#22688=EDGE_CURVE ( 'NONE', #20108, #16766, #29892, .T. ) ;
#22690=DIRECTION ( 'NONE',  ( 5.188838149069472160E-16, -1.699382548006136559E-16, -1.000000000000000000 ) ) ;
#22691=AXIS2_PLACEMENT_3D ( 'NONE', #33923, #1555, #4754 ) ;
#22692=AXIS2_PLACEMENT_3D ( 'NONE', #19122, #9340, #28718 ) ;
#22714=CARTESIAN_POINT ( 'NONE',  ( -50.04979780823605751, 16.23027998585079601, -4.918765685689631795 ) ) ;
#22732=CARTESIAN_POINT ( 'NONE',  ( -47.01067208220106863, 24.90190543975541360, 1.870441909736396902 ) ) ;
#22734=CARTESIAN_POINT ( 'NONE',  ( -47.43570116002442205, 20.37060963802031566, 5.342502768866032703 ) ) ;
#22735=DIRECTION ( 'NONE',  ( -0.8745520943968250194, 0.4849315768086535083, -5.424246918827963022E-16 ) ) ;
#22738=EDGE_CURVE ( 'NONE', #6546, #39412, #23773, .T. ) ;
#22741=FACE_OUTER_BOUND ( 'NONE', #19621, .T. ) ;
#22749=DIRECTION ( 'NONE',  ( 0.6559537821943243197, -0.7548010569845282625, 8.537024980200743918E-16 ) ) ;
#22750=LINE ( 'NONE', #2994, #10388 ) ;
#22759=VERTEX_POINT ( 'NONE', #37002 ) ;
#22765=ADVANCED_FACE ( 'NONE', ( #40615 ), #16965, .T. ) ;
#22769=CARTESIAN_POINT ( 'NONE',  ( -42.01646181069634878, 22.10209156318453694, 0.7046475714187654393 ) ) ;
#22777=CARTESIAN_POINT ( 'NONE',  ( -48.16862273754407653, 19.56935307722002193, -5.361094314902742575 ) ) ;
#22782=CYLINDRICAL_SURFACE ( 'NONE', #3425, 0.6350000000000014522 ) ;
#22783=CARTESIAN_POINT ( 'NONE',  ( -26.07955644221209113, 72.55303096390359485, 1.269999999999993356 ) ) ;
#22784=CARTESIAN_POINT ( 'NONE',  ( -58.82993853617183788, -0.2576789964694181645, 0.02280678270975886393 ) ) ;
#22808=ORIENTED_EDGE ( 'NONE', *, *, #6349, .F. ) ;
#22813=ADVANCED_FACE ( 'NONE', ( #4844 ), #1229, .F. ) ;
#22825=CARTESIAN_POINT ( 'NONE',  ( -58.60752282809816904, -0.1920500713008393978, -0.6598870774482961110 ) ) ;
#22837=CARTESIAN_POINT ( 'NONE',  ( -46.70722035912341141, 25.99002130462735849, 1.524000028476692359 ) ) ;
#22840=DIRECTION ( 'NONE',  ( -5.188838149069471174E-16, 1.699382548006136313E-16, 1.000000000000000000 ) ) ;
#22841=CARTESIAN_POINT ( 'NONE',  ( -48.19617591663109124, 18.61566378669634503, -4.750300018642161781 ) ) ;
#22844=CARTESIAN_POINT ( 'NONE',  ( -46.61813330717926362, 26.15088526608503372, -1.277411791215423031 ) ) ;
#22845=DIRECTION ( 'NONE',  ( -0.4849315768086535083, -0.8745520943968250194, -1.030032898892974695E-16 ) ) ;
#22850=CARTESIAN_POINT ( 'NONE',  ( -57.35225397299146977, 4.112755766825001658, 0.3099640861128158398 ) ) ;
#22851=CIRCLE ( 'NONE', #26278, 0.2540000000000029456 ) ;
#22852=CARTESIAN_POINT ( 'NONE',  ( -57.43854689232674815, 1.757847328446624058, 1.624773336220232789 ) ) ;
#22854=AXIS2_PLACEMENT_3D ( 'NONE', #39489, #36299, #17517 ) ;
#22855=ORIENTED_EDGE ( 'NONE', *, *, #28953, .T. ) ;
#22856=CARTESIAN_POINT ( 'NONE',  ( -53.65397596840620764, 15.31786685697163897, -0.6615342354324158514 ) ) ;
#22857=AXIS2_PLACEMENT_3D ( 'NONE', #14064, #30052, #889 ) ;
#22860=DIRECTION ( 'NONE',  ( -5.188838149069472160E-16, 1.699382548006136559E-16, 1.000000000000000000 ) ) ;
#22874=ORIENTED_EDGE ( 'NONE', *, *, #38086, .T. ) ;
#22875=CARTESIAN_POINT ( 'NONE',  ( -58.36964224452065508, -0.2912198378497423135, -0.01722170194331728438 ) ) ;
#22888=TOROIDAL_SURFACE ( 'NONE', #17462, 3.111499999999999488, 0.2540000000000000036 ) ;
#22889=CARTESIAN_POINT ( 'NONE',  ( -37.66124916107632714, 74.02712188174415076, 1.523999999999987587 ) ) ;
#22890=CARTESIAN_POINT ( 'NONE',  ( -48.38589991294941939, 19.15920805527091630, -5.452675306770326635 ) ) ;
#22891=AXIS2_PLACEMENT_3D ( 'NONE', #39659, #32841, #13872 ) ;
#22892=ORIENTED_EDGE ( 'NONE', *, *, #12395, .F. ) ;
#22901=CARTESIAN_POINT ( 'NONE',  ( -30.75918919842648336, 69.77432548395512413, -1.524000000000007793 ) ) ;
#22902=CIRCLE ( 'NONE', #33828, 9.048749999999998295 ) ;
#22903=EDGE_CURVE ( 'NONE', #38897, #6194, #14259, .T. ) ;
#22911=DIRECTION ( 'NONE',  ( -0.3256999990547897461, -0.9454731675810318370, 0.000000000000000000 ) ) ;
#22914=EDGE_LOOP ( 'NONE', ( #12946, #38564, #10568, #38128 ) ) ;
#22917=DIRECTION ( 'NONE',  ( 0.3582377630123916856, -0.9336303900108853249, 3.445432962228668055E-16 ) ) ;
#22918=LINE ( 'NONE', #9740, #22392 ) ;
#22919=CIRCLE ( 'NONE', #39969, 0.2539999999999975056 ) ;
#22923=CARTESIAN_POINT ( 'NONE',  ( -48.16232371146166003, 19.02200717996782586, -5.227009030934667955 ) ) ;
#22924=DIRECTION ( 'NONE',  ( -5.188838149069472160E-16, 1.699382548006136559E-16, 1.000000000000000000 ) ) ;
#22928=ORIENTED_EDGE ( 'NONE', *, *, #16805, .F. ) ;
#22932=LINE ( 'NONE', #3597, #24078 ) ;
#22941=EDGE_CURVE ( 'NONE', #21011, #29590, #7821, .T. ) ;
#22945=CARTESIAN_POINT ( 'NONE',  ( -46.74369117050184741, 25.88875364612797725, 1.392958786023526185 ) ) ;
#22946=CARTESIAN_POINT ( 'NONE',  ( -49.37240900658670739, 23.24656341648388036, 0.6295958749597029280 ) ) ;
#22948=EDGE_CURVE ( 'NONE', #17342, #41432, #24400, .T. ) ;
#22949=CARTESIAN_POINT ( 'NONE',  ( -56.21344593158320180, 5.939860726778031896, 2.828251681716853927 ) ) ;
#22950=CARTESIAN_POINT ( 'NONE',  ( -58.81783741892115103, -0.2724193165228563362, 0.09424156098961072869 ) ) ;
#22952=CARTESIAN_POINT ( 'NONE',  ( -58.37241122568488549, -0.2962816677227891882, -1.026553828834651941E-14 ) ) ;
#22953=VERTEX_POINT ( 'NONE', #13982 ) ;
#22959=CARTESIAN_POINT ( 'NONE',  ( -46.95726096424718321, 25.94444535518948669, -0.08936005021616608146 ) ) ;
#22962=CARTESIAN_POINT ( 'NONE',  ( -14.53564353655538000, 79.78436006922240153, -1.524000000000001132 ) ) ;
#22972=CARTESIAN_POINT ( 'NONE',  ( -17.14500000000466784, 71.11999999999886768, -1.270000000000000684 ) ) ;
#22977=AXIS2_PLACEMENT_3D ( 'NONE', #37639, #21842, #21631 ) ;
#22979=ORIENTED_EDGE ( 'NONE', *, *, #27378, .T. ) ;
#22980=ADVANCED_FACE ( 'NONE', ( #10582 ), #20783, .F. ) ;
#22981=ORIENTED_EDGE ( 'NONE', *, *, #26007, .T. ) ;
#22982=CARTESIAN_POINT ( 'NONE',  ( -45.23155955595164812, 20.39474799592974463, 2.956275845755106157 ) ) ;
#22989=DIRECTION ( 'NONE',  ( 5.188838149069472160E-16, -1.699382548006136559E-16, -1.000000000000000000 ) ) ;
#22993=ORIENTED_EDGE ( 'NONE', *, *, #28269, .T. ) ;
#22994=CARTESIAN_POINT ( 'NONE',  ( -10.00099186598785650, 77.19260062651656540, 1.270000000000000684 ) ) ;
#23011=LINE ( 'NONE', #41816, #18239 ) ;
#23020=LINE ( 'NONE', #2683, #35983 ) ;
#23022=LINE ( 'NONE', #28600, #14779 ) ;
#23024=CARTESIAN_POINT ( 'NONE',  ( -30.20416046766209561, 71.17241488000101413, 1.523999999999992028 ) ) ;
#23029=CARTESIAN_POINT ( 'NONE',  ( -58.76039124197362185, -0.3072667177839057961, -0.2129973275852694858 ) ) ;
#23030=ORIENTED_EDGE ( 'NONE', *, *, #39363, .T. ) ;
#23031=CARTESIAN_POINT ( 'NONE',  ( -25.77058783747419213, 72.83664265955201245, 1.523999999999993804 ) ) ;
#23035=CARTESIAN_POINT ( 'NONE',  ( -43.55282894732439303, 21.75186528800919916, 2.470256908105690652 ) ) ;
#23037=AXIS2_PLACEMENT_3D ( 'NONE', #15787, #25796, #29419 ) ;
#23039=CARTESIAN_POINT ( 'NONE',  ( -57.71946847630993460, 1.146847591362354368, -1.351507486235954403 ) ) ;
#23051=ADVANCED_FACE ( 'NONE', ( #28237 ), #40794, .T. ) ;
#23055=AXIS2_PLACEMENT_3D ( 'NONE', #1276, #4264, #23608 ) ;
#23056=CARTESIAN_POINT ( 'NONE',  ( -48.50421218116025557, 14.67712143704001626, -8.170758227952415863E-15 ) ) ;
#23057=AXIS2_PLACEMENT_3D ( 'NONE', #33902, #36675, #23870 ) ;
#23059=DIRECTION ( 'NONE',  ( 2.731847993664264244E-14, -1.365923996832132122E-14, 1.000000000000000000 ) ) ;
#23061=CARTESIAN_POINT ( 'NONE',  ( -30.15519950990045572, 69.97033940222175374, -1.270000000000007123 ) ) ;
#23065=CARTESIAN_POINT ( 'NONE',  ( -8.584014518950162653, 73.13423810798757074, 1.270000000000002460 ) ) ;
#23066=CARTESIAN_POINT ( 'NONE',  ( -56.90927647567382763, 5.206763508130138440, 0.7605795637954813060 ) ) ;
#23067=CARTESIAN_POINT ( 'NONE',  ( -56.65231406860745977, 4.194353530936431262, 2.518504496425231221 ) ) ;
#23070=CARTESIAN_POINT ( 'NONE',  ( -51.08083271936510528, 17.88738476406025057, -2.973263991802298278 ) ) ;
#23089=CARTESIAN_POINT ( 'NONE',  ( -58.36967811586515609, -0.2912949152869354075, -0.01564362208030510917 ) ) ;
#23096=AXIS2_PLACEMENT_3D ( 'NONE', #15983, #25785, #19391 ) ;
#23101=VECTOR ( 'NONE', #35069, 1000.000000000000227 ) ;
#23103=CARTESIAN_POINT ( 'NONE',  ( -14.38915334913366983, 80.27078028363496287, 1.269999999999998019 ) ) ;
#23104=CARTESIAN_POINT ( 'NONE',  ( -46.25688858429101202, 20.73875112231587892, -4.700046123029353318 ) ) ;
#23107=CARTESIAN_POINT ( 'NONE',  ( -16.71197878298170991, 83.87086364642222236, -1.524000000000002686 ) ) ;
#23112=DIRECTION ( 'NONE',  ( 0.8745520943968249084, -0.4849315768086533418, 5.271987356194193006E-16 ) ) ;
#23113=FACE_OUTER_BOUND ( 'NONE', #20049, .T. ) ;
#23115=EDGE_LOOP ( 'NONE', ( #5124, #41976, #32331, #23984 ) ) ;
#23121=CARTESIAN_POINT ( 'NONE',  ( -33.20758249455312239, 49.81222039523557044, 1.523999999999993804 ) ) ;
#23127=CARTESIAN_POINT ( 'NONE',  ( -6.135835944515187101, 77.40800365160224317, -1.269999999999996243 ) ) ;
#23131=DIRECTION ( 'NONE',  ( -0.5149185422762221354, 0.8572391118119440101, -4.128606161907601007E-16 ) ) ;
#23136=ORIENTED_EDGE ( 'NONE', *, *, #31794, .T. ) ;
#23141=CARTESIAN_POINT ( 'NONE',  ( -18.88948446928058544, 80.17638627449419175, -1.524000000000003352 ) ) ;
#23145=DIRECTION ( 'NONE',  ( -0.9998501190848636533, -0.01731298258487451447, -5.158639060800524920E-16 ) ) ;
#23149=EDGE_CURVE ( 'NONE', #5536, #4600, #41470, .T. ) ;
#23153=CARTESIAN_POINT ( 'NONE',  ( -50.65446802363735657, 15.06743570032490176, 4.641860962342715169 ) ) ;
#23154=CARTESIAN_POINT ( 'NONE',  ( -50.95401362087786623, 21.69085173448186055, 0.3723302588259275736 ) ) ;
#23157=CARTESIAN_POINT ( 'NONE',  ( -48.65005484009959957, 18.46594748123760965, 5.297328305960426142 ) ) ;
#23162=ORIENTED_EDGE ( 'NONE', *, *, #3533, .T. ) ;
#23163=CARTESIAN_POINT ( 'NONE',  ( -42.72397600927682504, 22.83316142988638831, 1.683267422954620063 ) ) ;
#23175=DIRECTION ( 'NONE',  ( -0.6675346791887244446, 0.7445787077807199950, 3.626530295975567369E-14 ) ) ;
#23179=CARTESIAN_POINT ( 'NONE',  ( -5.719305292821792008, 76.92870498041706639, -1.269999999999995799 ) ) ;
#23185=EDGE_CURVE ( 'NONE', #1265, #26041, #21398, .T. ) ;
#23186=ORIENTED_EDGE ( 'NONE', *, *, #39378, .T. ) ;
#23187=CARTESIAN_POINT ( 'NONE',  ( -45.58494389689082738, 18.10922195552005221, 0.2974575429725789255 ) ) ;
#23203=LINE ( 'NONE', #7058, #22505 ) ;
#23205=CARTESIAN_POINT ( 'NONE',  ( -29.81357423954495189, 70.62209452652477637, 1.269999999999991802 ) ) ;
#23208=CIRCLE ( 'NONE', #39582, 0.2539999999999998925 ) ;
#23209=DIRECTION ( 'NONE',  ( -5.188838149069472160E-16, 1.699382548006136559E-16, 1.000000000000000000 ) ) ;
#23224=CARTESIAN_POINT ( 'NONE',  ( -47.35944255389382107, 21.37623662739424191, -4.722871667523179440 ) ) ;
#23225=DIRECTION ( 'NONE',  ( -0.1565721916418034432, -0.9876665170007953298, 8.659954811667511346E-17 ) ) ;
#23230=ORIENTED_EDGE ( 'NONE', *, *, #36703, .F. ) ;
#23231=DIRECTION ( 'NONE',  ( -0.8745520943968243532, 0.4849315768086547296, -6.829619984160642269E-16 ) ) ;
#23239=CARTESIAN_POINT ( 'NONE',  ( -58.62437260890455093, -0.2808582271535189356, -0.3920676774944526488 ) ) ;
#23241=FACE_OUTER_BOUND ( 'NONE', #20482, .T. ) ;
#23248=CARTESIAN_POINT ( 'NONE',  ( -58.43690671596436914, -0.4125963578781866037, -1.035377653829272970E-14 ) ) ;
#23249=ADVANCED_FACE ( 'NONE', ( #8861 ), #31857, .T. ) ;
#23253=ORIENTED_EDGE ( 'NONE', *, *, #19933, .F. ) ;
#23258=CARTESIAN_POINT ( 'NONE',  ( -58.33992048227231209, -0.2288887037933118318, 0.2155571079148066727 ) ) ;
#23264=LINE ( 'NONE', #33734, #39219 ) ;
#23266=CARTESIAN_POINT ( 'NONE',  ( -53.95448410595108157, 8.335714161839828051, -2.220323970834214844 ) ) ;
#23269=DIRECTION ( 'NONE',  ( -0.1906721105965040186, 0.9816537812491095139, -2.657572025465703189E-16 ) ) ;
#23271=CARTESIAN_POINT ( 'NONE',  ( -6.194847070882102180, 64.72978607931611350, -1.269999999999994023 ) ) ;
#23275=CARTESIAN_POINT ( 'NONE',  ( -58.21785149106106871, 1.559091779220117546, 0.3785645914142855561 ) ) ;
#23276=CARTESIAN_POINT ( 'NONE',  ( -57.80205714066466527, 2.371715784325115095, 1.753227392946289598 ) ) ;
#23280=CARTESIAN_POINT ( 'NONE',  ( -57.84788464146735265, 2.520999533240836143, -0.7145982302433674382 ) ) ;
#23288=CIRCLE ( 'NONE', #36243, 0.2539999999999962288 ) ;
#23291=CARTESIAN_POINT ( 'NONE',  ( -29.26089923143846860, 65.68766220334288164, 1.269999999999992912 ) ) ;
#23295=DIRECTION ( 'NONE',  ( -0.3256999990547864710, -0.9454731675810330582, 1.399154850856895850E-16 ) ) ;
#23298=ORIENTED_EDGE ( 'NONE', *, *, #38816, .T. ) ;
#23300=CARTESIAN_POINT ( 'NONE',  ( -57.58831721485822186, 1.394338577185886274, -1.315253866661476367 ) ) ;
#23308=AXIS2_PLACEMENT_3D ( 'NONE', #28263, #24635, #12076 ) ;
#23312=ORIENTED_EDGE ( 'NONE', *, *, #17586, .F. ) ;
#23317=CARTESIAN_POINT ( 'NONE',  ( -52.50198181065980663, 11.96455506022023307, -4.263607785004590589 ) ) ;
#23318=CARTESIAN_POINT ( 'NONE',  ( -30.50798996576767763, 65.61473877417354572, 1.523999999999992694 ) ) ;
#23320=LINE ( 'NONE', #781, #16104 ) ;
#23321=AXIS2_PLACEMENT_3D ( 'NONE', #26340, #32744, #3577 ) ;
#23323=CIRCLE ( 'NONE', #38313, 0.7620000000000000107 ) ;
#23334=CARTESIAN_POINT ( 'NONE',  ( -4.518622368304341386, 75.45558079800476037, 1.524000000000004462 ) ) ;
#23343=CARTESIAN_POINT ( 'NONE',  ( -23.91048590848665611, 81.84235438443283783, -1.270000000000006235 ) ) ;
#23345=EDGE_CURVE ( 'NONE', #31840, #38617, #20015, .T. ) ;
#23348=CARTESIAN_POINT ( 'NONE',  ( -57.20860189791900297, 2.757428422320434613, -2.041684569451241327 ) ) ;
#23355=ORIENTED_EDGE ( 'NONE', *, *, #356, .F. ) ;
#23356=VECTOR ( 'NONE', #37633, 1000.000000000000114 ) ;
#23359=CARTESIAN_POINT ( 'NONE',  ( -42.19606231239161787, 22.08888036620040296, 1.545000424059492339 ) ) ;
#23360=CIRCLE ( 'NONE', #20654, 0.6350000000000014522 ) ;
#23364=CARTESIAN_POINT ( 'NONE',  ( -17.14500000000466784, 71.11999999999886768, 1.269999999999998241 ) ) ;
#23371=CARTESIAN_POINT ( 'NONE',  ( -23.43300365160793319, 82.12916405548841681, 1.269999999999994023 ) ) ;
#23372=CARTESIAN_POINT ( 'NONE',  ( -48.76205491696826044, 18.14848438229189753, 5.115617678642917276 ) ) ;
#23373=CARTESIAN_POINT ( 'NONE',  ( -49.85168879002940656, 22.56840098298264152, 0.7122439767497134033 ) ) ;
#23375=CARTESIAN_POINT ( 'NONE',  ( -55.11216289415786207, 6.786895728730008237, 3.177266426849158609 ) ) ;
#23376=CARTESIAN_POINT ( 'NONE',  ( -58.24081614096904502, 0.5413803788780069404, 1.084122344208306332 ) ) ;
#23378=CARTESIAN_POINT ( 'NONE',  ( -17.14500000000466784, 71.11999999999886768, 1.269999999999998241 ) ) ;
#23379=ORIENTED_EDGE ( 'NONE', *, *, #37045, .T. ) ;
#23396=DIRECTION ( 'NONE',  ( -5.188838149069471174E-16, 1.699382548006136313E-16, 1.000000000000000000 ) ) ;
#23403=VERTEX_POINT ( 'NONE', #22041 ) ;
#23405=CARTESIAN_POINT ( 'NONE',  ( -41.93982928939168175, 22.21638423992008882, 1.241790202385180342 ) ) ;
#23410=AXIS2_PLACEMENT_3D ( 'NONE', #28537, #24915, #31515 ) ;
#23412=FACE_OUTER_BOUND ( 'NONE', #13463, .T. ) ;
#23416=ORIENTED_EDGE ( 'NONE', *, *, #27215, .T. ) ;
#23420=DIRECTION ( 'NONE',  ( 5.188838149069472160E-16, -1.699382548006136559E-16, -1.000000000000000000 ) ) ;
#23436=CARTESIAN_POINT ( 'NONE',  ( -28.69846420587789737, 77.20784726182124302, 1.269999999999991580 ) ) ;
#23437=DIRECTION ( 'NONE',  ( -0.3256999990547844170, -0.9454731675810337244, -8.328397965206681691E-18 ) ) ;
#23441=ADVANCED_FACE ( 'NONE', ( #5684 ), #5053, .F. ) ;
#23443=CARTESIAN_POINT ( 'NONE',  ( -13.79703500197643073, 79.79115557309579287, 1.523999999999998911 ) ) ;
#23450=ADVANCED_FACE ( 'NONE', ( #31213 ), #29711, .T. ) ;
#23451=CARTESIAN_POINT ( 'NONE',  ( -58.54066364324206972, -0.1080589709450771596, -0.6031363701337029148 ) ) ;
#23452=VERTEX_POINT ( 'NONE', #16071 ) ;
#23455=FILL_AREA_STYLE_COLOUR ( '', #21626 ) ;
#23460=CARTESIAN_POINT ( 'NONE',  ( -27.59695233663404679, 58.25262445104075226, -1.270000000000004015 ) ) ;
#23461=ORIENTED_EDGE ( 'NONE', *, *, #33952, .T. ) ;
#23463=ADVANCED_FACE ( 'NONE', ( #16284 ), #10113, .T. ) ;
#23468=CARTESIAN_POINT ( 'NONE',  ( -58.35999251409275246, -0.2710268728049192166, 0.1245515173811342219 ) ) ;
#23478=CARTESIAN_POINT ( 'NONE',  ( -52.67395729902614221, 10.59333423579336753, -2.513629069394799576 ) ) ;
#23481=DIRECTION ( 'NONE',  ( 0.9816537812491126225, 0.1906721105964872265, 8.537024980200846470E-16 ) ) ;
#23482=DIRECTION ( 'NONE',  ( -5.188838149069472160E-16, 1.699382548006136559E-16, 1.000000000000000000 ) ) ;
#23483=CARTESIAN_POINT ( 'NONE',  ( -29.42319995514127839, 68.34872547565998957, -1.524000000000006905 ) ) ;
#23486=CARTESIAN_POINT ( 'NONE',  ( -17.14500000000466784, 71.11999999999886768, -1.270000000000000684 ) ) ;
#23487=CARTESIAN_POINT ( 'NONE',  ( -57.84788464146735265, 2.520999533240836143, 0.7145982302433464550 ) ) ;
#23488=CARTESIAN_POINT ( 'NONE',  ( -58.60752282809816904, -0.1920500713008393978, 0.6598870774482750168 ) ) ;
#23490=ORIENTED_EDGE ( 'NONE', *, *, #28512, .F. ) ;
#23491=CARTESIAN_POINT ( 'NONE',  ( -55.74683331106318462, 9.129907917338066170, -0.4890489271862362708 ) ) ;
#23494=DIRECTION ( 'NONE',  ( -0.8745520943967999283, 0.4849315768086988609, -5.424246918827959078E-16 ) ) ;
#23504=DIRECTION ( 'NONE',  ( -0.8745520943968250194, 0.4849315768086532863, -5.361993529360574930E-16 ) ) ;
#23506=AXIS2_PLACEMENT_3D ( 'NONE', #31691, #31475, #37871 ) ;
#23509=CARTESIAN_POINT ( 'NONE',  ( -57.95255339509083825, 0.6073592009028576655, -0.9201367675222190678 ) ) ;
#23515=CARTESIAN_POINT ( 'NONE',  ( -47.00787117332040310, 24.49876931072293829, -2.333946431867834015 ) ) ;
#23519=ORIENTED_EDGE ( 'NONE', *, *, #11106, .F. ) ;
#23524=CARTESIAN_POINT ( 'NONE',  ( -53.83456308493991571, 9.379524109395250164, -3.755176697756441140 ) ) ;
#23525=ADVANCED_FACE ( 'NONE', ( #6097 ), #9286, .T. ) ;
#23527=B_SPLINE_SURFACE_WITH_KNOTS ( 'NONE', 3, 3, ( 
 ( #5771, #38136, #39983, #4829, #10774, #29375, #27386, #7807, #11190 ),
 ( #36987, #214, #3621, #33585, #19771, #9986, #23968, #30780, #14376 ),
 ( #40396, #32791, #16586, #13189, #1419, #6802, #1629, #22959, #16370 ),
 ( #20769, #1214, #4621, #33793, #29595, #20555, #27177, #26174, #14584 ),
 ( #39179, #3402, #17576, #30580, #24176, #37185, #40598, #4417, #8007 ),
 ( #10986, #17375, #23755, #35988, #36777, #20978, #8208, #7593, #33999 ),
 ( #1004, #17781, #27589, #30365, #14173, #40191, #13968, #11398, #24385 ),
 ( #26972, #37390, #32570, #11822, #2681, #37598, #41228, #31841, #27798 ),
 ( #15638, #5242, #24811, #34622, #38243, #28643, #17993, #2041, #12462 ),
 ( #41654, #28005, #35054, #41014, #30991, #15433, #38024, #41442, #22025 ),
 ( #1831, #34409, #21593, #8424, #40806, #12031, #18837, #2472, #25456 ),
 ( #11607, #5449, #18409, #5874, #21383, #34208, #37806, #38453, #8631 ),
 ( #31416, #2258, #15220, #34835, #28222, #31198, #24591, #25022, #21809 ),
 ( #8845, #14795, #21180, #5669, #5036, #18626, #18197, #15006, #9060 ),
 ( #31631, #28436, #12247, #25240, #19466, #330, #39291, #22434, #32903 ),
 ( #42079, #39082, #6081, #19673, #29697, #6287, #32474, #13082, #10097 ),
 ( #6704, #2886, #3304, #23070, #6918, #36103, #35464, #16269, #38868 ),
 ( #26074, #538, #13296, #118, #19887, #15849, #19044, #22228, #9884 ),
 ( #26283, #38663, #35257, #28855, #13512, #3734, #22856, #12872, #35894 ),
 ( #29059, #19258, #3522, #29489, #26501, #25861, #32688, #16483, #9680 ),
 ( #32266, #16692, #32049, #3096, #9271, #41868, #16057, #22646, #12667 ),
 ( #25656, #29271, #9471, #35680, #6489, #7965, #23491, #30116, #10725 ),
 ( #33956, #36316, #20295, #30738, #29907, #20932, #4152, #11148, #17115 ),
 ( #33748, #14127, #17531, #40353, #1163, #7135, #10520, #39933, #26714 ),
 ( #30318, #37143, #20724, #1586, #4573, #39722, #36518, #20092, #16905 ),
 ( #4787, #33536, #10311, #23923, #17737, #24134, #13720, #14544, #36725 ),
 ( #956, #33323, #39505, #745, #23280, #36939, #7337, #13925, #3945 ),
 ( #33116, #26918, #27128, #23705, #7547, #1372, #20508, #4368, #17328 ),
 ( #40142, #10934, #7760, #30532, #14329, #27341, #15172, #24981, #37980 ),
 ( #14961, #21763, #41398, #5408, #40971, #5201, #34165, #31159, #18580 ),
 ( #1998, #31588, #5831, #40764, #5623, #21979, #24766, #27963, #8588 ),
 ( #34368, #11775, #37553, #37764, #28178, #18156, #9015, #1791, #18364 ),
 ( #4991, #31370, #38198, #11562, #21552, #34581, #2426, #35012, #24343 ),
 ( #18786, #17949, #31799, #2214, #12203, #41183, #37348, #34789, #11986 ) ),
 .UNSPECIFIED., .F., .F., .F.,
 ( 4, 1, 1, 1, 1, 1, 1, 1, 1, 1, 1, 2, 1, 1, 1, 1, 1, 1, 1, 1, 1, 1, 1, 1, 1, 1, 1, 1, 1, 1, 4 ),
 ( 4, 1, 1, 1, 1, 1, 4 ),
 ( 0.000000000000000000, 0.01653533301974152714, 0.03307066603948305428, 0.04960599905922458142, 0.06614133207896610855, 0.09921199811844916283, 0.1322826641579322171, 0.1653533301974152714, 0.1984239962368983257, 0.2314946622763813799, 0.2500000000000000000, 0.2645653283158644342, 0.3105299952961229071, 0.3335123287862520325, 0.3564946622763812689, 0.4024593292566397418, 0.4943886632171566875, 0.5863179971776735222, 0.6666666666666666297, 0.6782473311381906900, 0.7701766650987074136, 0.8161413320789658865, 0.8850883325493537068, 0.8965794992944182695, 0.9080706660394826102, 0.9195618327845473949, 0.9310529995296121797, 0.9425441662746769644, 0.9540353330197415271, 0.9770176665098706525, 1.000000000000000000 ),
 ( 0.000000000000000000, 0.2500000000000000000, 0.4444444444444445308, 0.5000000000000000000, 0.7500000000000000000, 0.8333333333333333703, 1.000000000000000000 ),
 .UNSPECIFIED. ) ;
#23532=AXIS2_PLACEMENT_3D ( 'NONE', #11716, #24703, #20873 ) ;
#23535=CIRCLE ( 'NONE', #31707, 0.6350000000000014522 ) ;
#23537=AXIS2_PLACEMENT_3D ( 'NONE', #11084, #37908, #24071 ) ;
#23539=DIRECTION ( 'NONE',  ( -0.8745520943968241312, 0.4849315768086548406, -5.691349986800536046E-16 ) ) ;
#23541=ORIENTED_EDGE ( 'NONE', *, *, #16231, .F. ) ;
#23550=FACE_OUTER_BOUND ( 'NONE', #7207, .T. ) ;
#23554=DIRECTION ( 'NONE',  ( 0.1906721105964958585, -0.9816537812491110682, -9.356030339620071016E-15 ) ) ;
#23556=VERTEX_POINT ( 'NONE', #3317 ) ;
#23559=DIRECTION ( 'NONE',  ( -0.9336303900108928744, -0.3582377630123714241, 0.000000000000000000 ) ) ;
#23560=DIRECTION ( 'NONE',  ( 0.5149185422762211362, -0.8572391118119444542, 0.000000000000000000 ) ) ;
#23564=CARTESIAN_POINT ( 'NONE',  ( -58.82993853617958280, -0.2576789964487402607, -0.02280678271007593322 ) ) ;
#23565=DIRECTION ( 'NONE',  ( -0.8745520943968225769, 0.4849315768086578382, -5.691349986800571545E-16 ) ) ;
#23571=AXIS2_PLACEMENT_3D ( 'NONE', #22109, #17721, #27327 ) ;
#23574=DIRECTION ( 'NONE',  ( 0.8745520943968235761, -0.4849315768086558398, 0.000000000000000000 ) ) ;
#23579=CARTESIAN_POINT ( 'NONE',  ( -29.90236731146035609, 69.13284574330884880, -1.270000000000007123 ) ) ;
#23580=TOROIDAL_SURFACE ( 'NONE', #16098, 0.3810000000000002829, 0.2540000000000000036 ) ;
#23587=AXIS2_PLACEMENT_3D ( 'NONE', #24849, #1665, #40842 ) ;
#23588=CARTESIAN_POINT ( 'NONE',  ( -57.76462175338717486, 1.013803242785049630, 1.137036206963185414 ) ) ;
#23589=CARTESIAN_POINT ( 'NONE',  ( -48.57236063951932437, 24.64054515024589165, -8.874850105164511634E-15 ) ) ;
#23590=DIRECTION ( 'NONE',  ( 5.188838149069472160E-16, -1.699382548006136559E-16, -1.000000000000000000 ) ) ;
#23591=ADVANCED_FACE ( 'NONE', ( #9898 ), #7790, .T. ) ;
#23592=CARTESIAN_POINT ( 'NONE',  ( -52.30895062419047292, 13.66434875625866674, 4.401212925246481333 ) ) ;
#23593=CARTESIAN_POINT ( 'NONE',  ( -57.77616480963058621, 1.544201637102598168, 1.578764309266320831 ) ) ;
#23596=CIRCLE ( 'NONE', #12060, 0.7620000000000015650 ) ;
#23598=CARTESIAN_POINT ( 'NONE',  ( -43.82859865241511699, 24.63416949198730421, 1.523999999999993138 ) ) ;
#23608=DIRECTION ( 'NONE',  ( 0.9998501190848629872, 0.01731298258490734585, 8.537024980200777445E-16 ) ) ;
#23618=AXIS2_PLACEMENT_3D ( 'NONE', #25538, #25332, #25121 ) ;
#23621=CARTESIAN_POINT ( 'NONE',  ( -53.80167111242602118, 9.145755618221249605, 3.362987294923124537 ) ) ;
#23639=LINE ( 'NONE', #36662, #30191 ) ;
#23640=TOROIDAL_SURFACE ( 'NONE', #34560, 0.3810000000000002829, 0.2540000000000000036 ) ;
#23645=ORIENTED_EDGE ( 'NONE', *, *, #25006, .F. ) ;
#23650=LINE ( 'NONE', #480, #24979 ) ;
#23654=DIRECTION ( 'NONE',  ( -0.9454731675810359448, 0.3256999990547780333, -5.459396135145339171E-16 ) ) ;
#23661=LINE ( 'NONE', #27293, #526 ) ;
#23662=ORIENTED_EDGE ( 'NONE', *, *, #11563, .F. ) ;
#23663=FACE_OUTER_BOUND ( 'NONE', #27797, .T. ) ;
#23667=ORIENTED_EDGE ( 'NONE', *, *, #32062, .F. ) ;
#23668=DIRECTION ( 'NONE',  ( -5.188838149069472160E-16, 1.699382548006136559E-16, 1.000000000000000000 ) ) ;
#23675=CARTESIAN_POINT ( 'NONE',  ( -13.79703500197643073, 79.79115557309579287, 1.269999999999998685 ) ) ;
#23676=VERTEX_POINT ( 'NONE', #26297 ) ;
#23682=CARTESIAN_POINT ( 'NONE',  ( -48.97544177848091351, 17.83334834807254055, 5.075951225175634463 ) ) ;
#23686=AXIS2_PLACEMENT_3D ( 'NONE', #29000, #12813, #35404 ) ;
#23687=EDGE_CURVE ( 'NONE', #16908, #18068, #13220, .T. ) ;
#23692=CARTESIAN_POINT ( 'NONE',  ( -51.60883138897295908, 11.95321700621929040, -1.992363451474707947 ) ) ;
#23694=CARTESIAN_POINT ( 'NONE',  ( -11.73534362491071903, 82.73994711668952107, -1.524000000000000021 ) ) ;
#23695=CARTESIAN_POINT ( 'NONE',  ( -4.466782427718574588, 71.06098887363195615, 1.270000000000005791 ) ) ;
#23696=DIRECTION ( 'NONE',  ( -0.8745520943968241312, 0.4849315768086548406, -5.691349986800536046E-16 ) ) ;
#23697=CARTESIAN_POINT ( 'NONE',  ( -28.89366501045254765, 63.08038031660233003, -1.524000000000005128 ) ) ;
#23699=CARTESIAN_POINT ( 'NONE',  ( -46.43586784920008625, 25.95560800814362423, 1.524002373413926303 ) ) ;
#23701=CARTESIAN_POINT ( 'NONE',  ( -58.29256068059346063, 1.279866164410503604, 0.9167068831667634088 ) ) ;
#23704=ORIENTED_EDGE ( 'NONE', *, *, #29579, .F. ) ;
#23705=CARTESIAN_POINT ( 'NONE',  ( -58.00234944525002589, 2.059104932340308114, -0.8980956459801348046 ) ) ;
#23707=CIRCLE ( 'NONE', #29152, 0.6350000000000006750 ) ;
#23708=EDGE_LOOP ( 'NONE', ( #36727, #19350, #30240, #29303 ) ) ;
#23721=DIRECTION ( 'NONE',  ( -0.8745520943968240202, 0.4849315768086552292, -5.361993529360572958E-16 ) ) ;
#23722=ORIENTED_EDGE ( 'NONE', *, *, #36658, .F. ) ;
#23725=CARTESIAN_POINT ( 'NONE',  ( -58.24246139542360368, -0.02011471684311166505, -0.4719173402914386695 ) ) ;
#23730=CARTESIAN_POINT ( 'NONE',  ( -47.07934102874902749, 22.98505637820369429, -3.579966862081945145 ) ) ;
#23738=DIRECTION ( 'NONE',  ( 5.188838149069472160E-16, -1.699382548006136559E-16, -1.000000000000000000 ) ) ;
#23740=CARTESIAN_POINT ( 'NONE',  ( -55.11216289415786207, 6.786895728730008237, -3.177266426849177705 ) ) ;
#23744=AXIS2_PLACEMENT_3D ( 'NONE', #13670, #7289, #28857 ) ;
#23745=AXIS2_PLACEMENT_3D ( 'NONE', #1321, #33059, #40303 ) ;
#23754=ORIENTED_EDGE ( 'NONE', *, *, #41075, .F. ) ;
#23755=CARTESIAN_POINT ( 'NONE',  ( -47.17284909187768704, 24.49633334977720978, -1.858123130129392564 ) ) ;
#23757=CARTESIAN_POINT ( 'NONE',  ( -46.70722035912778125, 25.99002130463116700, -1.524000028481488522 ) ) ;
#23768=CIRCLE ( 'NONE', #16990, 0.7620000000000015650 ) ;
#23770=ORIENTED_EDGE ( 'NONE', *, *, #12017, .T. ) ;
#23773=CIRCLE ( 'NONE', #10158, 0.6349999999999998979 ) ;
#23776=CARTESIAN_POINT ( 'NONE',  ( -58.03077483564815964, 0.4858688437076191247, -1.087158688094550296 ) ) ;
#23777=DIRECTION ( 'NONE',  ( -0.7548010569845216011, -0.6559537821943317581, -2.801824109679580762E-16 ) ) ;
#23784=ADVANCED_FACE ( 'NONE', ( #16921 ), #7088, .T. ) ;
#23786=CARTESIAN_POINT ( 'NONE',  ( -26.51793118801306548, 72.98537704160715123, -1.524000000000006017 ) ) ;
#23787=EDGE_CURVE ( 'NONE', #27418, #33914, #17287, .T. ) ;
#23791=CARTESIAN_POINT ( 'NONE',  ( -26.37263903973852663, 72.23735686029533554, 1.523999999999993582 ) ) ;
#23792=CARTESIAN_POINT ( 'NONE',  ( -30.15519950990045572, 69.97033940222175374, -1.270000000000007123 ) ) ;
#23796=DIRECTION ( 'NONE',  ( 0.9336303900108815501, 0.3582377630124009560, 4.235673982319039874E-16 ) ) ;
#23798=ADVANCED_FACE ( 'NONE', ( #36333 ), #38403, .T. ) ;
#23800=DIRECTION ( 'NONE',  ( -0.8745520943968235761, 0.4849315768086558398, -4.268512490100410909E-16 ) ) ;
#23801=CARTESIAN_POINT ( 'NONE',  ( -56.94799265811163025, 2.765196624222747701, 1.846149193847710368 ) ) ;
#23802=CARTESIAN_POINT ( 'NONE',  ( -47.69778088985397346, 22.45332703829874887, 3.190613414150596405 ) ) ;
#23803=CARTESIAN_POINT ( 'NONE',  ( -50.15972161391664486, 17.13814111569220699, 4.955022299345067438 ) ) ;
#23804=CARTESIAN_POINT ( 'NONE',  ( -58.41428929413609694, 0.1660174354409331698, 0.8423104164767426516 ) ) ;
#23808=CARTESIAN_POINT ( 'NONE',  ( -45.68084146533627887, 21.25878370237693815, 4.188014402015102000 ) ) ;
#23817=ADVANCED_FACE ( 'NONE', ( #39737 ), #17938, .T. ) ;
#23820=CARTESIAN_POINT ( 'NONE',  ( -47.61073963479441318, 19.67761866749937028, 5.209507068477045699 ) ) ;
#23834=CARTESIAN_POINT ( 'NONE',  ( -47.89521659674720411, 15.90546175020217312, 0.7967971578063748339 ) ) ;
#23840=ORIENTED_EDGE ( 'NONE', *, *, #4860, .F. ) ;
#23849=ORIENTED_EDGE ( 'NONE', *, *, #34679, .F. ) ;
#23853=CIRCLE ( 'NONE', #5507, 0.5080000000000000071 ) ;
#23854=DIRECTION ( 'NONE',  ( 0.9816537812491075154, 0.1906721105965147323, 1.009874931538509940E-14 ) ) ;
#23856=FACE_OUTER_BOUND ( 'NONE', #14067, .T. ) ;
#23857=CIRCLE ( 'NONE', #4156, 0.7619999999999976792 ) ;
#23862=ORIENTED_EDGE ( 'NONE', *, *, #28742, .T. ) ;
#23868=DIRECTION ( 'NONE',  ( 5.188838149069472160E-16, -1.699382548006136559E-16, -1.000000000000000000 ) ) ;
#23870=DIRECTION ( 'NONE',  ( -0.4849315768086480682, -0.8745520943968280170, -1.030032898892941538E-16 ) ) ;
#23878=CARTESIAN_POINT ( 'NONE',  ( -36.98328822617348521, 27.82293856516310981, 1.269999999999995355 ) ) ;
#23881=CIRCLE ( 'NONE', #29328, 0.2540000000000012248 ) ;
#23884=VERTEX_POINT ( 'NONE', #35396 ) ;
#23889=CARTESIAN_POINT ( 'NONE',  ( -33.42971872652992005, 49.93539301574497102, 1.269999999999993578 ) ) ;
#23893=DIRECTION ( 'NONE',  ( 0.6850534820564753158, -0.7284927773988556510, -1.146843430008118057E-15 ) ) ;
#23898=AXIS2_PLACEMENT_3D ( 'NONE', #13457, #20246, #17683 ) ;
#23900=CARTESIAN_POINT ( 'NONE',  ( -58.34682947232719386, -0.2434262655763852479, 0.1887554165967793296 ) ) ;
#23910=CARTESIAN_POINT ( 'NONE',  ( -53.75865956017525349, 9.373754164828760338, -3.697140908559944261 ) ) ;
#23915=CARTESIAN_POINT ( 'NONE',  ( -29.14841176368481257, 63.09186355668505541, -1.270000000000006013 ) ) ;
#23917=DIRECTION ( 'NONE',  ( 5.188838149069472160E-16, -1.699382548006136559E-16, -1.000000000000000000 ) ) ;
#23919=CARTESIAN_POINT ( 'NONE',  ( -57.96050266256141725, 2.261623006455215634, 0.4698253072426024635 ) ) ;
#23920=CARTESIAN_POINT ( 'NONE',  ( -58.43690671596436914, -0.4125963578781866037, 0.2423173958219003998 ) ) ;
#23922=EDGE_LOOP ( 'NONE', ( #4636, #24518, #28179, #424 ) ) ;
#23923=CARTESIAN_POINT ( 'NONE',  ( -57.73934301000005576, 2.737667398473711433, -1.050169850737068478 ) ) ;
#23925=( BOUNDED_SURFACE ( )  B_SPLINE_SURFACE ( 3, 2, ( 
 ( #29252, #22628, #12233 ),
 ( #22420, #22837, #6474 ),
 ( #38850, #38440, #3287 ),
 ( #38229, #28840, #96 ),
 ( #2455, #6067, #28626 ),
 ( #9043, #13063, #29042 ) ),
 .UNSPECIFIED., .F., .F., .T. ) 
 B_SPLINE_SURFACE_WITH_KNOTS ( ( 4, 2, 4 ),
 ( 3, 3 ),
 ( 0.000000000000000000, 0.0007381999790946839474, 0.001476399958189367895 ),
 ( 0.000000000000000000, 1.000000000000000000 ),
 .UNSPECIFIED. ) 
 GEOMETRIC_REPRESENTATION_ITEM ( )  RATIONAL_B_SPLINE_SURFACE ( (
 ( 1.000000000000000000, 0.7071067811865388020, 1.000000000000000000),
 ( 1.000000000000000000, 0.7071031648627850164, 1.000000000000000000),
 ( 1.000000000000000000, 0.7049885726730517055, 1.000000000000000000),
 ( 1.000000000000000000, 0.6987948356720484755, 1.000000000000000000),
 ( 1.000000000000000000, 0.6949210395580179833, 1.000000000000000000),
 ( 1.000000000000000000, 0.6916534930270952231, 1.000000000000000000) ) ) 
 REPRESENTATION_ITEM ( '' )  SURFACE ( )  );
#23926=ORIENTED_EDGE ( 'NONE', *, *, #35977, .T. ) ;
#23935=CARTESIAN_POINT ( 'NONE',  ( -50.39203423948032423, 15.66273372407933273, -4.838163006325442161 ) ) ;
#23939=CARTESIAN_POINT ( 'NONE',  ( -58.22348609355718452, 0.02088251804533911363, -0.5098280860662359748 ) ) ;
#23943=CARTESIAN_POINT ( 'NONE',  ( -47.61549956331938205, 19.66157307908738261, -5.197827534590572895 ) ) ;
#23951=DIRECTION ( 'NONE',  ( 0.1906721105965043517, -0.9816537812491096249, 2.657572025465705161E-16 ) ) ;
#23953=CARTESIAN_POINT ( 'NONE',  ( -50.29507671575587580, 15.72791930032350827, -4.796563717952114558 ) ) ;
#23956=CARTESIAN_POINT ( 'NONE',  ( -36.43259636504752308, 28.15155085495446485, 1.269999999999994911 ) ) ;
#23964=AXIS2_PLACEMENT_3D ( 'NONE', #14177, #4625, #8011 ) ;
#23965=CARTESIAN_POINT ( 'NONE',  ( -57.35932467317038430, 1.578336987915054834, 0.2403330148843857983 ) ) ;
#23968=CARTESIAN_POINT ( 'NONE',  ( -46.71787546252079437, 26.08696747599453047, -0.2117558669993572784 ) ) ;
#23976=CARTESIAN_POINT ( 'NONE',  ( -41.09670346151854403, 23.04688172093031895, 1.270085369932502095 ) ) ;
#23978=CARTESIAN_POINT ( 'NONE',  ( -24.46582648842864316, 82.15028593570633575, 1.269999999999993356 ) ) ;
#23982=AXIS2_PLACEMENT_3D ( 'NONE', #32034, #25439, #25842 ) ;
#23983=CARTESIAN_POINT ( 'NONE',  ( -10.84307050033138431, 78.30450799593342026, -1.523999999999998911 ) ) ;
#23984=ORIENTED_EDGE ( 'NONE', *, *, #42044, .F. ) ;
#23988=CARTESIAN_POINT ( 'NONE',  ( -48.98643424070617414, 17.83616253325781642, -5.099923142903347362 ) ) ;
#23997=VECTOR ( 'NONE', #13204, 1000.000000000000000 ) ;
#24004=AXIS2_PLACEMENT_3D ( 'NONE', #27429, #14838, #21429 ) ;
#24011=DIRECTION ( 'NONE',  ( -0.8745520943968130290, 0.4849315768086749356, -6.829619984160618603E-16 ) ) ;
#24012=CARTESIAN_POINT ( 'NONE',  ( -57.51365629832210402, 1.555024991728927830, 1.385071661654051267 ) ) ;
#24014=CARTESIAN_POINT ( 'NONE',  ( -57.81953393267934160, 1.609514594907199392, 1.636666387507130782 ) ) ;
#24015=CARTESIAN_POINT ( 'NONE',  ( -58.52180102370724057, -0.06713305130389136954, 0.6434702267309780899 ) ) ;
#24018=DIRECTION ( 'NONE',  ( -0.8745520943968240202, 0.4849315768086553402, -6.829619984160650158E-16 ) ) ;
#24020=CARTESIAN_POINT ( 'NONE',  ( -42.09814309847200064, 23.46876350539121248, 1.523999999999994026 ) ) ;
#24024=VECTOR ( 'NONE', #10931, 1000.000000000000000 ) ;
#24034=AXIS2_PLACEMENT_3D ( 'NONE', #41047, #17815, #18227 ) ;
#24035=CARTESIAN_POINT ( 'NONE',  ( -45.60639265695088795, 20.98815520443602978, 4.238054969589494902 ) ) ;
#24036=CARTESIAN_POINT ( 'NONE',  ( -17.14500000000466784, 71.11999999999886768, 1.523999999999998689 ) ) ;
#24048=CARTESIAN_POINT ( 'NONE',  ( -49.81365592435692236, 14.60358288955459294, 2.185970286000758822 ) ) ;
#24053=ORIENTED_EDGE ( 'NONE', *, *, #8457, .F. ) ;
#24058=EDGE_LOOP ( 'NONE', ( #25243, #1663, #7886, #21716 ) ) ;
#24064=EDGE_CURVE ( 'NONE', #7720, #32811, #41107, .T. ) ;
#24065=AXIS2_PLACEMENT_3D ( 'NONE', #1361, #734, #1577 ) ;
#24067=EDGE_CURVE ( 'NONE', #1690, #4252, #988, .T. ) ;
#24068=CARTESIAN_POINT ( 'NONE',  ( -24.57769139521899149, 76.70147894597536720, -1.524000000000005572 ) ) ;
#24069=AXIS2_PLACEMENT_3D ( 'NONE', #24476, #37480, #4503 ) ;
#24071=DIRECTION ( 'NONE',  ( 6.829619984160660610E-15, 0.000000000000000000, 1.000000000000000000 ) ) ;
#24078=VECTOR ( 'NONE', #19537, 999.9999999999998863 ) ;
#24084=CARTESIAN_POINT ( 'NONE',  ( -28.36525985791271154, 77.02308833105713859, -1.524000000000007571 ) ) ;
#24089=DIRECTION ( 'NONE',  ( 0.6559537821943262070, -0.7548010569845264861, 8.537024980200723210E-16 ) ) ;
#24095=EDGE_CURVE ( 'NONE', #6738, #16059, #29546, .T. ) ;
#24097=VERTEX_POINT ( 'NONE', #31098 ) ;
#24098=ORIENTED_EDGE ( 'NONE', *, *, #35051, .T. ) ;
#24099=CARTESIAN_POINT ( 'NONE',  ( -6.559134203278485842, 78.24119908707510263, 1.524000000000002908 ) ) ;
#24105=DIRECTION ( 'NONE',  ( 0.1906721105965055174, -0.9816537812491091808, 0.000000000000000000 ) ) ;
#24106=ORIENTED_EDGE ( 'NONE', *, *, #2446, .T. ) ;
#24112=CARTESIAN_POINT ( 'NONE',  ( -55.76611385812141464, 5.250064693407802352, 2.603441191288020207 ) ) ;
#24120=CARTESIAN_POINT ( 'NONE',  ( -57.63883995378735392, 1.113466886629776997, -0.4249547484444705647 ) ) ;
#24123=DIRECTION ( 'NONE',  ( 5.188838149069472160E-16, -1.699382548006136559E-16, -1.000000000000000000 ) ) ;
#24124=DIRECTION ( 'NONE',  ( -0.9575201071113191853, 0.2883665106726643890, 1.122696976216276426E-15 ) ) ;
#24125=DIRECTION ( 'NONE',  ( -0.9816537812491089587, -0.1906721105965065444, -4.769617732184475162E-16 ) ) ;
#24130=CARTESIAN_POINT ( 'NONE',  ( -58.16194989728258946, 1.772972946764553193, -1.047404914941014506E-14 ) ) ;
#24134=CARTESIAN_POINT ( 'NONE',  ( -57.70501761738805158, 2.967533670478833763, -0.5494564739991270041 ) ) ;
#24135=EDGE_CURVE ( 'NONE', #4116, #34378, #24699, .T. ) ;
#24137=CARTESIAN_POINT ( 'NONE',  ( -45.09675090430819466, 21.02858785303356370, -3.680331723257411092 ) ) ;
#24142=CARTESIAN_POINT ( 'NONE',  ( -30.55012479247526613, 56.28806726182424569, 1.269999999999993801 ) ) ;
#24144=CARTESIAN_POINT ( 'NONE',  ( -49.49989884566186049, 17.08151615281530056, -5.027407696123642467 ) ) ;
#24145=ORIENTED_EDGE ( 'NONE', *, *, #16295, .T. ) ;
#24148=CARTESIAN_POINT ( 'NONE',  ( -58.28173089090353187, -0.1048243024652170952, -0.3852004869047068181 ) ) ;
#24152=CARTESIAN_POINT ( 'NONE',  ( -47.02779878473986486, 24.11651466984139702, -2.637840241488492943 ) ) ;
#24161=CARTESIAN_POINT ( 'NONE',  ( -54.32300027520380326, 9.724537220608771904, -3.743864951777645445 ) ) ;
#24168=CARTESIAN_POINT ( 'NONE',  ( -58.07447437077728125, 1.735896131820596766, -1.499107834811110429 ) ) ;
#24169=CARTESIAN_POINT ( 'NONE',  ( -45.61851195612273813, 20.88128798641513129, -4.109017096224391707 ) ) ;
#24171=CARTESIAN_POINT ( 'NONE',  ( -58.37241122568487128, -0.2962816677227753104, 0.2416009568453807155 ) ) ;
#24172=EDGE_CURVE ( 'NONE', #35654, #27477, #27694, .T. ) ;
#24176=CARTESIAN_POINT ( 'NONE',  ( -47.15184857521119710, 25.06101562935922900, -0.8929867115423409940 ) ) ;
#24187=ORIENTED_EDGE ( 'NONE', *, *, #32062, .T. ) ;
#24190=DIRECTION ( 'NONE',  ( 6.208586974181048556E-14, 1.531143599749384201E-13, -1.000000000000000000 ) ) ;
#24191=EDGE_LOOP ( 'NONE', ( #24725, #28846, #34017, #5624 ) ) ;
#24197=CARTESIAN_POINT ( 'NONE',  ( -54.56827866224300294, 7.775013980778200384, -3.396949012670559487 ) ) ;
#24208=ORIENTED_EDGE ( 'NONE', *, *, #33625, .F. ) ;
#24211=ADVANCED_FACE ( 'NONE', ( #41334 ), #1938, .F. ) ;
#24218=DIRECTION ( 'NONE',  ( 5.188838149069472160E-16, -1.699382548006136559E-16, -1.000000000000000000 ) ) ;
#24219=CARTESIAN_POINT ( 'NONE',  ( -57.90444776229139023, 0.7116094859540841311, 0.9800384988091017657 ) ) ;
#24220=CARTESIAN_POINT ( 'NONE',  ( -14.38915334913366806, 80.27078028363496287, -1.524000000000001132 ) ) ;
#24221=CARTESIAN_POINT ( 'NONE',  ( -58.24002838079472610, 0.001074765447070524793, 0.6562585879479657658 ) ) ;
#24222=CARTESIAN_POINT ( 'NONE',  ( -58.46457299168318400, 0.05672257835903128653, 0.7533826903934722763 ) ) ;
#24224=DIRECTION ( 'NONE',  ( 0.8745520943968472238, -0.4849315768086133738, -1.512686642312110832E-15 ) ) ;
#24228=CARTESIAN_POINT ( 'NONE',  ( -48.65005484009959957, 18.46594748123760965, 5.297328305960426142 ) ) ;
#24234=CIRCLE ( 'NONE', #29693, 0.2539999999999960067 ) ;
#24239=CARTESIAN_POINT ( 'NONE',  ( -8.816700480405424756, 73.94613776634058411, 1.524000000000002464 ) ) ;
#24240=CARTESIAN_POINT ( 'NONE',  ( -47.33874550351462318, 19.91900851599329414, 5.121984950673859061 ) ) ;
#24241=AXIS2_PLACEMENT_3D ( 'NONE', #4824, #16951, #37181 ) ;
#24242=CARTESIAN_POINT ( 'NONE',  ( -5.525052883313952279, 65.71034362490503611, -1.523999999999993804 ) ) ;
#24246=FACE_OUTER_BOUND ( 'NONE', #15944, .T. ) ;
#24254=CARTESIAN_POINT ( 'NONE',  ( -48.50421218116025557, 14.67712143704001626, -7.357606598588287537E-15 ) ) ;
#24262=CARTESIAN_POINT ( 'NONE',  ( -26.01970228765382132, 72.88622078690372064, -1.270000000000005791 ) ) ;
#24263=ADVANCED_FACE ( 'NONE', ( #40907 ), #5767, .T. ) ;
#24270=ADVANCED_FACE ( 'NONE', ( #21284 ), #34722, .T. ) ;
#24272=CIRCLE ( 'NONE', #16114, 0.2540000000000040559 ) ;
#24276=DIRECTION ( 'NONE',  ( -5.188838149069471174E-16, 1.699382548006136313E-16, 1.000000000000000000 ) ) ;
#24295=ORIENTED_EDGE ( 'NONE', *, *, #26687, .T. ) ;
#24296=DIRECTION ( 'NONE',  ( -0.6825627711659331132, -0.7308269722843310223, -2.299753143848214142E-16 ) ) ;
#24300=ORIENTED_EDGE ( 'NONE', *, *, #31808, .F. ) ;
#24302=DIRECTION ( 'NONE',  ( -0.01731298258488772612, 0.9998501190848633202, -1.788962107505314604E-16 ) ) ;
#24312=PLANE ( 'NONE',  #7283 ) ;
#24315=ORIENTED_EDGE ( 'NONE', *, *, #38480, .F. ) ;
#24319=VECTOR ( 'NONE', #1804, 1000.000000000000114 ) ;
#24320=EDGE_CURVE ( 'NONE', #13736, #35500, #36371, .T. ) ;
#24321=CARTESIAN_POINT ( 'NONE',  ( -57.02215525308559307, 2.672977372688998710, 2.026151568886835452 ) ) ;
#24329=CARTESIAN_POINT ( 'NONE',  ( -57.27679765945803325, 1.994406527888931135, -1.325560616021183025 ) ) ;
#24333=CARTESIAN_POINT ( 'NONE',  ( -8.313969523394650452, 67.96940778435646280, 1.270000000000003348 ) ) ;
#24342=ORIENTED_EDGE ( 'NONE', *, *, #30339, .F. ) ;
#24343=CARTESIAN_POINT ( 'NONE',  ( -58.73915225836901044, 0.1638436772961188170, -1.050014585470044348E-14 ) ) ;
#24344=VERTEX_POINT ( 'NONE', #22536 ) ;
#24353=ADVANCED_FACE ( 'NONE', ( #22741 ), #34329, .T. ) ;
#24354=CARTESIAN_POINT ( 'NONE',  ( -53.62081550738785296, 9.969973585557744045, -3.871466490782108139 ) ) ;
#24355=ORIENTED_EDGE ( 'NONE', *, *, #30339, .T. ) ;
#24358=CARTESIAN_POINT ( 'NONE',  ( -47.84356795211461844, 19.38525671449500010, -5.197506975155170572 ) ) ;
#24361=CARTESIAN_POINT ( 'NONE',  ( -47.87216941255763203, 19.82042534259524658, -5.426529464407940928 ) ) ;
#24368=CARTESIAN_POINT ( 'NONE',  ( -8.576171974424218192, 74.02775907367175989, 1.270000000000001350 ) ) ;
#24369=CARTESIAN_POINT ( 'NONE',  ( -14.38915334913366806, 80.27078028363496287, -1.524000000000001132 ) ) ;
#24371=DIRECTION ( 'NONE',  ( -0.8745520943968235761, 0.4849315768086558398, -5.691349986800547879E-16 ) ) ;
#24375=CARTESIAN_POINT ( 'NONE',  ( -30.19451713491628198, 70.61549828015994024, 1.269999999999991802 ) ) ;
#24376=AXIS2_PLACEMENT_3D ( 'NONE', #9307, #12704, #16091 ) ;
#24380=CARTESIAN_POINT ( 'NONE',  ( -25.70569512491730180, 74.05161654054386133, -1.524000000000005794 ) ) ;
#24381=CARTESIAN_POINT ( 'NONE',  ( -58.37241122568488549, -0.2962816677227891882, -1.041461608706327627E-14 ) ) ;
#24385=CARTESIAN_POINT ( 'NONE',  ( -48.57236063951932437, 24.64054515024589165, -1.011057066080545894E-14 ) ) ;
#24399=CARTESIAN_POINT ( 'NONE',  ( -17.65389921742010060, 84.42347906515803402, -1.524000000000003352 ) ) ;
#24400=LINE ( 'NONE', #30177, #21030 ) ;
#24405=CARTESIAN_POINT ( 'NONE',  ( -49.99157512322356922, 16.20856241626062655, -4.827055480674552257 ) ) ;
#24412=CIRCLE ( 'NONE', #42138, 8.794749999999996959 ) ;
#24414=CARTESIAN_POINT ( 'NONE',  ( -7.842268484490568348, 73.30875693322846587, -1.523999999999996247 ) ) ;
#24416=ORIENTED_EDGE ( 'NONE', *, *, #35498, .F. ) ;
#24423=CARTESIAN_POINT ( 'NONE',  ( -47.85244527695896011, 19.39403540832957518, 5.219971639306693056 ) ) ;
#24426=CARTESIAN_POINT ( 'NONE',  ( -57.91476036080663903, 0.6893188445402892439, 0.9676700770145346686 ) ) ;
#24428=CARTESIAN_POINT ( 'NONE',  ( -49.52983867584422484, 17.03535102234312859, 5.021609156700045595 ) ) ;
#24433=CARTESIAN_POINT ( 'NONE',  ( -47.87216941255763203, 19.82042534259524658, 5.426529464407925829 ) ) ;
#24437=FACE_OUTER_BOUND ( 'NONE', #36105, .T. ) ;
#24445=DIRECTION ( 'NONE',  ( -0.8745520943968235761, 0.4849315768086558398, -5.691349986800547879E-16 ) ) ;
#24446=CARTESIAN_POINT ( 'NONE',  ( -44.00561601145927426, 21.61144970255518771, 2.814601217462325167 ) ) ;
#24447=CARTESIAN_POINT ( 'NONE',  ( -28.60507221318229298, 76.72702915747851193, -1.524000000000007793 ) ) ;
#24459=CARTESIAN_POINT ( 'NONE',  ( -50.60903162571948855, 13.45680032611325849, 2.107060282091932191 ) ) ;
#24465=ORIENTED_EDGE ( 'NONE', *, *, #5652, .T. ) ;
#24468=EDGE_CURVE ( 'NONE', #35513, #1265, #21364, .T. ) ;
#24470=AXIS2_PLACEMENT_3D ( 'NONE', #18974, #40379, #15572 ) ;
#24476=CARTESIAN_POINT ( 'NONE',  ( -28.69846420587789737, 77.20784726182124302, -1.270000000000007567 ) ) ;
#24482=EDGE_LOOP ( 'NONE', ( #9942, #4646, #10874, #15399 ) ) ;
#24483=ORIENTED_EDGE ( 'NONE', *, *, #7382, .T. ) ;
#24499=EDGE_LOOP ( 'NONE', ( #13436, #24355, #8390, #10114, #36121, #32810 ) ) ;
#24506=DIRECTION ( 'NONE',  ( -5.188838149069471174E-16, 1.699382548006136313E-16, 1.000000000000000000 ) ) ;
#24518=ORIENTED_EDGE ( 'NONE', *, *, #22521, .T. ) ;
#24520=AXIS2_PLACEMENT_3D ( 'NONE', #28579, #15574, #2614 ) ;
#24522=CARTESIAN_POINT ( 'NONE',  ( -55.98935619762568194, 5.304184903327291423, 2.807757416346100765 ) ) ;
#24523=EDGE_CURVE ( 'NONE', #22644, #1116, #4670, .T. ) ;
#24531=CARTESIAN_POINT ( 'NONE',  ( -57.80191396384030611, 0.8575073823135492823, -0.7186190270693895155 ) ) ;
#24542=ADVANCED_FACE ( 'NONE', ( #30419 ), #28940, .F. ) ;
#24545=ORIENTED_EDGE ( 'NONE', *, *, #3533, .F. ) ;
#24546=DIRECTION ( 'NONE',  ( -0.8572391118119481179, -0.5149185422762151410, 0.000000000000000000 ) ) ;
#24548=ORIENTED_EDGE ( 'NONE', *, *, #26450, .F. ) ;
#24554=EDGE_CURVE ( 'NONE', #10652, #7108, #10722, .T. ) ;
#24558=CARTESIAN_POINT ( 'NONE',  ( -51.03298409374609435, 14.59756979370895991, -4.682653388026000840 ) ) ;
#24566=CARTESIAN_POINT ( 'NONE',  ( -53.83456308493991571, 9.379524109395250164, -3.755176697756441140 ) ) ;
#24573=CARTESIAN_POINT ( 'NONE',  ( -57.95878807693440393, 1.295030275130740094, -1.504629864475988787 ) ) ;
#24582=CARTESIAN_POINT ( 'NONE',  ( -42.98746435103614516, 21.25571956186866984, -0.9029888148949808402 ) ) ;
#24585=AXIS2_PLACEMENT_3D ( 'NONE', #35837, #6858, #9626 ) ;
#24587=CARTESIAN_POINT ( 'NONE',  ( -58.37241122568488549, -0.2962816677227891882, -1.042239624154175981E-14 ) ) ;
#24588=CARTESIAN_POINT ( 'NONE',  ( -50.10414895690885828, 20.83497401302349061, 1.621381026025490613 ) ) ;
#24591=CARTESIAN_POINT ( 'NONE',  ( -50.73416975447392474, 21.22185706673585059, -0.7846160747445178885 ) ) ;
#24600=DIRECTION ( 'NONE',  ( -5.188838149069471174E-16, 1.699382548006136313E-16, 1.000000000000000000 ) ) ;
#24601=AXIS2_PLACEMENT_3D ( 'NONE', #23065, #19882, #39500 ) ;
#24603=EDGE_CURVE ( 'NONE', #35748, #6398, #8380, .T. ) ;
#24605=FACE_OUTER_BOUND ( 'NONE', #41772, .T. ) ;
#24608=CARTESIAN_POINT ( 'NONE',  ( -47.36402078847329733, 19.94680556959678697, -5.177108626122005397 ) ) ;
#24612=CARTESIAN_POINT ( 'NONE',  ( -24.49496359545907609, 76.94162913054094588, -1.270000000000005569 ) ) ;
#24614=CARTESIAN_POINT ( 'NONE',  ( -58.45640570440971828, -0.4407481023139133147, -0.3169051027093325312 ) ) ;
#24623=AXIS2_PLACEMENT_3D ( 'NONE', #34572, #15377, #18146 ) ;
#24627=ORIENTED_EDGE ( 'NONE', *, *, #38665, .F. ) ;
#24629=CARTESIAN_POINT ( 'NONE',  ( -17.14500000000466784, 71.11999999999886768, 1.269999999999998241 ) ) ;
#24635=DIRECTION ( 'NONE',  ( 5.188838149069472160E-16, -1.699382548006136559E-16, -1.000000000000000000 ) ) ;
#24637=CARTESIAN_POINT ( 'NONE',  ( -23.34387769576312621, 77.71194901948682343, -1.524000000000005128 ) ) ;
#24638=CARTESIAN_POINT ( 'NONE',  ( -58.07466396318727675, 0.3426375511560262321, 0.7560645715230442931 ) ) ;
#24643=FACE_OUTER_BOUND ( 'NONE', #36074, .T. ) ;
#24645=CARTESIAN_POINT ( 'NONE',  ( -47.43570116002442205, 20.37060963802031566, 5.342502768866032703 ) ) ;
#24656=CARTESIAN_POINT ( 'NONE',  ( -29.36430674031901944, 68.35616281593667054, 1.523999999999992472 ) ) ;
#24657=DIRECTION ( 'NONE',  ( 5.188838149069472160E-16, -1.699382548006136559E-16, -1.000000000000000000 ) ) ;
#24658=CARTESIAN_POINT ( 'NONE',  ( -42.47169588413780161, 21.98427696618763960, 1.915014136675358580 ) ) ;
#24659=DIRECTION ( 'NONE',  ( 0.6559537821943239866, -0.7548010569845283735, 4.686333752532408853E-16 ) ) ;
#24671=ORIENTED_EDGE ( 'NONE', *, *, #41569, .F. ) ;
#24672=CARTESIAN_POINT ( 'NONE',  ( -57.27679765945803325, 1.994406527888931135, 1.325560616021162597 ) ) ;
#24678=CIRCLE ( 'NONE', #6331, 3.111499999999999932 ) ;
#24679=EDGE_LOOP ( 'NONE', ( #14184, #20361, #6778, #25520 ) ) ;
#24683=AXIS2_PLACEMENT_3D ( 'NONE', #13804, #6634, #36817 ) ;
#24684=VERTEX_POINT ( 'NONE', #1944 ) ;
#24687=CARTESIAN_POINT ( 'NONE',  ( -9.909999474182706436, 76.95545850745379823, 1.524000000000001576 ) ) ;
#24690=CARTESIAN_POINT ( 'NONE',  ( -23.43300365160792964, 82.12916405548841681, -1.270000000000006013 ) ) ;
#24695=CARTESIAN_POINT ( 'NONE',  ( -7.921807157844599878, 72.80702234259206307, -1.269999999999996021 ) ) ;
#24697=VERTEX_POINT ( 'NONE', #21920 ) ;
#24699=LINE ( 'NONE', #8528, #13884 ) ;
#24703=DIRECTION ( 'NONE',  ( -5.188838149069472160E-16, 1.699382548006136559E-16, 1.000000000000000000 ) ) ;
#24711=ADVANCED_FACE ( 'NONE', ( #14903 ), #18306, .T. ) ;
#24713=CARTESIAN_POINT ( 'NONE',  ( -38.65395868481546415, 29.38327706004843876, -1.270000000000004903 ) ) ;
#24723=ORIENTED_EDGE ( 'NONE', *, *, #38040, .T. ) ;
#24725=ORIENTED_EDGE ( 'NONE', *, *, #24776, .T. ) ;
#24730=CARTESIAN_POINT ( 'NONE',  ( -41.28107547821694112, 23.22158991241130011, 1.523999999999988475 ) ) ;
#24733=VECTOR ( 'NONE', #3310, 1000.000000000000114 ) ;
#24741=AXIS2_PLACEMENT_3D ( 'NONE', #34096, #36876, #30253 ) ;
#24742=CARTESIAN_POINT ( 'NONE',  ( -58.45128286774038884, -0.4309378487369980304, 0.3205346425638702090 ) ) ;
#24747=AXIS2_PLACEMENT_3D ( 'NONE', #1782, #4982, #27332 ) ;
#24748=AXIS2_PLACEMENT_3D ( 'NONE', #6567, #25524, #38524 ) ;
#24753=CARTESIAN_POINT ( 'NONE',  ( -57.65203525413342334, 1.118929822212927361, -0.5921937322712454987 ) ) ;
#24756=AXIS2_PLACEMENT_3D ( 'NONE', #34943, #25129, #30890 ) ;
#24760=CARTESIAN_POINT ( 'NONE',  ( -29.91139568370675761, 83.95719535527389610, 1.523999999999989807 ) ) ;
#24761=CARTESIAN_POINT ( 'NONE',  ( -58.83227707057486811, -0.08366279997995551554, -1.533110566128066119E-14 ) ) ;
#24765=ORIENTED_EDGE ( 'NONE', *, *, #10530, .F. ) ;
#24766=CARTESIAN_POINT ( 'NONE',  ( -58.35673254475433680, 1.205555466438051893, -0.1480423017862652624 ) ) ;
#24767=VERTEX_POINT ( 'NONE', #3838 ) ;
#24768=CARTESIAN_POINT ( 'NONE',  ( -47.84356795211438396, 19.38525671449516352, -5.197506975155015141 ) ) ;
#24775=CARTESIAN_POINT ( 'NONE',  ( -48.65109498377578490, 18.34191667582345175, -5.169736723450931493 ) ) ;
#24776=EDGE_CURVE ( 'NONE', #40395, #25154, #29476, .T. ) ;
#24781=CARTESIAN_POINT ( 'NONE',  ( -56.28088753042789705, 4.173514606889340506, -2.292216047950881297 ) ) ;
#24784=CARTESIAN_POINT ( 'NONE',  ( -51.73272837791831336, 13.19950324185369794, -4.393710239503588078 ) ) ;
#24792=CARTESIAN_POINT ( 'NONE',  ( -57.92346726745822849, 0.7446056814934959300, -1.206286704679871535 ) ) ;
#24793=MANIFOLD_SOLID_BREP ( 'Stock-MAS-162-1', #38728 ) ;
#24794=CARTESIAN_POINT ( 'NONE',  ( -29.81357423954495189, 70.62209452652477637, 1.523999999999992250 ) ) ;
#24796=DIRECTION ( 'NONE',  ( -0.8745520943968249084, 0.4849315768086536194, -5.575199987069925217E-16 ) ) ;
#24803=CARTESIAN_POINT ( 'NONE',  ( -43.08902205111511563, 20.96483665317663991, -0.2987222196696421861 ) ) ;
#24804=ORIENTED_EDGE ( 'NONE', *, *, #6574, .T. ) ;
#24807=DIRECTION ( 'NONE',  ( -0.8745520943968246863, 0.4849315768086537859, -5.361993529360573944E-16 ) ) ;
#24808=CARTESIAN_POINT ( 'NONE',  ( -51.58376292578905975, 16.21309621351152330, 3.606096628736468634 ) ) ;
#24810=ORIENTED_EDGE ( 'NONE', *, *, #39334, .T. ) ;
#24811=CARTESIAN_POINT ( 'NONE',  ( -47.69778088985397346, 22.45332703829874887, -3.190613414150612837 ) ) ;
#24822=CARTESIAN_POINT ( 'NONE',  ( -17.64290547347870941, 83.78857423953914463, -1.270000000000003126 ) ) ;
#24828=AXIS2_PLACEMENT_3D ( 'NONE', #35995, #9993, #22336 ) ;
#24832=CARTESIAN_POINT ( 'NONE',  ( -48.43799250123969102, 18.62746361536592943, -5.176101822179832723 ) ) ;
#24838=ORIENTED_EDGE ( 'NONE', *, *, #26384, .T. ) ;
#24844=B_SPLINE_CURVE_WITH_KNOTS ( 'NONE', 3,
 ( #34951, #21495, #15326, #25136, #37712, #11505, #2368, #18518, #8535, #37496, #31108, #14904, #15543, #38140, #5354, #18307, #27907, #8954, #12361, #21085, #8321, #30898 ),
 .UNSPECIFIED., .F., .F.,
 ( 4, 1, 1, 1, 1, 1, 1, 1, 1, 1, 1, 1, 1, 1, 1, 1, 1, 1, 1, 4 ),
 ( 0.000000000000000000, 0.02298233349012935092, 0.04596466698025848674, 0.05745583372532304250, 0.06894700047038783419, 0.08043816721545261894, 0.09192933396051740369, 0.1034205007055817443, 0.1149116674506463071, 0.1838586679210341135, 0.2298233349012926141, 0.3217526688618093655, 0.3333333333333334259, 0.4136820028223265333, 0.5056113367828434235, 0.5975406707433602582, 0.6435053377236188421, 0.6664876712137480785, 0.6894700047038772039, 0.7354344192538687652 ),
 .UNSPECIFIED. ) ;
#24849=CARTESIAN_POINT ( 'NONE',  ( -30.15642192025596202, 71.36377005712995469, -1.270000000000007345 ) ) ;
#24856=CARTESIAN_POINT ( 'NONE',  ( -46.68395179480138779, 26.03198510454123848, -1.524000000000008459 ) ) ;
#24857=AXIS2_PLACEMENT_3D ( 'NONE', #31262, #34683, #15280 ) ;
#24860=CARTESIAN_POINT ( 'NONE',  ( -58.09361251268546766, 0.3016395514430970093, 0.7289802440182748811 ) ) ;
#24861=CARTESIAN_POINT ( 'NONE',  ( -29.18709815850009903, 67.04824513552235032, -1.524000000000005794 ) ) ;
#24862=DIRECTION ( 'NONE',  ( 0.7770581983690837413, -0.6294287539884032556, 5.101669463485834765E-16 ) ) ;
#24865=ORIENTED_EDGE ( 'NONE', *, *, #39968, .T. ) ;
#24866=CARTESIAN_POINT ( 'NONE',  ( -50.15972161391664486, 17.13814111569220699, 4.955022299345067438 ) ) ;
#24871=DIRECTION ( 'NONE',  ( -0.8745520943968235761, 0.4849315768086558398, -5.691349986800547879E-16 ) ) ;
#24873=ORIENTED_EDGE ( 'NONE', *, *, #6991, .T. ) ;
#24875=CARTESIAN_POINT ( 'NONE',  ( -31.80708539065861373, 53.04900798524919736, 1.269999999999994467 ) ) ;
#24876=CYLINDRICAL_SURFACE ( 'NONE', #36456, 0.6350000000000006750 ) ;
#24877=CARTESIAN_POINT ( 'NONE',  ( -7.772068811996249771, 69.25462295839062676, 1.270000000000003570 ) ) ;
#24878=CARTESIAN_POINT ( 'NONE',  ( -47.87705743256026381, 19.40768263586563691, 5.264533221178260725 ) ) ;
#24889=ORIENTED_EDGE ( 'NONE', *, *, #2710, .T. ) ;
#24890=CARTESIAN_POINT ( 'NONE',  ( -56.90438685736649660, 2.765855619508456265, 1.561774844827657605 ) ) ;
#24894=VERTEX_POINT ( 'NONE', #41073 ) ;
#24899=EDGE_LOOP ( 'NONE', ( #15594, #32674, #14197, #8124 ) ) ;
#24901=DIRECTION ( 'NONE',  ( -0.4849315768086425726, -0.8745520943968309036, -1.030032898892908012E-16 ) ) ;
#24903=EDGE_CURVE ( 'NONE', #29093, #9109, #38333, .T. ) ;
#24914=ORIENTED_EDGE ( 'NONE', *, *, #26749, .F. ) ;
#24915=DIRECTION ( 'NONE',  ( 0.6559537821943240976, -0.7548010569845284845, 4.686333752532409839E-16 ) ) ;
#24916=AXIS2_PLACEMENT_3D ( 'NONE', #4719, #34718, #31509 ) ;
#24929=DIRECTION ( 'NONE',  ( -5.188838149069472160E-16, 1.699382548006136559E-16, 1.000000000000000000 ) ) ;
#24933=ORIENTED_EDGE ( 'NONE', *, *, #13629, .F. ) ;
#24941=DIRECTION ( 'NONE',  ( -5.188838149069471174E-16, 1.699382548006136313E-16, 1.000000000000000000 ) ) ;
#24947=AXIS2_PLACEMENT_3D ( 'NONE', #23364, #36398, #20174 ) ;
#24954=ORIENTED_EDGE ( 'NONE', *, *, #7451, .F. ) ;
#24958=CARTESIAN_POINT ( 'NONE',  ( -58.21232023750257412, 0.08677210334570391315, 0.8315773506257112535 ) ) ;
#24963=CIRCLE ( 'NONE', #23618, 0.2539999999999981162 ) ;
#24967=CARTESIAN_POINT ( 'NONE',  ( -57.29531047346088712, 2.067549486662559222, -1.749273462387502809 ) ) ;
#24975=DIRECTION ( 'NONE',  ( 5.188838149069472160E-16, -1.699382548006136559E-16, -1.000000000000000000 ) ) ;
#24979=VECTOR ( 'NONE', #7281, 1000.000000000000000 ) ;
#24981=CARTESIAN_POINT ( 'NONE',  ( -58.03428750496623678, 2.144022121626051991, -0.09394692876221440170 ) ) ;
#24982=ORIENTED_EDGE ( 'NONE', *, *, #31794, .F. ) ;
#24983=CARTESIAN_POINT ( 'NONE',  ( -42.22422426686775765, 22.06987237837593696, -1.558155077124144583 ) ) ;
#24990=CARTESIAN_POINT ( 'NONE',  ( -58.43714447420092739, 0.1158066806379677849, -0.8009346905749505918 ) ) ;
#24991=EDGE_LOOP ( 'NONE', ( #41884, #17546, #12377, #36434 ) ) ;
#24993=LINE ( 'NONE', #15188, #40675 ) ;
#24995=CARTESIAN_POINT ( 'NONE',  ( -53.68617469749651860, 9.442005736215490330, -3.589663193476668290 ) ) ;
#24998=CARTESIAN_POINT ( 'NONE',  ( -49.56090548067184898, 17.87959676410238430, -5.165259844110624776 ) ) ;
#24999=AXIS2_PLACEMENT_3D ( 'NONE', #2439, #25423, #5214 ) ;
#25001=ORIENTED_EDGE ( 'NONE', *, *, #23149, .T. ) ;
#25006=EDGE_CURVE ( 'NONE', #11474, #1265, #11778, .T. ) ;
#25007=CARTESIAN_POINT ( 'NONE',  ( -58.87911280034276018, -0.2081424763510641984, -0.2451831517279998984 ) ) ;
#25010=FACE_OUTER_BOUND ( 'NONE', #38638, .T. ) ;
#25014=CARTESIAN_POINT ( 'NONE',  ( -42.80040666669066241, 21.79149265709745009, -2.067570201390457552 ) ) ;
#25017=DIRECTION ( 'NONE',  ( -5.188838149069471174E-16, 1.699382548006136313E-16, 1.000000000000000000 ) ) ;
#25019=CARTESIAN_POINT ( 'NONE',  ( -50.45326722236683281, 19.63324548489221044, 2.269669894115894593 ) ) ;
#25022=CARTESIAN_POINT ( 'NONE',  ( -51.10637696787394191, 21.44594517334857287, -0.3731469903906515784 ) ) ;
#25035=EDGE_CURVE ( 'NONE', #40156, #4929, #19927, .T. ) ;
#25037=CARTESIAN_POINT ( 'NONE',  ( -41.05189575270520663, 23.09451173561983239, -1.523999999999987365 ) ) ;
#25038=DIRECTION ( 'NONE',  ( 5.188838149069472160E-16, -1.699382548006136559E-16, -1.000000000000000000 ) ) ;
#25039=VERTEX_POINT ( 'NONE', #5303 ) ;
#25066=DIRECTION ( 'NONE',  ( -0.8745520943968310146, 0.4849315768086426837, -5.361993529360588735E-16 ) ) ;
#25067=CIRCLE ( 'NONE', #23686, 0.7620000000000000107 ) ;
#25068=CARTESIAN_POINT ( 'NONE',  ( -58.05759491991644694, 0.3796087429759146814, 0.7800566416505788636 ) ) ;
#25070=CARTESIAN_POINT ( 'NONE',  ( -18.83202234259777086, 80.34319284215894186, -1.270000000000002904 ) ) ;
#25071=DIRECTION ( 'NONE',  ( -0.8745520943968243532, 0.4849315768086547296, -5.361993529360573944E-16 ) ) ;
#25074=CARTESIAN_POINT ( 'NONE',  ( -52.76912830878634253, 12.08540908813377612, 4.334427935445234858 ) ) ;
#25079=CARTESIAN_POINT ( 'NONE',  ( -37.66124916107632714, 74.02712188174415076, -1.270000000000011786 ) ) ;
#25080=EDGE_LOOP ( 'NONE', ( #9344, #16215, #2522, #9337, #23030, #36986 ) ) ;
#25082=CARTESIAN_POINT ( 'NONE',  ( -33.42971872652992005, 49.93539301574497102, 1.269999999999994023 ) ) ;
#25087=EDGE_CURVE ( 'NONE', #22433, #3009, #28784, .T. ) ;
#25095=CIRCLE ( 'NONE', #16912, 0.2539999999999992819 ) ;
#25098=EDGE_CURVE ( 'NONE', #28177, #1859, #2288, .T. ) ;
#25101=CARTESIAN_POINT ( 'NONE',  ( -57.22211421646275653, 1.778355698664441098, -1.009576694067165286E-14 ) ) ;
#25105=ORIENTED_EDGE ( 'NONE', *, *, #26636, .F. ) ;
#25107=VERTEX_POINT ( 'NONE', #5506 ) ;
#25111=EDGE_LOOP ( 'NONE', ( #11690, #30990, #3303 ) ) ;
#25113=DIRECTION ( 'NONE',  ( -0.8745520943968269068, 0.4849315768086501222, -8.537024980200721238E-16 ) ) ;
#25119=DIRECTION ( 'NONE',  ( -0.01731298258488772612, 0.9998501190848634312, -1.788962107505314851E-16 ) ) ;
#25120=CARTESIAN_POINT ( 'NONE',  ( -46.95274714683655759, 25.03842815569886326, 1.954508796226629208 ) ) ;
#25121=DIRECTION ( 'NONE',  ( 0.9469626219732555361, 0.3213437296502561491, 8.537024980200885913E-16 ) ) ;
#25123=CARTESIAN_POINT ( 'NONE',  ( -47.16890147375937659, 22.20336809214646578, 4.187060126831876339 ) ) ;
#25124=CARTESIAN_POINT ( 'NONE',  ( -24.10666987309389597, 82.16896248603319464, -1.524000000000006239 ) ) ;
#25126=EDGE_CURVE ( 'NONE', #13983, #29032, #30901, .T. ) ;
#25129=DIRECTION ( 'NONE',  ( -5.188838149069472160E-16, 1.699382548006136559E-16, 1.000000000000000000 ) ) ;
#25133=FACE_OUTER_BOUND ( 'NONE', #17690, .T. ) ;
#25136=CARTESIAN_POINT ( 'NONE',  ( -58.50860430493788300, 0.7049166599848583070, 0.9756837515128382599 ) ) ;
#25152=ADVANCED_FACE ( 'NONE', ( #6543 ), #3144, .F. ) ;
#25154=VERTEX_POINT ( 'NONE', #42129 ) ;
#25157=CARTESIAN_POINT ( 'NONE',  ( -41.05189575270519242, 23.09451173561982174, 0.2116666666666617014 ) ) ;
#25165=APPLICATION_CONTEXT ( 'automotive_design' ) ;
#25175=CARTESIAN_POINT ( 'NONE',  ( -58.44960050528106876, -0.4277149010491103076, 0.3217025345704653261 ) ) ;
#25187=DIRECTION ( 'NONE',  ( -0.8745520943968240202, 0.4849315768086551737, -5.361993529360572958E-16 ) ) ;
#25196=CARTESIAN_POINT ( 'NONE',  ( -8.438477507926631205, 69.62414081991882142, 1.270000000000003126 ) ) ;
#25200=AXIS2_PLACEMENT_3D ( 'NONE', #15074, #23131, #35319 ) ;
#25204=CARTESIAN_POINT ( 'NONE',  ( -57.59359650234090822, 1.936081701823850088, -1.738013837494228220 ) ) ;
#25209=CARTESIAN_POINT ( 'NONE',  ( -51.06239344698444427, 14.35285235637163659, -4.522483476426243598 ) ) ;
#25211=AXIS2_PLACEMENT_3D ( 'NONE', #14059, #1304, #885 ) ;
#25214=CARTESIAN_POINT ( 'NONE',  ( -56.71132732703541990, 3.319205314284062958, -2.191228219141365230 ) ) ;
#25220=CARTESIAN_POINT ( 'NONE',  ( -57.78858274104275949, 1.044662872677112997, -1.355440516197766732 ) ) ;
#25223=CARTESIAN_POINT ( 'NONE',  ( -5.525052883313952279, 65.71034362490503611, -1.269999999999993801 ) ) ;
#25227=LINE ( 'NONE', #13498, #16087 ) ;
#25228=CARTESIAN_POINT ( 'NONE',  ( -41.90039389258884484, 22.27519970079744382, -1.481527307957015926 ) ) ;
#25229=ORIENTED_EDGE ( 'NONE', *, *, #32944, .F. ) ;
#25230=DIRECTION ( 'NONE',  ( 5.188838149069472160E-16, -1.699382548006136559E-16, -1.000000000000000000 ) ) ;
#25231=CIRCLE ( 'NONE', #30671, 0.2540000000000052771 ) ;
#25232=CARTESIAN_POINT ( 'NONE',  ( -57.95878807693440393, 1.295030275130740094, 1.504629864475967915 ) ) ;
#25233=CARTESIAN_POINT ( 'NONE',  ( -56.50625740582004397, 4.231662007982201601, 2.501568669484166563 ) ) ;
#25236=CARTESIAN_POINT ( 'NONE',  ( -49.25189787529244967, 18.82624764011888630, 4.709232814563275582 ) ) ;
#25240=CARTESIAN_POINT ( 'NONE',  ( -50.06058399760020450, 19.37794936593257589, -3.106418048087412842 ) ) ;
#25243=ORIENTED_EDGE ( 'NONE', *, *, #36259, .T. ) ;
#25248=DIRECTION ( 'NONE',  ( -0.7770581983690896255, 0.6294287539883960392, 1.268759650262045389E-15 ) ) ;
#25253=DIRECTION ( 'NONE',  ( -0.8745520943968247973, 0.4849315768086537304, -5.361993529360573944E-16 ) ) ;
#25263=CIRCLE ( 'NONE', #6899, 0.2540000000000000591 ) ;
#25271=ORIENTED_EDGE ( 'NONE', *, *, #17876, .T. ) ;
#25281=CARTESIAN_POINT ( 'NONE',  ( -58.34772544449950971, -0.2453081154814788778, 0.1850187449336859469 ) ) ;
#25287=ORIENTED_EDGE ( 'NONE', *, *, #34464, .T. ) ;
#25291=CARTESIAN_POINT ( 'NONE',  ( -28.94717034978515713, 63.96727089252595988, 1.523999999999992916 ) ) ;
#25296=CARTESIAN_POINT ( 'NONE',  ( -29.24370919332844210, 62.65993627038479019, 1.523999999999994470 ) ) ;
#25298=CARTESIAN_POINT ( 'NONE',  ( -41.34781391884743584, 22.78346824045823737, 1.529410470707965208 ) ) ;
#25310=VERTEX_POINT ( 'NONE', #35307 ) ;
#25312=CARTESIAN_POINT ( 'NONE',  ( -54.22787649382025421, 6.886497292746610377, -9.139123573059997208E-15 ) ) ;
#25320=ORIENTED_EDGE ( 'NONE', *, *, #36240, .T. ) ;
#25325=ADVANCED_FACE ( 'NONE', ( #22490 ), #41720, .T. ) ;
#25331=CARTESIAN_POINT ( 'NONE',  ( -46.87366875892457330, 25.48678770706554175, 1.642247700512937669 ) ) ;
#25332=DIRECTION ( 'NONE',  ( -0.3213437296502708040, 0.9469626219732506511, -9.578090222180217247E-17 ) ) ;
#25333=EDGE_CURVE ( 'NONE', #41136, #19839, #31898, .T. ) ;
#25335=CARTESIAN_POINT ( 'NONE',  ( -46.82679756180435504, 21.08486709759267086, 4.907624977305271585 ) ) ;
#25340=DIRECTION ( 'NONE',  ( -5.188838149069472160E-16, 1.699382548006136559E-16, 1.000000000000000000 ) ) ;
#25346=AXIS2_PLACEMENT_3D ( 'NONE', #19891, #22860, #23494 ) ;
#25348=DIRECTION ( 'NONE',  ( -5.188838149069471174E-16, 1.699382548006136313E-16, 1.000000000000000000 ) ) ;
#25362=TOROIDAL_SURFACE ( 'NONE', #39661, 0.3809999999999999498, 0.2540000000000000036 ) ;
#25376=DIRECTION ( 'NONE',  ( -0.2290273297124504059, 0.9734199927291325993, 0.000000000000000000 ) ) ;
#25378=EDGE_CURVE ( 'NONE', #29332, #32282, #14533, .T. ) ;
#25381=CARTESIAN_POINT ( 'NONE',  ( -25.80936006922821591, 73.72935646344811289, -1.270000000000005791 ) ) ;
#25385=AXIS2_PLACEMENT_3D ( 'NONE', #21093, #27087, #14086 ) ;
#25391=ADVANCED_FACE ( 'NONE', ( #38503 ), #33521, .T. ) ;
#25403=CARTESIAN_POINT ( 'NONE',  ( -30.20416046766210272, 71.17241488000101413, -1.270000000000007345 ) ) ;
#25411=DIRECTION ( 'NONE',  ( -0.9816537812491089587, -0.1906721105965065444, -4.769617732184475162E-16 ) ) ;
#25412=VERTEX_POINT ( 'NONE', #30171 ) ;
#25413=DIRECTION ( 'NONE',  ( -0.8745520943968243532, 0.4849315768086547296, -6.829619984160642269E-16 ) ) ;
#25419=CARTESIAN_POINT ( 'NONE',  ( -58.40556995236380544, 0.1837532267470638192, -0.8520485832066984067 ) ) ;
#25423=DIRECTION ( 'NONE',  ( 5.188838149069472160E-16, -1.699382548006136559E-16, -1.000000000000000000 ) ) ;
#25425=DIRECTION ( 'NONE',  ( -0.8745520943968225769, 0.4849315768086578382, -5.691349986800571545E-16 ) ) ;
#25428=CARTESIAN_POINT ( 'NONE',  ( -50.29507671575587580, 15.72791930032350827, -4.796563717952114558 ) ) ;
#25429=CIRCLE ( 'NONE', #16561, 0.2540000000000000036 ) ;
#25431=ORIENTED_EDGE ( 'NONE', *, *, #31589, .T. ) ;
#25434=CIRCLE ( 'NONE', #35657, 0.7620000000000030083 ) ;
#25436=CARTESIAN_POINT ( 'NONE',  ( -5.861642722916909243, 64.54502714855203749, 1.524000000000005572 ) ) ;
#25439=DIRECTION ( 'NONE',  ( -5.188838149069471174E-16, 1.699382548006136313E-16, 1.000000000000000000 ) ) ;
#25446=CARTESIAN_POINT ( 'NONE',  ( -47.44699234454015624, 15.94620872345377904, -0.4021177788561511313 ) ) ;
#25448=CARTESIAN_POINT ( 'NONE',  ( -57.66338803320029882, 2.692357263605615891, 1.869785753600835987 ) ) ;
#25449=CARTESIAN_POINT ( 'NONE',  ( -53.62923018145963283, 9.955465683803918608, 3.869326235999875241 ) ) ;
#25450=CARTESIAN_POINT ( 'NONE',  ( -29.63955751525485383, 69.20430988267358430, -1.524000000000006905 ) ) ;
#25451=AXIS2_PLACEMENT_3D ( 'NONE', #27066, #17047, #4716 ) ;
#25453=CARTESIAN_POINT ( 'NONE',  ( -53.65397596840620764, 15.31786685697163897, 0.6615342354323947571 ) ) ;
#25456=CARTESIAN_POINT ( 'NONE',  ( -50.64083584635693569, 22.17031203569813513, -1.070075483901071409E-14 ) ) ;
#25459=ORIENTED_EDGE ( 'NONE', *, *, #25098, .F. ) ;
#25462=AXIS2_PLACEMENT_3D ( 'NONE', #39370, #20375, #37017 ) ;
#25471=FACE_OUTER_BOUND ( 'NONE', #26664, .T. ) ;
#25475=CARTESIAN_POINT ( 'NONE',  ( -58.35793580214877352, -0.2667336269367078794, -0.1357860315391856976 ) ) ;
#25488=VERTEX_POINT ( 'NONE', #36157 ) ;
#25490=DIRECTION ( 'NONE',  ( 0.000000000000000000, 0.000000000000000000, -1.000000000000000000 ) ) ;
#25499=ORIENTED_EDGE ( 'NONE', *, *, #35780, .F. ) ;
#25501=CARTESIAN_POINT ( 'NONE',  ( -58.37116772670351850, -0.2940390518722524327, -2.603646672650065119E-13 ) ) ;
#25505=VERTEX_POINT ( 'NONE', #39562 ) ;
#25507=CARTESIAN_POINT ( 'NONE',  ( -30.53944104333574217, 56.31939948593669243, 1.269999999999994023 ) ) ;
#25514=DIRECTION ( 'NONE',  ( -5.188838149069472160E-16, 1.699382548006136559E-16, 1.000000000000000000 ) ) ;
#25520=ORIENTED_EDGE ( 'NONE', *, *, #24067, .F. ) ;
#25522=EDGE_CURVE ( 'NONE', #11267, #37307, #38377, .T. ) ;
#25524=DIRECTION ( 'NONE',  ( -5.188838149069472160E-16, 1.699382548006136559E-16, 1.000000000000000000 ) ) ;
#25527=CIRCLE ( 'NONE', #35071, 0.5080000000000000071 ) ;
#25538=CARTESIAN_POINT ( 'NONE',  ( -8.816700480405424756, 73.94613776634058411, -1.269999999999996909 ) ) ;
#25540=CARTESIAN_POINT ( 'NONE',  ( -46.52557095416602806, 23.25943309041075224, 3.047882326417268750 ) ) ;
#25541=CARTESIAN_POINT ( 'NONE',  ( -58.68165211130394709, -0.3140782993471775142, 0.3080062417138906827 ) ) ;
#25544=ORIENTED_EDGE ( 'NONE', *, *, #15680, .T. ) ;
#25549=DIRECTION ( 'NONE',  ( -0.8745520943968139171, 0.4849315768086732703, -5.271987356194193006E-16 ) ) ;
#25555=CARTESIAN_POINT ( 'NONE',  ( -18.01920641645600796, 83.84822824455466161, -1.270000000000003348 ) ) ;
#25566=EDGE_CURVE ( 'NONE', #17215, #37322, #7747, .T. ) ;
#25567=ORIENTED_EDGE ( 'NONE', *, *, #4338, .F. ) ;
#25573=CARTESIAN_POINT ( 'NONE',  ( -17.09258512000246455, 84.17916046765628835, 1.269999999999996243 ) ) ;
#25593=EDGE_CURVE ( 'NONE', #14480, #28898, #13853, .T. ) ;
#25599=FACE_OUTER_BOUND ( 'NONE', #23708, .T. ) ;
#25607=VERTEX_POINT ( 'NONE', #26556 ) ;
#25610=EDGE_LOOP ( 'NONE', ( #192, #8062, #28239, #34136, #27229 ) ) ;
#25611=DIRECTION ( 'NONE',  ( 5.188838149069472160E-16, -1.699382548006136559E-16, -1.000000000000000000 ) ) ;
#25616=CARTESIAN_POINT ( 'NONE',  ( -53.81263303816225374, 9.606026272359288853, -3.797673599996276739 ) ) ;
#25618=CARTESIAN_POINT ( 'NONE',  ( -58.54486130996896520, -0.6084878433709398626, -0.2286541811367976129 ) ) ;
#25622=DIRECTION ( 'NONE',  ( 5.188838149069472160E-16, -1.699382548006136559E-16, -1.000000000000000000 ) ) ;
#25623=ADVANCED_FACE ( 'NONE', ( #17383 ), #1222, .T. ) ;
#25626=CARTESIAN_POINT ( 'NONE',  ( -57.55343345497419705, 2.880119995625998630, -1.988856187846590018 ) ) ;
#25634=TOROIDAL_SURFACE ( 'NONE', #12039, 0.7620000000000000107, 0.2540000000000000036 ) ;
#25635=CARTESIAN_POINT ( 'NONE',  ( -41.05189575270517821, 23.09451173561986792, -5.652993304041789371E-15 ) ) ;
#25645=CARTESIAN_POINT ( 'NONE',  ( -49.01239152747368166, 15.29178156536908872, -1.600675721865278289 ) ) ;
#25646=VERTEX_POINT ( 'NONE', #4837 ) ;
#25649=CARTESIAN_POINT ( 'NONE',  ( -49.54009375067479937, 17.01946532844685223, 5.019578552719032416 ) ) ;
#25652=CARTESIAN_POINT ( 'NONE',  ( -54.22526503003591358, 12.24891082007571086, 1.741649939400648606 ) ) ;
#25656=CARTESIAN_POINT ( 'NONE',  ( -55.34794038087419210, 7.786537553440359360, -3.264576684945873275 ) ) ;
#25659=ORIENTED_EDGE ( 'NONE', *, *, #39143, .F. ) ;
#25671=DIRECTION ( 'NONE',  ( -0.9511648638205115747, -0.3086833358529540439, -8.537024980200888871E-16 ) ) ;
#25672=DIRECTION ( 'NONE',  ( 5.188838149069472160E-16, -1.699382548006136559E-16, -1.000000000000000000 ) ) ;
#25675=ORIENTED_EDGE ( 'NONE', *, *, #20890, .F. ) ;
#25676=CARTESIAN_POINT ( 'NONE',  ( -58.36413812860618577, -0.2797192912122439812, -0.09355837775955268276 ) ) ;
#25684=AXIS2_PLACEMENT_3D ( 'NONE', #36896, #20883, #7290 ) ;
#25688=CARTESIAN_POINT ( 'NONE',  ( -17.14500000000466784, 71.11999999999886768, -1.524000000000000909 ) ) ;
#25689=CARTESIAN_POINT ( 'NONE',  ( -45.45367893016184979, 22.54667639846615046, -3.012003376585093317 ) ) ;
#25690=VERTEX_POINT ( 'NONE', #18205 ) ;
#25707=CARTESIAN_POINT ( 'NONE',  ( -30.29872984418086901, 56.23795811436772851, 1.523999999999994248 ) ) ;
#25712=LINE ( 'NONE', #9528, #29637 ) ;
#25713=DIRECTION ( 'NONE',  ( 5.188838149069472160E-16, -1.699382548006136559E-16, -1.000000000000000000 ) ) ;
#25724=ORIENTED_EDGE ( 'NONE', *, *, #36656, .F. ) ;
#25732=CARTESIAN_POINT ( 'NONE',  ( -7.917360960270791281, 70.00264313970245666, -1.269999999999995799 ) ) ;
#25741=CARTESIAN_POINT ( 'NONE',  ( -44.96292901393739783, 21.56701576681934540, 3.486870777078499017 ) ) ;
#25744=CARTESIAN_POINT ( 'NONE',  ( -58.36439606173801309, -0.2818266832427390733, -0.2195612235341928287 ) ) ;
#25752=CIRCLE ( 'NONE', #13518, 0.2539999999999942859 ) ;
#25753=DIRECTION ( 'NONE',  ( -5.188838149069471174E-16, 1.699382548006136313E-16, 1.000000000000000000 ) ) ;
#25755=DIRECTION ( 'NONE',  ( 0.8745520943968251304, -0.4849315768086535638, -5.653143757709532409E-15 ) ) ;
#25757=LINE ( 'NONE', #33372, #12436 ) ;
#25765=ORIENTED_EDGE ( 'NONE', *, *, #13703, .F. ) ;
#25766=LINE ( 'NONE', #19369, #19929 ) ;
#25771=ORIENTED_EDGE ( 'NONE', *, *, #17307, .T. ) ;
#25784=ORIENTED_EDGE ( 'NONE', *, *, #9101, .F. ) ;
#25785=DIRECTION ( 'NONE',  ( -5.188838149069472160E-16, 1.699382548006136559E-16, 1.000000000000000000 ) ) ;
#25786=AXIS2_PLACEMENT_3D ( 'NONE', #3997, #4202, #4623 ) ;
#25788=CIRCLE ( 'NONE', #31915, 0.2539999999999989488 ) ;
#25789=DIRECTION ( 'NONE',  ( -0.8745520943968252414, 0.4849315768086529532, -5.691349986800548865E-16 ) ) ;
#25796=DIRECTION ( 'NONE',  ( -0.1906721105965138718, 0.9816537812491076265, -2.657572025465751014E-16 ) ) ;
#25811=CIRCLE ( 'NONE', #4771, 0.2540000000000057767 ) ;
#25821=CARTESIAN_POINT ( 'NONE',  ( -58.14663602181426683, 0.7450421216238902744, -1.200248684312827496 ) ) ;
#25823=CARTESIAN_POINT ( 'NONE',  ( -58.10259267898851476, 0.2821446311931097295, -0.7168088428569907578 ) ) ;
#25826=DIRECTION ( 'NONE',  ( -0.9816537812491076265, -0.1906721105965138718, -4.769617732184456426E-16 ) ) ;
#25829=CARTESIAN_POINT ( 'NONE',  ( -58.33777482027510786, 1.113448835244251756, -1.208045587469442017 ) ) ;
#25830=ORIENTED_EDGE ( 'NONE', *, *, #9148, .F. ) ;
#25832=EDGE_CURVE ( 'NONE', #25646, #12982, #34007, .T. ) ;
#25834=ORIENTED_EDGE ( 'NONE', *, *, #7844, .T. ) ;
#25838=CARTESIAN_POINT ( 'NONE',  ( -46.67338572489354931, 16.85372243840488338, -7.793947694802422673E-15 ) ) ;
#25842=DIRECTION ( 'NONE',  ( 0.8745520943968249084, -0.4849315768086533418, 5.271987356194193006E-16 ) ) ;
#25845=DIRECTION ( 'NONE',  ( -5.188838149069471174E-16, 1.699382548006136313E-16, 1.000000000000000000 ) ) ;
#25848=CARTESIAN_POINT ( 'NONE',  ( -49.86808358410245745, 14.13890166617936472, -1.547476669397169546 ) ) ;
#25849=CARTESIAN_POINT ( 'NONE',  ( -30.15642192025596202, 71.36377005712995469, 1.269999999999991580 ) ) ;
#25850=CARTESIAN_POINT ( 'NONE',  ( -46.75046525359888960, 25.87185527623879366, -1.402209946078870173 ) ) ;
#25851=CARTESIAN_POINT ( 'NONE',  ( -54.48477107295269661, 8.311058014251186066, 3.524008549750177188 ) ) ;
#25853=EDGE_CURVE ( 'NONE', #35981, #13983, #41070, .T. ) ;
#25855=DIRECTION ( 'NONE',  ( 0.6559537821943227653, -0.7548010569845297058, 4.686333752532403923E-16 ) ) ;
#25856=CARTESIAN_POINT ( 'NONE',  ( -56.90132276708389725, 4.901539372897764757, 1.453963793661417370 ) ) ;
#25857=CARTESIAN_POINT ( 'NONE',  ( -57.97566020452313040, 1.918554019021911916, 1.632400077439698061 ) ) ;
#25860=ORIENTED_EDGE ( 'NONE', *, *, #17757, .F. ) ;
#25861=CARTESIAN_POINT ( 'NONE',  ( -54.34407705511657127, 12.44913727002957415, -1.242021477015530451 ) ) ;
#25865=CIRCLE ( 'NONE', #31304, 0.3810000000000015041 ) ;
#25875=CARTESIAN_POINT ( 'NONE',  ( -10.44685452804832160, 82.62549350906336088, 1.269999999999998908 ) ) ;
#25877=ORIENTED_EDGE ( 'NONE', *, *, #37318, .T. ) ;
#25886=AXIS2_PLACEMENT_3D ( 'NONE', #17151, #30151, #993 ) ;
#25894=CARTESIAN_POINT ( 'NONE',  ( -46.52557095416602806, 23.25943309041075224, -3.047882326417284293 ) ) ;
#25901=CARTESIAN_POINT ( 'NONE',  ( -8.723850037987372019, 68.58388863026053173, -1.269999999999996021 ) ) ;
#25905=B_SPLINE_CURVE_WITH_KNOTS ( 'NONE', 3,
 ( #25635, #19650, #16459, #36080, #6895, #16244, #25838, #12443, #32453, #9449, #13060, #42057, #39061, #41850, #35442, #26260, #19023, #22625, #6268, #19238, #29038, #32248, #26049, #6064, #12648, #9863, #2660, #32031, #28837 ),
 .UNSPECIFIED., .F., .F.,
 ( 4, 1, 1, 1, 1, 1, 1, 2, 1, 1, 1, 1, 1, 1, 1, 1, 1, 1, 1, 1, 1, 1, 1, 1, 1, 4 ),
 ( 0.000000000000000000, 0.03307066603948304734, 0.06614133207896609468, 0.09921199811844919059, 0.1653533301974152714, 0.1984239962368983812, 0.2314946622763813522, 0.2645653283158643787, 0.3105299952961229071, 0.3564946622763812689, 0.4024593292566397418, 0.4484239962368982702, 0.5403533301974150493, 0.6322826641579321061, 0.7242119981184491628, 0.7701766650987074136, 0.8161413320789658865, 0.8850883325493537068, 0.8965794992944182695, 0.9080706660394826102, 0.9195618327845473949, 0.9310529995296121797, 0.9425441662746769644, 0.9540353330197415271, 0.9770176665098706525, 1.000000000000000000 ),
 .UNSPECIFIED. ) ;
#25908=DIRECTION ( 'NONE',  ( 0.3256999990547864710, 0.9454731675810330582, 1.565722810161054351E-16 ) ) ;
#25911=ORIENTED_EDGE ( 'NONE', *, *, #35344, .T. ) ;
#25916=CARTESIAN_POINT ( 'NONE',  ( -24.57769139521899149, 76.70147894597536720, 1.269999999999993578 ) ) ;
#25918=ORIENTED_EDGE ( 'NONE', *, *, #9662, .T. ) ;
#25926=FACE_OUTER_BOUND ( 'NONE', #9183, .T. ) ;
#25938=DIRECTION ( 'NONE',  ( 0.1906721105965186736, -0.9816537812491066273, 0.000000000000000000 ) ) ;
#25939=DIRECTION ( 'NONE',  ( 0.1565721916417968096, 0.9876665170007964401, 0.000000000000000000 ) ) ;
#25944=EDGE_CURVE ( 'NONE', #39773, #20108, #39035, .T. ) ;
#25948=CARTESIAN_POINT ( 'NONE',  ( -46.77796495209232575, 25.80132671658136090, 1.441379436031522410 ) ) ;
#25949=CARTESIAN_POINT ( 'NONE',  ( -47.29859047510723258, 25.70208046547991287, 0.1062880809757735939 ) ) ;
#25951=ADVANCED_FACE ( 'NONE', ( #2689 ), #9478, .T. ) ;
#25952=CARTESIAN_POINT ( 'NONE',  ( -47.20791569504335428, 21.28685671521062517, 4.803936552638831792 ) ) ;
#25953=DIRECTION ( 'NONE',  ( -0.8745520943968235761, 0.4849315768086558398, -4.268512490100410909E-16 ) ) ;
#25955=CARTESIAN_POINT ( 'NONE',  ( -58.37241122568488549, -0.2962816677227891882, -1.035588846938697759E-14 ) ) ;
#25966=CARTESIAN_POINT ( 'NONE',  ( -8.473844426907701788, 67.77203500197072117, -1.523999999999995802 ) ) ;
#25976=DIRECTION ( 'NONE',  ( -0.8745520943968249084, 0.4849315768086533418, -5.311926654347176508E-16 ) ) ;
#25981=AXIS2_PLACEMENT_3D ( 'NONE', #27548, #27336, #11142 ) ;
#25983=ORIENTED_EDGE ( 'NONE', *, *, #12591, .F. ) ;
#25985=CARTESIAN_POINT ( 'NONE',  ( -46.67338572489354931, 16.85372243840488338, -6.574220250756231762E-15 ) ) ;
#25991=DIRECTION ( 'NONE',  ( 0.4849315768086534528, 0.8745520943968250194, 1.030032898892974942E-16 ) ) ;
#25995=ORIENTED_EDGE ( 'NONE', *, *, #6887, .F. ) ;
#25996=AXIS2_PLACEMENT_3D ( 'NONE', #4142, #24123, #946 ) ;
#25997=CARTESIAN_POINT ( 'NONE',  ( -20.79116009376201646, 79.67004825550966984, 1.269999999999995133 ) ) ;
#25998=CARTESIAN_POINT ( 'NONE',  ( -20.79116009376201646, 79.67004825550966984, 1.523999999999995358 ) ) ;
#25999=CARTESIAN_POINT ( 'NONE',  ( -58.73303099470203392, -0.3138845496159919923, 0.2515151591903359574 ) ) ;
#26007=EDGE_CURVE ( 'NONE', #7000, #28177, #15879, .T. ) ;
#26013=DIRECTION ( 'NONE',  ( 0.8745520943968235761, -0.4849315768086558398, 8.537024980200821818E-16 ) ) ;
#26022=CIRCLE ( 'NONE', #34193, 0.2540000000000000036 ) ;
#26023=VERTEX_POINT ( 'NONE', #38251 ) ;
#26025=ORIENTED_EDGE ( 'NONE', *, *, #24468, .F. ) ;
#26031=CARTESIAN_POINT ( 'NONE',  ( -58.55703382916102129, -0.1428860932337914225, -0.5663864201305394142 ) ) ;
#26032=ORIENTED_EDGE ( 'NONE', *, *, #25035, .T. ) ;
#26037=DIRECTION ( 'NONE',  ( -0.7770581983690896255, 0.6294287539883960392, -4.360450048231423821E-16 ) ) ;
#26040=CARTESIAN_POINT ( 'NONE',  ( -58.87911280034276018, -0.2081424763510641984, -1.061797465414398100E-14 ) ) ;
#26041=VERTEX_POINT ( 'NONE', #42086 ) ;
#26047=EDGE_CURVE ( 'NONE', #10071, #120, #18845, .T. ) ;
#26049=CARTESIAN_POINT ( 'NONE',  ( -57.47393550255003447, 1.325481720219581661, -1.020368242535414227E-14 ) ) ;
#26053=FACE_OUTER_BOUND ( 'NONE', #20428, .T. ) ;
#26058=CARTESIAN_POINT ( 'NONE',  ( -48.39470387610976587, 16.07729130905085313, -1.622931888101232678 ) ) ;
#26061=AXIS2_PLACEMENT_3D ( 'NONE', #15063, #11882, #24871 ) ;
#26062=CARTESIAN_POINT ( 'NONE',  ( -46.68342141079460106, 26.02334812023122268, -1.327713788494189862 ) ) ;
#26063=CARTESIAN_POINT ( 'NONE',  ( -47.85244527695896011, 19.39403540832957518, 5.219971639306693056 ) ) ;
#26068=CARTESIAN_POINT ( 'NONE',  ( -57.37345908981379949, 3.796002467274087078, 0.9053535129858855113 ) ) ;
#26069=CARTESIAN_POINT ( 'NONE',  ( -57.64973313486724038, 1.352533784701764885, 1.499908592384902706 ) ) ;
#26070=EDGE_CURVE ( 'NONE', #22433, #30888, #3531, .T. ) ;
#26073=ORIENTED_EDGE ( 'NONE', *, *, #36656, .T. ) ;
#26074=CARTESIAN_POINT ( 'NONE',  ( -51.09183723991096571, 15.73968240350219538, -4.743875354843006598 ) ) ;
#26077=DIRECTION ( 'NONE',  ( -5.188838149069471174E-16, 1.699382548006136313E-16, 1.000000000000000000 ) ) ;
#26090=ORIENTED_EDGE ( 'NONE', *, *, #26205, .T. ) ;
#26105=ORIENTED_EDGE ( 'NONE', *, *, #19897, .F. ) ;
#26108=CARTESIAN_POINT ( 'NONE',  ( -28.09515292912719175, 77.51021392068167870, -1.270000000000007345 ) ) ;
#26109=EDGE_CURVE ( 'NONE', #16254, #33959, #11136, .T. ) ;
#26110=CARTESIAN_POINT ( 'NONE',  ( -44.36446822842629700, 21.81554158013422651, -2.896954608336749892 ) ) ;
#26116=AXIS2_PLACEMENT_3D ( 'NONE', #33770, #26526, #26740 ) ;
#26121=CARTESIAN_POINT ( 'NONE',  ( -47.59458007651616640, 19.66657808744393066, -5.176039278150066814 ) ) ;
#26122=TOROIDAL_SURFACE ( 'NONE', #9793, 0.3810000000000000608, 0.2540000000000000036 ) ;
#26123=AXIS2_PLACEMENT_3D ( 'NONE', #16345, #19745, #6360 ) ;
#26127=VERTEX_POINT ( 'NONE', #16490 ) ;
#26133=CARTESIAN_POINT ( 'NONE',  ( -32.35036891424130090, 51.35816619018828533, 1.523999999999994692 ) ) ;
#26135=ORIENTED_EDGE ( 'NONE', *, *, #26690, .T. ) ;
#26138=CARTESIAN_POINT ( 'NONE',  ( -17.82828877264048373, 64.92754330167842625, -1.270000000000000018 ) ) ;
#26140=EDGE_CURVE ( 'NONE', #22436, #30491, #22677, .T. ) ;
#26163=CARTESIAN_POINT ( 'NONE',  ( -46.63086599321469095, 26.12812040998877450, 1.284766365014880840 ) ) ;
#26164=CARTESIAN_POINT ( 'NONE',  ( -49.54051387650593341, 20.87470723125096228, 2.270501476849533518 ) ) ;
#26166=CARTESIAN_POINT ( 'NONE',  ( -53.75224695799815322, 9.373383622779334345, 3.688627211158417296 ) ) ;
#26167=CARTESIAN_POINT ( 'NONE',  ( -58.82991074935231524, -0.2577531494038359794, -1.058401375502683064E-14 ) ) ;
#26169=CARTESIAN_POINT ( 'NONE',  ( -58.37241122568487128, -0.2962816677227614326, -1.020154024344285766E-14 ) ) ;
#26170=ORIENTED_EDGE ( 'NONE', *, *, #33993, .T. ) ;
#26174=CARTESIAN_POINT ( 'NONE',  ( -47.29859047510723258, 25.70208046547991287, -0.1062880809757916212 ) ) ;
#26195=ORIENTED_EDGE ( 'NONE', *, *, #7941, .T. ) ;
#26196=CARTESIAN_POINT ( 'NONE',  ( -43.13073682054402269, 20.84535665847938546, -5.417716557342317191E-15 ) ) ;
#26199=AXIS2_PLACEMENT_3D ( 'NONE', #36207, #39400, #1062 ) ;
#26204=CARTESIAN_POINT ( 'NONE',  ( -7.917360960270791281, 70.00264313970245666, -1.523999999999995802 ) ) ;
#26205=EDGE_CURVE ( 'NONE', #38326, #34680, #26784, .T. ) ;
#26213=CARTESIAN_POINT ( 'NONE',  ( -58.76944392236323012, -0.3049061203703323786, 0.2000781065762422262 ) ) ;
#26225=DIRECTION ( 'NONE',  ( -5.188838149069471174E-16, 1.699382548006136313E-16, 1.000000000000000000 ) ) ;
#26226=DIRECTION ( 'NONE',  ( 5.188838149069472160E-16, -1.699382548006136559E-16, -1.000000000000000000 ) ) ;
#26234=ORIENTED_EDGE ( 'NONE', *, *, #19071, .F. ) ;
#26237=DIRECTION ( 'NONE',  ( 0.01731298258486638209, -0.9998501190848636533, 0.000000000000000000 ) ) ;
#26242=CARTESIAN_POINT ( 'NONE',  ( -58.61964679745516094, -0.2719338414218400723, -0.4055338230047252912 ) ) ;
#26243=ORIENTED_EDGE ( 'NONE', *, *, #15372, .F. ) ;
#26244=DIRECTION ( 'NONE',  ( 0.7308269722843605543, -0.6825627711659012498, 8.537024980200792236E-16 ) ) ;
#26248=CARTESIAN_POINT ( 'NONE',  ( -44.39753764704820327, 21.50835213917398647, 3.136200482385998800 ) ) ;
#26251=CARTESIAN_POINT ( 'NONE',  ( -57.67794393518098417, 1.927849678527493449, -1.763631237166056520 ) ) ;
#26252=ORIENTED_EDGE ( 'NONE', *, *, #40223, .T. ) ;
#26260=CARTESIAN_POINT ( 'NONE',  ( -54.22787649382025421, 6.886497292746610377, -9.681224659302749425E-15 ) ) ;
#26267=CARTESIAN_POINT ( 'NONE',  ( -47.30388380253317138, 17.78501317193704168, -2.251402236601650397 ) ) ;
#26271=CARTESIAN_POINT ( 'NONE',  ( -46.68142054004553643, 26.02750436334470052, -1.325888764026806665 ) ) ;
#26272=FACE_OUTER_BOUND ( 'NONE', #35275, .T. ) ;
#26273=CARTESIAN_POINT ( 'NONE',  ( -30.15519950990045572, 69.97033940222173953, -1.524000000000010457 ) ) ;
#26275=DIRECTION ( 'NONE',  ( 5.188838149069472160E-16, -1.699382548006136559E-16, -1.000000000000000000 ) ) ;
#26276=CARTESIAN_POINT ( 'NONE',  ( -16.71197878298170991, 83.87086364642222236, 1.523999999999996691 ) ) ;
#26277=CARTESIAN_POINT ( 'NONE',  ( -56.91937565786325592, 5.591339438888994984, 0.1632292574589306045 ) ) ;
#26278=AXIS2_PLACEMENT_3D ( 'NONE', #7085, #20677, #24089 ) ;
#26279=CARTESIAN_POINT ( 'NONE',  ( -58.33777482027510786, 1.113448835244251756, 1.208045587469420701 ) ) ;
#26283=CARTESIAN_POINT ( 'NONE',  ( -52.32205026661357294, 13.67230311332622072, -4.407798173677540454 ) ) ;
#26285=ORIENTED_EDGE ( 'NONE', *, *, #7752, .F. ) ;
#26286=CARTESIAN_POINT ( 'NONE',  ( -8.336765840796966032, 73.19241104973453105, -1.269999999999996687 ) ) ;
#26297=CARTESIAN_POINT ( 'NONE',  ( -11.34554992887676228, 77.73165686004496422, -1.523999999999998911 ) ) ;
#26300=ORIENTED_EDGE ( 'NONE', *, *, #7190, .F. ) ;
#26302=CARTESIAN_POINT ( 'NONE',  ( -58.36917081973859922, -0.2902516154645916058, -0.03021462763837517995 ) ) ;
#26308=EDGE_CURVE ( 'NONE', #20372, #36001, #32224, .T. ) ;
#26309=DIRECTION ( 'NONE',  ( 5.188838149069472160E-16, -1.699382548006136559E-16, -1.000000000000000000 ) ) ;
#26316=CIRCLE ( 'NONE', #24947, 2.857500000000000817 ) ;
#26318=CARTESIAN_POINT ( 'NONE',  ( -46.07906060731711761, 24.80782705053048076, -1.769089518196001798 ) ) ;
#26330=VECTOR ( 'NONE', #12261, 1000.000000000000227 ) ;
#26331=EDGE_CURVE ( 'NONE', #5685, #17866, #1653, .T. ) ;
#26336=AXIS2_PLACEMENT_3D ( 'NONE', #18257, #31261, #15696 ) ;
#26340=CARTESIAN_POINT ( 'NONE',  ( -17.14500000000466784, 71.11999999999886768, 1.269999999999998241 ) ) ;
#26347=AXIS2_PLACEMENT_3D ( 'NONE', #27085, #10679, #26875 ) ;
#26351=DIRECTION ( 'NONE',  ( -0.3582377630123916856, 0.9336303900108853249, -3.445432962228668055E-16 ) ) ;
#26352=CARTESIAN_POINT ( 'NONE',  ( -8.690931667554782081, 74.34623700195145091, 1.270000000000002238 ) ) ;
#26363=EDGE_CURVE ( 'NONE', #34378, #20421, #3686, .T. ) ;
#26366=PLANE ( 'NONE',  #41283 ) ;
#26373=CARTESIAN_POINT ( 'NONE',  ( -48.81378120017792099, 18.07100238705057649, 5.105379834343001910 ) ) ;
#26374=CARTESIAN_POINT ( 'NONE',  ( -47.91489772873670461, 20.73163290703075745, 4.601312741204995227 ) ) ;
#26376=CARTESIAN_POINT ( 'NONE',  ( -50.82551848962686591, 16.13924203555649228, 4.804203053272154911 ) ) ;
#26377=CARTESIAN_POINT ( 'NONE',  ( -58.71329930298021083, -0.3143398509990111278, 0.2746998690518271946 ) ) ;
#26379=B_SPLINE_CURVE_WITH_KNOTS ( 'NONE', 3,
 ( #7348, #20941, #27349, #10322, #17337, #14339, #24142, #17126, #36735, #29707, #33548, #30127, #1381, #4379, #7972, #23291, #16917, #13935, #33966, #13523 ),
 .UNSPECIFIED., .F., .F.,
 ( 4, 2, 2, 2, 2, 2, 2, 2, 2, 4 ),
 ( -5.999999999384015929E-08, 0.002615939326670506469, 0.005231938653341007377, 0.007847937980011505249, 0.01046393730668200746, 0.01307993663335250793, 0.01438793629668775817, 0.01569593596002300667, 0.01831193528669351062, 0.02092793461336401456 ),
 .UNSPECIFIED. ) ;
#26381=CARTESIAN_POINT ( 'NONE',  ( -23.43300365160793319, 82.12916405548841681, 1.523999999999993360 ) ) ;
#26382=VERTEX_POINT ( 'NONE', #7454 ) ;
#26383=CARTESIAN_POINT ( 'NONE',  ( -47.19936399096372526, 20.24790404726484283, 5.251082349106850344 ) ) ;
#26384=EDGE_CURVE ( 'NONE', #32222, #1192, #11053, .T. ) ;
#26391=ADVANCED_FACE ( 'NONE', ( #30433 ), #32724, .T. ) ;
#26406=AXIS2_PLACEMENT_3D ( 'NONE', #35756, #38739, #6571 ) ;
#26408=EDGE_LOOP ( 'NONE', ( #23662, #16935, #12461, #4797 ) ) ;
#26410=CARTESIAN_POINT ( 'NONE',  ( -46.67338572489352089, 16.85372243840493311, 0.3683569569372045494 ) ) ;
#26417=DIRECTION ( 'NONE',  ( -0.4849315768086535638, -0.8745520943968251304, -1.030032898892975065E-16 ) ) ;
#26421=ORIENTED_EDGE ( 'NONE', *, *, #33993, .F. ) ;
#26426=DIRECTION ( 'NONE',  ( -0.8745520943968466687, 0.4849315768086143730, -6.829619984160688614E-16 ) ) ;
#26431=CIRCLE ( 'NONE', #17606, 0.5080000000000030047 ) ;
#26440=DIRECTION ( 'NONE',  ( -0.8745520943968250194, 0.4849315768086535083, -5.424246918827963022E-16 ) ) ;
#26445=DIRECTION ( 'NONE',  ( 5.188838149069472160E-16, -1.699382548006136559E-16, -1.000000000000000000 ) ) ;
#26450=EDGE_CURVE ( 'NONE', #34427, #35121, #14237, .T. ) ;
#26454=VERTEX_POINT ( 'NONE', #37252 ) ;
#26460=CARTESIAN_POINT ( 'NONE',  ( -58.78715887833730847, -0.2958247752677126141, -0.1682579856030674004 ) ) ;
#26461=ORIENTED_EDGE ( 'NONE', *, *, #31687, .T. ) ;
#26465=LINE ( 'NONE', #23889, #9599 ) ;
#26470=CARTESIAN_POINT ( 'NONE',  ( -58.37241122568488549, -0.2962816677227753104, -0.2416009568454014489 ) ) ;
#26471=ORIENTED_EDGE ( 'NONE', *, *, #19395, .T. ) ;
#26474=ORIENTED_EDGE ( 'NONE', *, *, #38908, .T. ) ;
#26478=CARTESIAN_POINT ( 'NONE',  ( -56.37342374758031127, 3.980281407817698458, 2.237022232197619864 ) ) ;
#26484=CARTESIAN_POINT ( 'NONE',  ( -5.369399562154598904, 64.90898011766716991, -1.269999999999993578 ) ) ;
#26487=CARTESIAN_POINT ( 'NONE',  ( -51.51920269172890698, 12.50394502492935978, -2.730133853924327170 ) ) ;
#26490=DIRECTION ( 'NONE',  ( 5.188838149069472160E-16, -1.699382548006136559E-16, -1.000000000000000000 ) ) ;
#26491=CARTESIAN_POINT ( 'NONE',  ( -10.55305098051677248, 77.31887769575739355, -1.269999999999998241 ) ) ;
#26492=DIRECTION ( 'NONE',  ( -5.188838149069471174E-16, 1.699382548006136313E-16, 1.000000000000000000 ) ) ;
#26495=CARTESIAN_POINT ( 'NONE',  ( -29.82321757229076908, 71.17901112636586447, 1.269999999999991802 ) ) ;
#26496=DIRECTION ( 'NONE',  ( 0.7548010569845216011, 0.6559537821943317581, 2.801824109679580762E-16 ) ) ;
#26497=CARTESIAN_POINT ( 'NONE',  ( -58.60381103753274346, 0.5214191424347813797, 0.2072982876684393294 ) ) ;
#26498=CARTESIAN_POINT ( 'NONE',  ( -57.00508801794419611, 2.691366720778187727, 1.977812201481533583 ) ) ;
#26500=ORIENTED_EDGE ( 'NONE', *, *, #72, .F. ) ;
#26501=CARTESIAN_POINT ( 'NONE',  ( -54.22526503003591358, 12.24891082007571086, -1.741649939400669478 ) ) ;
#26503=VERTEX_POINT ( 'NONE', #40667 ) ;
#26517=VERTEX_POINT ( 'NONE', #8277 ) ;
#26520=CARTESIAN_POINT ( 'NONE',  ( -57.92026434645431010, 0.6774725698580426059, -0.9613144842853563743 ) ) ;
#26526=DIRECTION ( 'NONE',  ( -0.1951894777626509980, -0.9807655518882909540, 3.317599696243019336E-15 ) ) ;
#26527=AXIS2_PLACEMENT_3D ( 'NONE', #23103, #23738, #36758 ) ;
#26537=CARTESIAN_POINT ( 'NONE',  ( -51.02479983779974049, 14.46739584830851477, -4.600955224801065668 ) ) ;
#26545=CARTESIAN_POINT ( 'NONE',  ( -42.04985097881030498, 22.19100705996983436, -1.479702663569509413 ) ) ;
#26546=VERTEX_POINT ( 'NONE', #21875 ) ;
#26548=UNCERTAINTY_MEASURE_WITH_UNIT (LENGTH_MEASURE( 1.000000000000000082E-05 ), #7512, 'distance_accuracy_value', 'NONE');
#26550=ORIENTED_EDGE ( 'NONE', *, *, #8135, .T. ) ;
#26556=CARTESIAN_POINT ( 'NONE',  ( -7.868930244179279221, 69.75330307926518003, -1.269999999999995799 ) ) ;
#26558=EDGE_LOOP ( 'NONE', ( #32132, #35846, #32357, #41104 ) ) ;
#26566=DIRECTION ( 'NONE',  ( 0.9336303900108928744, 0.3582377630123714241, 0.000000000000000000 ) ) ;
#26571=ORIENTED_EDGE ( 'NONE', *, *, #16805, .T. ) ;
#26574=AXIS2_PLACEMENT_3D ( 'NONE', #18762, #8566, #38590 ) ;
#26575=CARTESIAN_POINT ( 'NONE',  ( -8.438477507926631205, 69.62414081991882142, -1.269999999999996021 ) ) ;
#26577=ORIENTED_EDGE ( 'NONE', *, *, #2142, .T. ) ;
#26580=CARTESIAN_POINT ( 'NONE',  ( -46.95911617132933458, 24.98948415085536823, -1.986615011824472088 ) ) ;
#26584=ADVANCED_FACE ( 'NONE', ( #22086 ), #5516, .T. ) ;
#26587=CARTESIAN_POINT ( 'NONE',  ( -49.16877686933415248, 17.52905763403498085, 5.029729607253535129 ) ) ;
#26588=CARTESIAN_POINT ( 'NONE',  ( -47.99264284736476327, 22.55967899981254376, 2.517363275470459794 ) ) ;
#26589=AXIS2_PLACEMENT_3D ( 'NONE', #35913, #10118, #2906 ) ;
#26591=CARTESIAN_POINT ( 'NONE',  ( -53.65759266121656879, 11.01975743955735432, 4.003319250743206936 ) ) ;
#26592=CARTESIAN_POINT ( 'NONE',  ( -58.29986746207860904, 0.4137999759807384215, 1.006442112984123227 ) ) ;
#26597=ORIENTED_EDGE ( 'NONE', *, *, #8405, .F. ) ;
#26598=CARTESIAN_POINT ( 'NONE',  ( -44.13308345971568514, 24.21351174012166396, 1.567149544246648762 ) ) ;
#26608=CARTESIAN_POINT ( 'NONE',  ( -17.14500000000466784, 71.11999999999886768, 1.269999999999998241 ) ) ;
#26620=CARTESIAN_POINT ( 'NONE',  ( -45.30933510662926977, 19.89173180141312614, 2.333898071402933816 ) ) ;
#26623=EDGE_CURVE ( 'NONE', #25646, #21812, #38826, .T. ) ;
#26627=CARTESIAN_POINT ( 'NONE',  ( -17.22465686008793995, 48.97870818484556565, -1.269999999999997131 ) ) ;
#26628=CIRCLE ( 'NONE', #40896, 0.2540000000000045555 ) ;
#26633=ORIENTED_EDGE ( 'NONE', *, *, #38625, .F. ) ;
#26635=DIRECTION ( 'NONE',  ( -0.8745520943968235761, 0.4849315768086558398, -5.691349986800547879E-16 ) ) ;
#26636=EDGE_CURVE ( 'NONE', #20372, #32706, #15453, .T. ) ;
#26637=CIRCLE ( 'NONE', #35496, 0.2540000000000010583 ) ;
#26654=VECTOR ( 'NONE', #32897, 1000.000000000000114 ) ;
#26656=CARTESIAN_POINT ( 'NONE',  ( -10.12396263145945774, 65.41168055974398499, 1.270000000000002904 ) ) ;
#26657=CARTESIAN_POINT ( 'NONE',  ( -15.27962295839633811, 80.49293118800726177, -1.524000000000001576 ) ) ;
#26662=ORIENTED_EDGE ( 'NONE', *, *, #15232, .T. ) ;
#26663=LINE ( 'NONE', #39671, #28391 ) ;
#26664=EDGE_LOOP ( 'NONE', ( #26025, #27801, #19276, #12889 ) ) ;
#26671=EDGE_CURVE ( 'NONE', #34241, #20108, #40215, .T. ) ;
#26678=EDGE_CURVE ( 'NONE', #13951, #6380, #23853, .T. ) ;
#26682=VERTEX_POINT ( 'NONE', #24612 ) ;
#26687=EDGE_CURVE ( 'NONE', #11397, #39243, #8228, .T. ) ;
#26688=DIRECTION ( 'NONE',  ( 5.188838149069472160E-16, -1.699382548006136559E-16, -1.000000000000000000 ) ) ;
#26689=CIRCLE ( 'NONE', #8319, 0.3809999999999984510 ) ;
#26690=EDGE_CURVE ( 'NONE', #7253, #18068, #9556, .T. ) ;
#26692=CARTESIAN_POINT ( 'NONE',  ( -48.43799250123541356, 18.62746361536937911, 5.176101822176825351 ) ) ;
#26699=CARTESIAN_POINT ( 'NONE',  ( -30.45812239790965492, 71.16801738242446618, -1.524000000000007793 ) ) ;
#26701=CARTESIAN_POINT ( 'NONE',  ( -50.52646075385809610, 14.05410990099204049, -2.888145277534023947 ) ) ;
#26708=CARTESIAN_POINT ( 'NONE',  ( -46.95911617132934879, 24.98948415085533270, 1.986615011824473864 ) ) ;
#26709=CARTESIAN_POINT ( 'NONE',  ( -33.20758249455312239, 49.81222039523557044, 1.523999999999993804 ) ) ;
#26710=CARTESIAN_POINT ( 'NONE',  ( -58.73915225836901044, 0.1638436772961188170, -1.071698628919754437E-14 ) ) ;
#26711=CARTESIAN_POINT ( 'NONE',  ( -57.26626398570029863, 3.526386058942967860, 2.205039086913747948 ) ) ;
#26714=CARTESIAN_POINT ( 'NONE',  ( -56.91937565786339803, 5.591339438888828894, -1.085802076254212195E-14 ) ) ;
#26716=EDGE_LOOP ( 'NONE', ( #11481, #32902, #7488, #13143 ) ) ;
#26733=CARTESIAN_POINT ( 'NONE',  ( -57.76243589657412514, 1.018525044351360709, -1.139292060318100042 ) ) ;
#26739=VECTOR ( 'NONE', #31888, 1000.000000000000000 ) ;
#26740=DIRECTION ( 'NONE',  ( -0.9807655518882955059, 0.1951894777626270172, -8.537024980200854359E-16 ) ) ;
#26749=EDGE_CURVE ( 'NONE', #27753, #32986, #16357, .T. ) ;
#26750=CARTESIAN_POINT ( 'NONE',  ( -53.65759266121656879, 11.01975743955735432, -4.003319250743225588 ) ) ;
#26753=FACE_OUTER_BOUND ( 'NONE', #17292, .T. ) ;
#26759=CARTESIAN_POINT ( 'NONE',  ( -9.795036404550216957, 65.29837086945681790, -1.269999999999996021 ) ) ;
#26760=ORIENTED_EDGE ( 'NONE', *, *, #32338, .T. ) ;
#26761=LINE ( 'NONE', #39554, #11329 ) ;
#26762=CIRCLE ( 'NONE', #28114, 0.2539999999999978941 ) ;
#26766=CARTESIAN_POINT ( 'NONE',  ( -10.73808814597608574, 77.14487411131506178, 1.524000000000001132 ) ) ;
#26776=CARTESIAN_POINT ( 'NONE',  ( -26.29578028364076658, 73.87584665086983193, -1.270000000000006013 ) ) ;
#26781=CARTESIAN_POINT ( 'NONE',  ( -58.36601048454644314, 0.2708230324007659950, -0.9148880203699379932 ) ) ;
#26784=CIRCLE ( 'NONE', #37009, 0.2539999999999973390 ) ;
#26788=AXIS2_PLACEMENT_3D ( 'NONE', #24414, #8458, #21625 ) ;
#26791=CARTESIAN_POINT ( 'NONE',  ( -42.63057730194618244, 21.82620848986212181, 1.774738817929873758 ) ) ;
#26797=CIRCLE ( 'NONE', #17272, 0.5080000000000000071 ) ;
#26798=CARTESIAN_POINT ( 'NONE',  ( -30.08804090436192169, 69.76339842363584864, -1.270000000000007345 ) ) ;
#26806=CARTESIAN_POINT ( 'NONE',  ( -56.16595168976004970, 4.414070172726168195, 2.362198540470026309 ) ) ;
#26807=CARTESIAN_POINT ( 'NONE',  ( -47.63491852694408379, 24.04202919463459409, 1.290898778641160094 ) ) ;
#26809=CARTESIAN_POINT ( 'NONE',  ( -49.59816314059867182, 17.91649583374774224, 5.069000701391649599 ) ) ;
#26810=CARTESIAN_POINT ( 'NONE',  ( -58.59441299015681182, -0.2213268877428872239, 0.4750018593813392642 ) ) ;
#26813=VERTEX_POINT ( 'NONE', #14815 ) ;
#26814=CARTESIAN_POINT ( 'NONE',  ( -46.25688858429102623, 20.73875112231587892, 4.700046123029338219 ) ) ;
#26819=AXIS2_PLACEMENT_3D ( 'NONE', #5337, #25119, #38120 ) ;
#26825=CARTESIAN_POINT ( 'NONE',  ( -45.93641268020314783, 20.77718376654426180, 4.359287402722423543 ) ) ;
#26828=DIRECTION ( 'NONE',  ( 0.4849315768086427392, 0.8745520943968311256, 7.999751396575047988E-15 ) ) ;
#26838=CARTESIAN_POINT ( 'NONE',  ( -42.98746435103614516, 21.25571956186866984, 0.9029888148949687388 ) ) ;
#26855=CARTESIAN_POINT ( 'NONE',  ( -10.32579803928178031, 77.06797118195436269, -1.523999999999998245 ) ) ;
#26866=DIRECTION ( 'NONE',  ( 0.7770581983690878491, -0.6294287539883980376, 5.101669463485847584E-16 ) ) ;
#26868=CARTESIAN_POINT ( 'NONE',  ( -24.23745918283205114, 82.38670122043342303, -1.524000000000006461 ) ) ;
#26871=EDGE_CURVE ( 'NONE', #3266, #37307, #15691, .T. ) ;
#26875=DIRECTION ( 'NONE',  ( -0.8745520943968241312, 0.4849315768086548406, -5.691349986800536046E-16 ) ) ;
#26884=SHAPE_REPRESENTATION_RELATIONSHIP ( 'NONE' , 'NONE' ,  #22056, #41738 ) ;
#26895=CARTESIAN_POINT ( 'NONE',  ( -56.57399730107074021, 3.557946380840032674, 2.108622681941778154 ) ) ;
#26903=DIRECTION ( 'NONE',  ( -5.188838149069471174E-16, 1.699382548006136313E-16, 1.000000000000000000 ) ) ;
#26905=CARTESIAN_POINT ( 'NONE',  ( -50.84949806483947299, 11.71728973011885344, -0.3797569051948266328 ) ) ;
#26909=CARTESIAN_POINT ( 'NONE',  ( -3.831877602099685198, 71.07198261757335445, 1.270000000000005347 ) ) ;
#26910=CARTESIAN_POINT ( 'NONE',  ( -29.24397885296949440, 65.27318422236065487, -1.524000000000773181 ) ) ;
#26912=CARTESIAN_POINT ( 'NONE',  ( -28.42835727709238114, 77.69497285144578314, -1.524000000000007793 ) ) ;
#26914=CARTESIAN_POINT ( 'NONE',  ( -57.83255607995954506, 2.614142775670388996, 0.5104628509321454954 ) ) ;
#26917=ORIENTED_EDGE ( 'NONE', *, *, #7082, .T. ) ;
#26918=CARTESIAN_POINT ( 'NONE',  ( -58.05887703936295452, 1.806656698574160558, -1.362798277128405289 ) ) ;
#26923=CARTESIAN_POINT ( 'NONE',  ( -22.95370498042275642, 82.54569470718179502, 1.269999999999993356 ) ) ;
#26929=ADVANCED_FACE ( 'NONE', ( #349 ), #35483, .T. ) ;
#26935=DIRECTION ( 'NONE',  ( 5.188838149069472160E-16, -1.699382548006136559E-16, -1.000000000000000000 ) ) ;
#26939=CARTESIAN_POINT ( 'NONE',  ( -57.62437015934663265, 1.316655653385057079, -1.280333191779400082 ) ) ;
#26944=CARTESIAN_POINT ( 'NONE',  ( -46.52557095416602806, 23.25943309041075224, -3.047882326417284293 ) ) ;
#26949=VERTEX_POINT ( 'NONE', #12686 ) ;
#26952=CARTESIAN_POINT ( 'NONE',  ( -11.56352105402813280, 78.55269139521317356, -1.523999999999999133 ) ) ;
#26954=CARTESIAN_POINT ( 'NONE',  ( -54.77668461537430034, 8.146287316968315650, -3.518595155146543529 ) ) ;
#26960=AXIS2_PLACEMENT_3D ( 'NONE', #3411, #15751, #35578 ) ;
#26963=EDGE_CURVE ( 'NONE', #15388, #41065, #2813, .T. ) ;
#26971=ORIENTED_EDGE ( 'NONE', *, *, #12305, .T. ) ;
#26972=CARTESIAN_POINT ( 'NONE',  ( -47.07934102874911986, 22.98505637820354153, -3.579966862081940260 ) ) ;
#26980=CARTESIAN_POINT ( 'NONE',  ( -41.08171237912078055, 23.06270199366201368, 1.270028482464937936 ) ) ;
#26983=ORIENTED_EDGE ( 'NONE', *, *, #32173, .F. ) ;
#26986=CARTESIAN_POINT ( 'NONE',  ( -7.772068811996249771, 69.25462295839062676, 1.270000000000003570 ) ) ;
#26992=CARTESIAN_POINT ( 'NONE',  ( -50.51080154061983052, 15.37413104944036668, -4.759117110719017774 ) ) ;
#26998=TOROIDAL_SURFACE ( 'NONE', #10657, 0.3810000000000014486, 0.2540000000000000036 ) ;
#27001=CARTESIAN_POINT ( 'NONE',  ( -42.48565245465179885, 21.90714463913253240, 1.692305106577786322 ) ) ;
#27005=CARTESIAN_POINT ( 'NONE',  ( -26.01970228765382132, 72.88622078690372064, -1.524000000000005794 ) ) ;
#27014=DIRECTION ( 'NONE',  ( -0.8745520943968243532, 0.4849315768086547296, -5.361993529360573944E-16 ) ) ;
#27016=CARTESIAN_POINT ( 'NONE',  ( -57.43646543250576997, 1.720973480456895910, 1.454608885177623767 ) ) ;
#27017=CARTESIAN_POINT ( 'NONE',  ( -48.00704091872448487, 20.04541143072568232, 5.176114466449816653 ) ) ;
#27018=CARTESIAN_POINT ( 'NONE',  ( -49.39021242113546606, 17.77731941784099234, 5.290631085210035778 ) ) ;
#27019=CARTESIAN_POINT ( 'NONE',  ( -58.55448969609990684, -0.1373465052187913260, 0.5737898672011175760 ) ) ;
#27022=VECTOR ( 'NONE', #30730, 1000.000000000000000 ) ;
#27023=VERTEX_POINT ( 'NONE', #38471 ) ;
#27024=CARTESIAN_POINT ( 'NONE',  ( -47.04837031381860157, 23.61299024743492581, 3.054033755318061871 ) ) ;
#27033=DIRECTION ( 'NONE',  ( 5.188838149069472160E-16, -1.699382548006136559E-16, -1.000000000000000000 ) ) ;
#27034=CARTESIAN_POINT ( 'NONE',  ( -47.22690022493003426, 20.09066223305351784, 5.151063612125013513 ) ) ;
#27037=DIRECTION ( 'NONE',  ( -0.01731298258488772612, 0.9998501190848633202, -1.788962107505314604E-16 ) ) ;
#27046=ORIENTED_EDGE ( 'NONE', *, *, #15398, .F. ) ;
#27047=CARTESIAN_POINT ( 'NONE',  ( -48.19617591663109835, 18.61566378669634503, 4.750300018642145794 ) ) ;
#27053=VERTEX_POINT ( 'NONE', #15869 ) ;
#27059=VECTOR ( 'NONE', #277, 1000.000000000000114 ) ;
#27066=CARTESIAN_POINT ( 'NONE',  ( -30.75918919842648336, 69.77432548395512413, 1.523999999999991806 ) ) ;
#27079=DIRECTION ( 'NONE',  ( -5.188838149069472160E-16, 1.699382548006136559E-16, 1.000000000000000000 ) ) ;
#27085=CARTESIAN_POINT ( 'NONE',  ( -14.38915334913366983, 80.27078028363496287, 1.523999999999998467 ) ) ;
#27086=ORIENTED_EDGE ( 'NONE', *, *, #26671, .F. ) ;
#27087=DIRECTION ( 'NONE',  ( 5.188838149069472160E-16, -1.699382548006136559E-16, -1.000000000000000000 ) ) ;
#27092=DIRECTION ( 'NONE',  ( -0.4849315768086535083, -0.8745520943968250194, -1.030032898892975065E-16 ) ) ;
#27098=CYLINDRICAL_SURFACE ( 'NONE', #22691, 0.6350000000000014522 ) ;
#27102=ORIENTED_EDGE ( 'NONE', *, *, #37125, .T. ) ;
#27110=CIRCLE ( 'NONE', #14180, 8.794749999999993406 ) ;
#27114=CARTESIAN_POINT ( 'NONE',  ( -55.03835892454119261, 5.996057868307938854, -1.012875379724342828 ) ) ;
#27116=DIRECTION ( 'NONE',  ( 5.188838149069472160E-16, -1.699382548006136559E-16, -1.000000000000000000 ) ) ;
#27117=CARTESIAN_POINT ( 'NONE',  ( -46.86449850479133517, 25.52520254179917103, -1.615770181641761560 ) ) ;
#27118=DIRECTION ( 'NONE',  ( -0.01876124593811915112, -0.9998239923360757730, 0.000000000000000000 ) ) ;
#27119=CARTESIAN_POINT ( 'NONE',  ( -30.03903471050079688, 57.95649848187943576, -1.269999999999909424 ) ) ;
#27123=CARTESIAN_POINT ( 'NONE',  ( -58.82374062945601167, -0.06097470622967726683, 0.2234658159561953850 ) ) ;
#27124=EDGE_CURVE ( 'NONE', #21375, #20566, #13057, .T. ) ;
#27128=CARTESIAN_POINT ( 'NONE',  ( -58.03112897257378933, 1.932186039288422030, -1.137512825365928348 ) ) ;
#27129=DIRECTION ( 'NONE',  ( 5.188838149069472160E-16, -1.699382548006136559E-16, -1.000000000000000000 ) ) ;
#27132=CARTESIAN_POINT ( 'NONE',  ( -47.73297240351458015, 19.53746995444953072, -5.217258361096882346 ) ) ;
#27141=CARTESIAN_POINT ( 'NONE',  ( -52.46933349272310920, 12.09275889387806480, -4.271936536825034381 ) ) ;
#27147=CARTESIAN_POINT ( 'NONE',  ( -58.20240292368494295, 0.06644746378797894426, -0.5499427731179303835 ) ) ;
#27151=CARTESIAN_POINT ( 'NONE',  ( -47.65206802627297833, 20.46304711373551299, -5.210715034831075343 ) ) ;
#27160=EDGE_CURVE ( 'NONE', #332, #26503, #17728, .T. ) ;
#27161=CARTESIAN_POINT ( 'NONE',  ( -56.21344593158320180, 5.939860726778031896, -2.828251681716873911 ) ) ;
#27164=DIRECTION ( 'NONE',  ( -0.9998501190848634312, -0.01731298258488003436, -8.537024980200781389E-16 ) ) ;
#27167=CIRCLE ( 'NONE', #675, 0.2540000000000023350 ) ;
#27174=CARTESIAN_POINT ( 'NONE',  ( -58.36439606173801309, -0.2818266832427390733, 0.2195612235341721508 ) ) ;
#27177=CARTESIAN_POINT ( 'NONE',  ( -47.24381373535820217, 25.63803778330989047, -0.2531820549803648901 ) ) ;
#27185=DIRECTION ( 'NONE',  ( -0.1951894777626589361, -0.9807655518882891776, 6.538892540527331846E-17 ) ) ;
#27192=CARTESIAN_POINT ( 'NONE',  ( -10.34239276132902319, 65.15305678602257444, -1.523999999999996247 ) ) ;
#27193=EDGE_LOOP ( 'NONE', ( #25911, #24914, #3804, #20993 ) ) ;
#27198=CARTESIAN_POINT ( 'NONE',  ( -58.59897934080607484, -0.2308949485131245316, -0.4634499375560702239 ) ) ;
#27202=ORIENTED_EDGE ( 'NONE', *, *, #16771, .T. ) ;
#27203=EDGE_LOOP ( 'NONE', ( #30166, #34921, #39899, #4962 ) ) ;
#27207=EDGE_CURVE ( 'NONE', #22515, #29093, #29236, .T. ) ;
#27208=CARTESIAN_POINT ( 'NONE',  ( -47.72134626993259587, 19.52826264940933498, 5.191136457141920957 ) ) ;
#27215=EDGE_CURVE ( 'NONE', #18538, #26454, #8899, .T. ) ;
#27221=CARTESIAN_POINT ( 'NONE',  ( -30.45812239790965492, 71.16801738242446618, -1.270000000000007567 ) ) ;
#27223=CARTESIAN_POINT ( 'NONE',  ( -57.26722424190899829, 2.083881049937859054, 1.598295151127536062 ) ) ;
#27224=CARTESIAN_POINT ( 'NONE',  ( -29.57263912082353130, 58.75010695900488855, -1.524000000000004906 ) ) ;
#27225=CARTESIAN_POINT ( 'NONE',  ( -57.07867440696631434, 2.606095844753547830, 1.988717289889800677 ) ) ;
#27226=CARTESIAN_POINT ( 'NONE',  ( -58.27639478309521337, 0.4645451433633250860, 1.037811933420001997 ) ) ;
#27229=ORIENTED_EDGE ( 'NONE', *, *, #18869, .F. ) ;
#27230=CARTESIAN_POINT ( 'NONE',  ( -46.42538233320968288, 20.85422009098716956, 4.815137874471020041 ) ) ;
#27240=CARTESIAN_POINT ( 'NONE',  ( -46.96000079187150078, 20.35382130790558364, 5.064780906957706996 ) ) ;
#27243=CARTESIAN_POINT ( 'NONE',  ( -6.318938770521976167, 64.36956080246774548, 1.270000000000005347 ) ) ;
#27247=AXIS2_PLACEMENT_3D ( 'NONE', #4295, #39431, #26426 ) ;
#27252=EDGE_LOOP ( 'NONE', ( #24300, #3471, #15982, #20225 ) ) ;
#27253=CARTESIAN_POINT ( 'NONE',  ( -50.84949806483947299, 11.71728973011885344, 0.3797569051948097019 ) ) ;
#27265=ORIENTED_EDGE ( 'NONE', *, *, #30250, .T. ) ;
#27268=EDGE_CURVE ( 'NONE', #29626, #25154, #6211, .T. ) ;
#27271=EDGE_CURVE ( 'NONE', #12580, #28646, #28826, .T. ) ;
#27277=LINE ( 'NONE', #2356, #3164 ) ;
#27284=CARTESIAN_POINT ( 'NONE',  ( -17.14500000000466784, 71.11999999999886768, -1.524000000000000909 ) ) ;
#27288=CARTESIAN_POINT ( 'NONE',  ( -8.095114962461808616, 74.19100168833409725, 1.270000000000002460 ) ) ;
#27293=CARTESIAN_POINT ( 'NONE',  ( -7.868930244179279221, 69.75330307926518003, -1.523999999999995802 ) ) ;
#27294=EDGE_LOOP ( 'NONE', ( #38695, #27774, #717, #3944 ) ) ;
#27300=ORIENTED_EDGE ( 'NONE', *, *, #7804, .F. ) ;
#27301=ORIENTED_EDGE ( 'NONE', *, *, #5270, .T. ) ;
#27308=AXIS2_PLACEMENT_3D ( 'NONE', #15885, #12909, #13124 ) ;
#27310=CYLINDRICAL_SURFACE ( 'NONE', #9313, 0.2540000000000035008 ) ;
#27313=ORIENTED_EDGE ( 'NONE', *, *, #40749, .F. ) ;
#27317=CARTESIAN_POINT ( 'NONE',  ( -58.31893842775810555, -0.1844529990621818216, 0.2851935484600691129 ) ) ;
#27324=AXIS2_PLACEMENT_3D ( 'NONE', #7128, #20084, #3938 ) ;
#27327=DIRECTION ( 'NONE',  ( -0.8745520943968240202, 0.4849315768086553402, -6.829619984160650158E-16 ) ) ;
#27328=CARTESIAN_POINT ( 'NONE',  ( -51.67551711146813176, 11.54346324480936481, -1.411685438026464290 ) ) ;
#27331=DIRECTION ( 'NONE',  ( -0.8745520943968240202, 0.4849315768086553402, -6.829619984160650158E-16 ) ) ;
#27332=DIRECTION ( 'NONE',  ( -0.8745520943968240202, 0.4849315768086551737, -5.361993529360572958E-16 ) ) ;
#27333=CARTESIAN_POINT ( 'NONE',  ( -29.79391970823417068, 57.88946435433149418, -1.524000000000004240 ) ) ;
#27336=DIRECTION ( 'NONE',  ( 5.188838149069472160E-16, -1.699382548006136559E-16, -1.000000000000000000 ) ) ;
#27337=CARTESIAN_POINT ( 'NONE',  ( -57.90853684698413417, 2.514838786807874094, 0.1030880274588810847 ) ) ;
#27341=CARTESIAN_POINT ( 'NONE',  ( -58.08922378330620973, 1.909136410080003454, -0.4248916911265372964 ) ) ;
#27342=VERTEX_POINT ( 'NONE', #15818 ) ;
#27343=CARTESIAN_POINT ( 'NONE',  ( -45.89458612274419380, 20.88821703127394969, -4.453918368557551410 ) ) ;
#27349=CARTESIAN_POINT ( 'NONE',  ( -32.60270662228668925, 51.47373954847018496, 1.269999999999993356 ) ) ;
#27351=CARTESIAN_POINT ( 'NONE',  ( -48.71949277200916129, 18.24443030291588386, -5.160461098695489746 ) ) ;
#27352=ORIENTED_EDGE ( 'NONE', *, *, #3872, .T. ) ;
#27355=CARTESIAN_POINT ( 'NONE',  ( -57.84176729718492993, 0.8471481974509047497, -1.053121747471209346 ) ) ;
#27356=EDGE_CURVE ( 'NONE', #2001, #19344, #35420, .T. ) ;
#27360=CARTESIAN_POINT ( 'NONE',  ( -46.42538233320968288, 20.85422009098716956, -4.815137874471035140 ) ) ;
#27361=TOROIDAL_SURFACE ( 'NONE', #32808, 0.3809999999999999498, 0.2540000000000000036 ) ;
#27368=CARTESIAN_POINT ( 'NONE',  ( -19.04204117267709506, 56.84332656279845963, -1.269999999999999130 ) ) ;
#27370=ADVANCED_FACE ( 'NONE', ( #9436 ), #29307, .T. ) ;
#27371=CARTESIAN_POINT ( 'NONE',  ( -53.17586183559576085, 10.67386474145934372, -4.017225210190888518 ) ) ;
#27372=AXIS2_PLACEMENT_3D ( 'NONE', #31616, #15834, #9867 ) ;
#27378=EDGE_CURVE ( 'NONE', #3540, #41261, #22519, .T. ) ;
#27382=AXIS2_PLACEMENT_3D ( 'NONE', #10101, #29275, #17118 ) ;
#27383=CARTESIAN_POINT ( 'NONE',  ( -57.94149553976682654, 0.5275954726333825784, 0.3053296928521371800 ) ) ;
#27385=EDGE_LOOP ( 'NONE', ( #35260, #7835, #6488, #29149 ) ) ;
#27386=CARTESIAN_POINT ( 'NONE',  ( -46.60530155212504155, 26.17382724835477248, -0.2116666666666759400 ) ) ;
#27388=FACE_OUTER_BOUND ( 'NONE', #10007, .T. ) ;
#27398=EDGE_CURVE ( 'NONE', #40763, #39372, #21832, .T. ) ;
#27400=CARTESIAN_POINT ( 'NONE',  ( -42.82337701166415656, 22.05454930919483303, -2.000910692578694583 ) ) ;
#27402=DIRECTION ( 'NONE',  ( -5.188838149069471174E-16, 1.699382548006136313E-16, 1.000000000000000000 ) ) ;
#27407=CARTESIAN_POINT ( 'NONE',  ( -58.73303099469992361, -0.3138845496180736605, -0.2515151591905351314 ) ) ;
#27411=EDGE_CURVE ( 'NONE', #11774, #10192, #26628, .T. ) ;
#27416=AXIS2_PLACEMENT_3D ( 'NONE', #13253, #9842, #33069 ) ;
#27418=VERTEX_POINT ( 'NONE', #35859 ) ;
#27420=CARTESIAN_POINT ( 'NONE',  ( -5.684927786827005392, 65.51297084251929448, -1.523999999999993804 ) ) ;
#27421=CARTESIAN_POINT ( 'NONE',  ( -29.30640055155810941, 61.36565346392652742, -1.270000000000005791 ) ) ;
#27422=AXIS2_PLACEMENT_3D ( 'NONE', #18035, #28480, #21850 ) ;
#27429=CARTESIAN_POINT ( 'NONE',  ( -6.194847070882102180, 64.72978607931611350, 1.524000000000005350 ) ) ;
#27430=CARTESIAN_POINT ( 'NONE',  ( -57.31459482202865985, 1.982415423992395453, 1.558968780848406954 ) ) ;
#27431=CARTESIAN_POINT ( 'NONE',  ( -58.40597088826705630, 0.2738206778524349128, 0.9753506901443759203 ) ) ;
#27432=CARTESIAN_POINT ( 'NONE',  ( -58.64969807691807091, -0.3154622663803800520, 0.3299468374515310276 ) ) ;
#27435=ORIENTED_EDGE ( 'NONE', *, *, #22462, .T. ) ;
#27437=CARTESIAN_POINT ( 'NONE',  ( -50.36516092884956208, 15.79195539882771726, 4.916963016749596349 ) ) ;
#27440=AXIS2_PLACEMENT_3D ( 'NONE', #12556, #38548, #35349 ) ;
#27445=ORIENTED_EDGE ( 'NONE', *, *, #26308, .T. ) ;
#27449=CARTESIAN_POINT ( 'NONE',  ( -41.05192305526439611, 23.09448250258611068, -1.270000000023978615 ) ) ;
#27450=CARTESIAN_POINT ( 'NONE',  ( -44.28332145682819743, 21.53821517059777335, 3.041508016571806028 ) ) ;
#27453=ADVANCED_FACE ( 'NONE', ( #28614 ), #12432, .T. ) ;
#27454=DIRECTION ( 'NONE',  ( -5.188838149069472160E-16, 1.699382548006136559E-16, 1.000000000000000000 ) ) ;
#27467=CARTESIAN_POINT ( 'NONE',  ( -51.67551711146813176, 11.54346324480936481, 1.411685438026446526 ) ) ;
#27472=ORIENTED_EDGE ( 'NONE', *, *, #8400, .T. ) ;
#27477=VERTEX_POINT ( 'NONE', #36066 ) ;
#27480=PLANE ( 'NONE',  #14333 ) ;
#27481=DIRECTION ( 'NONE',  ( -5.188838149069472160E-16, 1.699382548006136559E-16, 1.000000000000000000 ) ) ;
#27482=VECTOR ( 'NONE', #1934, 1000.000000000000000 ) ;
#27484=CYLINDRICAL_SURFACE ( 'NONE', #32239, 0.6349999999999984546 ) ;
#27485=AXIS2_PLACEMENT_3D ( 'NONE', #30962, #34177, #12429 ) ;
#27487=DIRECTION ( 'NONE',  ( 5.188838149069472160E-16, -1.699382548006136559E-16, -1.000000000000000000 ) ) ;
#27488=DIRECTION ( 'NONE',  ( 0.4849315768086534528, 0.8745520943968250194, 1.030032898892974942E-16 ) ) ;
#27493=B_SPLINE_CURVE_WITH_KNOTS ( 'NONE', 3,
 ( #16979, #36596, #10172, #17192, #23359, #27001, #26791, #36808, #39583, #40012, #29979, #13374, #7625, #20584, #4443, #17401, #405, #36178, #30396, #6997, #1245, #14202, #27208, #11017 ),
 .UNSPECIFIED., .F., .F.,
 ( 4, 2, 2, 2, 2, 2, 2, 2, 2, 2, 2, 4 ),
 ( 0.000000000000000000, 0.001112600682894235998, 0.001668901024341350962, 0.002225201365788466359, 0.003337802048682695852, 0.004450402731576926646, 0.005563003414471156573, 0.006675604097365384765, 0.007231904438812500162, 0.007788204780259614692, 0.008344505121706728354, 0.008900805463153842884 ),
 .UNSPECIFIED. ) ;
#27501=FACE_OUTER_BOUND ( 'NONE', #18460, .T. ) ;
#27512=EDGE_CURVE ( 'NONE', #22599, #4427, #26465, .T. ) ;
#27514=ORIENTED_EDGE ( 'NONE', *, *, #33425, .T. ) ;
#27518=SURFACE_STYLE_FILL_AREA ( #20688 ) ;
#27520=CARTESIAN_POINT ( 'NONE',  ( -41.53952017147561548, 22.95708954751533781, 1.524002587545546294 ) ) ;
#27531=CARTESIAN_POINT ( 'NONE',  ( -58.45963793110873041, -0.4469582673315134480, 0.3141006534902464620 ) ) ;
#27539=( BOUNDED_SURFACE ( )  B_SPLINE_SURFACE ( 3, 2, ( 
 ( #8439, #25037, #21397 ),
 ( #20782, #34425, #14393 ),
 ( #37820, #8648, #18423 ),
 ( #40410, #2273, #15237 ) ),
 .UNSPECIFIED., .F., .F., .T. ) 
 B_SPLINE_SURFACE_WITH_KNOTS ( ( 4, 4 ),
 ( 3, 3 ),
 ( 5.204170427930421283E-18, 6.346505048318222639E-05 ),
 ( 0.000000000000000000, 1.000000000000000000 ),
 .UNSPECIFIED. ) 
 GEOMETRIC_REPRESENTATION_ITEM ( )  RATIONAL_B_SPLINE_SURFACE ( (
 ( 1.000000000000000000, 0.7071067811865614505, 1.000000000000000000),
 ( 1.000000000000000000, 0.7071067753522113364, 1.000000000000000000),
 ( 1.000000000000000000, 0.7071464246557911393, 1.000000000000000000),
 ( 1.000000000000000000, 0.7072256012392403868, 1.000000000000000000) ) ) 
 REPRESENTATION_ITEM ( '' )  SURFACE ( )  );
#27540=CARTESIAN_POINT ( 'NONE',  ( -57.91458998086623922, 0.5482684225795314559, -0.1438514718893213751 ) ) ;
#27542=CARTESIAN_POINT ( 'NONE',  ( -10.18297664959815663, 77.66688486464208552, -1.269999999999998019 ) ) ;
#27543=CYLINDRICAL_SURFACE ( 'NONE', #40425, 0.2539999999999937863 ) ;
#27545=DIRECTION ( 'NONE',  ( -0.8745520943968229099, 0.4849315768086570055, -5.361993529360569999E-16 ) ) ;
#27548=CARTESIAN_POINT ( 'NONE',  ( -7.772068811996249771, 69.25462295839062676, 1.270000000000003570 ) ) ;
#27552=ORIENTED_EDGE ( 'NONE', *, *, #11339, .T. ) ;
#27553=DIRECTION ( 'NONE',  ( 5.188838149069472160E-16, -1.699382548006136559E-16, -1.000000000000000000 ) ) ;
#27554=ORIENTED_EDGE ( 'NONE', *, *, #27271, .F. ) ;
#27555=CARTESIAN_POINT ( 'NONE',  ( -47.59852559864132360, 19.66225068540624932, -5.176489187672372871 ) ) ;
#27562=CARTESIAN_POINT ( 'NONE',  ( -49.41583470348051321, 17.21070444274963762, -5.043540371747944562 ) ) ;
#27565=CARTESIAN_POINT ( 'NONE',  ( -48.75754203680085652, 18.15534081570707414, -5.116688472081215799 ) ) ;
#27568=CARTESIAN_POINT ( 'NONE',  ( -45.91718695868514288, 25.22619731686664224, -1.578102078770073469 ) ) ;
#27575=CARTESIAN_POINT ( 'NONE',  ( -47.84356795211461844, 19.38525671449500010, -5.197506975155170572 ) ) ;
#27578=DIRECTION ( 'NONE',  ( -0.8745520943968235761, 0.4849315768086558398, 0.000000000000000000 ) ) ;
#27582=CARTESIAN_POINT ( 'NONE',  ( -58.33777482027510786, 1.113448835244251756, -1.208045587469442017 ) ) ;
#27583=CARTESIAN_POINT ( 'NONE',  ( -42.12253153191133492, 21.94389511927448311, -6.431429377749453771E-15 ) ) ;
#27586=CARTESIAN_POINT ( 'NONE',  ( -57.34787435976332404, 1.552391619547691004, -9.959991576465148270E-15 ) ) ;
#27589=CARTESIAN_POINT ( 'NONE',  ( -47.30609498763488574, 23.90227454495589399, -2.251708124038050762 ) ) ;
#27604=CARTESIAN_POINT ( 'NONE',  ( -46.04356002888985699, 20.98312591567169605, -4.505114092170838802 ) ) ;
#27605=ORIENTED_EDGE ( 'NONE', *, *, #6035, .T. ) ;
#27611=CARTESIAN_POINT ( 'NONE',  ( -58.22800107109949153, 0.01111325675459684525, -0.5047451677696692673 ) ) ;
#27616=VERTEX_POINT ( 'NONE', #3912 ) ;
#27619=FACE_OUTER_BOUND ( 'NONE', #11797, .T. ) ;
#27621=AXIS2_PLACEMENT_3D ( 'NONE', #11315, #40100, #24302 ) ;
#27633=CARTESIAN_POINT ( 'NONE',  ( -53.65068779629728368, 9.511520785580891868, 3.604358613835281222 ) ) ;
#27634=CARTESIAN_POINT ( 'NONE',  ( -50.92299000722575641, 14.78308106450686310, 4.710654750704142302 ) ) ;
#27635=CARTESIAN_POINT ( 'NONE',  ( -7.961576494521615643, 72.55615504727386167, 1.270000000000003126 ) ) ;
#27639=CARTESIAN_POINT ( 'NONE',  ( -48.21404017327530767, 19.06235592689615288, 5.351320745402585288 ) ) ;
#27645=DIRECTION ( 'NONE',  ( -0.5149185422762211362, 0.8572391118119444542, 0.000000000000000000 ) ) ;
#27648=VERTEX_POINT ( 'NONE', #17296 ) ;
#27651=DIRECTION ( 'NONE',  ( -5.188838149069471174E-16, 1.699382548006136313E-16, 1.000000000000000000 ) ) ;
#27652=CARTESIAN_POINT ( 'NONE',  ( -46.78477525497864775, 20.40172935490961237, 4.969468548369063932 ) ) ;
#27658=CARTESIAN_POINT ( 'NONE',  ( -6.650126595083637682, 78.47834120613788400, -1.523999999999996691 ) ) ;
#27666=EDGE_CURVE ( 'NONE', #39243, #41261, #18433, .T. ) ;
#27667=CARTESIAN_POINT ( 'NONE',  ( -52.76126113563441322, 10.11686208896574257, 1.835409310531171956 ) ) ;
#27671=VERTEX_POINT ( 'NONE', #40104 ) ;
#27672=CIRCLE ( 'NONE', #20176, 0.2539999999999997260 ) ;
#27677=ORIENTED_EDGE ( 'NONE', *, *, #16295, .F. ) ;
#27686=EDGE_CURVE ( 'NONE', #12622, #20165, #17138, .T. ) ;
#27687=LINE ( 'NONE', #37278, #29531 ) ;
#27693=ORIENTED_EDGE ( 'NONE', *, *, #35169, .F. ) ;
#27694=LINE ( 'NONE', #12136, #37694 ) ;
#27700=AXIS2_PLACEMENT_3D ( 'NONE', #29287, #32279, #25253 ) ;
#27715=ORIENTED_EDGE ( 'NONE', *, *, #41253, .T. ) ;
#27719=CYLINDRICAL_SURFACE ( 'NONE', #41601, 0.2540000000000012248 ) ;
#27727=VERTEX_POINT ( 'NONE', #31127 ) ;
#27730=CIRCLE ( 'NONE', #29097, 0.6350000000000014522 ) ;
#27731=CARTESIAN_POINT ( 'NONE',  ( -48.16232371144223379, 19.02200717994684354, 5.227009030889012031 ) ) ;
#27739=ADVANCED_FACE ( 'NONE', ( #21516 ), #27719, .T. ) ;
#27741=CARTESIAN_POINT ( 'NONE',  ( -57.47393550255003447, 1.325481720219581661, -1.020368242535414227E-14 ) ) ;
#27744=FACE_OUTER_BOUND ( 'NONE', #24482, .T. ) ;
#27746=DIRECTION ( 'NONE',  ( -5.188838149069472160E-16, 1.699382548006136559E-16, 1.000000000000000000 ) ) ;
#27750=CARTESIAN_POINT ( 'NONE',  ( -46.60530155212505576, 26.17382724835474406, -1.270000000000008233 ) ) ;
#27753=VERTEX_POINT ( 'NONE', #4954 ) ;
#27754=CARTESIAN_POINT ( 'NONE',  ( -41.09670346151854403, 23.04688172093030829, -1.270085369932534958 ) ) ;
#27756=CARTESIAN_POINT ( 'NONE',  ( -43.33782384754901074, 21.60941887712242959, -2.445739413454641742 ) ) ;
#27764=CARTESIAN_POINT ( 'NONE',  ( -49.77363268278942598, 16.65469053158889068, -4.972382134799542719 ) ) ;
#27772=CARTESIAN_POINT ( 'NONE',  ( -51.54051843738712080, 14.84038450301108192, -4.692172599169433411 ) ) ;
#27774=ORIENTED_EDGE ( 'NONE', *, *, #14708, .T. ) ;
#27778=CARTESIAN_POINT ( 'NONE',  ( -57.66338803320029882, 2.692357263605615891, -1.869785753600856637 ) ) ;
#27787=LINE ( 'NONE', #28424, #7242 ) ;
#27788=TOROIDAL_SURFACE ( 'NONE', #34612, 8.794749999999998735, 0.2540000000000000036 ) ;
#27789=CARTESIAN_POINT ( 'NONE',  ( -43.13073682054402269, 20.84535665847938546, -6.630667737810475277E-15 ) ) ;
#27790=ORIENTED_EDGE ( 'NONE', *, *, #5496, .F. ) ;
#27792=AXIS2_PLACEMENT_3D ( 'NONE', #40817, #27809, #8219 ) ;
#27794=CARTESIAN_POINT ( 'NONE',  ( -58.11144429832075531, 0.1746852717545294142, -1.039312118988176566E-14 ) ) ;
#27795=CARTESIAN_POINT ( 'NONE',  ( -51.68405183998543606, 20.46365084016696301, -1.001587320847779132E-14 ) ) ;
#27797=EDGE_LOOP ( 'NONE', ( #37563, #14454, #6758, #40314 ) ) ;
#27798=CARTESIAN_POINT ( 'NONE',  ( -49.15418727280429323, 24.05022843951647715, -1.025120094619365347E-14 ) ) ;
#27801=ORIENTED_EDGE ( 'NONE', *, *, #852, .T. ) ;
#27809=DIRECTION ( 'NONE',  ( 5.188838149069472160E-16, -1.699382548006136559E-16, -1.000000000000000000 ) ) ;
#27812=CARTESIAN_POINT ( 'NONE',  ( -8.519412162535125788, 69.40335734044577976, -1.269999999999996021 ) ) ;
#27814=CARTESIAN_POINT ( 'NONE',  ( -23.75997692595333177, 82.67351089148900201, -1.524000000000006239 ) ) ;
#27819=CARTESIAN_POINT ( 'NONE',  ( -58.31060438690772685, -0.1666892599193892099, -0.3090539641404843052 ) ) ;
#27824=B_SPLINE_CURVE_WITH_KNOTS ( 'NONE', 3,
 ( #5514, #20831, #4894, #37451, #2322, #15282, #40257 ),
 .UNSPECIFIED., .F., .F.,
 ( 4, 3, 4 ),
 ( -5.999999998588015393E-08, 2.316105715148477490E-21, 6.533385609066403601E-05 ),
 .UNSPECIFIED. ) ;
#27825=ORIENTED_EDGE ( 'NONE', *, *, #41808, .T. ) ;
#27828=VECTOR ( 'NONE', #33737, 1000.000000000000000 ) ;
#27831=DIRECTION ( 'NONE',  ( 0.9454731675810359448, -0.3256999990547780333, 5.459396135145339171E-16 ) ) ;
#27833=ORIENTED_EDGE ( 'NONE', *, *, #36079, .F. ) ;
#27840=CARTESIAN_POINT ( 'NONE',  ( -8.576171974424218192, 74.02775907367175989, -1.269999999999996909 ) ) ;
#27843=PLANE ( 'NONE',  #19237 ) ;
#27844=CARTESIAN_POINT ( 'NONE',  ( -58.36876032087972987, -0.2894071526118170423, 0.03821653909995503112 ) ) ;
#27845=CARTESIAN_POINT ( 'NONE',  ( -29.12312633940434381, 66.61190372955218209, -1.524000000000006017 ) ) ;
#27846=CARTESIAN_POINT ( 'NONE',  ( -25.77058783747419213, 72.83664265955201245, 1.269999999999993801 ) ) ;
#27849=ORIENTED_EDGE ( 'NONE', *, *, #26331, .F. ) ;
#27850=CARTESIAN_POINT ( 'NONE',  ( -52.97391985390434144, 12.30611266682019789, 4.247241762254901687 ) ) ;
#27851=AXIS2_PLACEMENT_3D ( 'NONE', #37615, #8440, #37821 ) ;
#27856=DIRECTION ( 'NONE',  ( -0.6559537821943227653, 0.7548010569845297058, -3.677505126197116308E-15 ) ) ;
#27861=CARTESIAN_POINT ( 'NONE',  ( -29.82321757229076908, 71.17901112636586447, 1.269999999999992690 ) ) ;
#27862=CARTESIAN_POINT ( 'NONE',  ( -41.28107547821696954, 23.22158991241120063, 1.523999999999993138 ) ) ;
#27863=CARTESIAN_POINT ( 'NONE',  ( -47.85244527695896011, 19.39403540832957518, 5.219971639306693056 ) ) ;
#27867=DIRECTION ( 'NONE',  ( 5.188838149069472160E-16, -1.699382548006136559E-16, -1.000000000000000000 ) ) ;
#27874=VERTEX_POINT ( 'NONE', #21309 ) ;
#27875=CARTESIAN_POINT ( 'NONE',  ( -53.01551111795199489, 8.729259440421063942, -8.823202585156807211E-15 ) ) ;
#27889=EDGE_CURVE ( 'NONE', #28485, #4128, #28667, .T. ) ;
#27890=CARTESIAN_POINT ( 'NONE',  ( -8.816700480405424756, 73.94613776634058411, 1.270000000000002460 ) ) ;
#27894=CARTESIAN_POINT ( 'NONE',  ( -41.18107378286554621, 22.95619949144852967, 1.523999999999987143 ) ) ;
#27902=CIRCLE ( 'NONE', #36771, 0.3810000000000000053 ) ;
#27907=CARTESIAN_POINT ( 'NONE',  ( -51.09183723991096571, 15.73968240350219538, 4.743875354842988834 ) ) ;
#27923=ORIENTED_EDGE ( 'NONE', *, *, #4066, .T. ) ;
#27924=ORIENTED_EDGE ( 'NONE', *, *, #22738, .F. ) ;
#27925=DIRECTION ( 'NONE',  ( -5.188838149069472160E-16, 1.699382548006136066E-16, 1.000000000000000000 ) ) ;
#27941=CARTESIAN_POINT ( 'NONE',  ( -58.49146960918517379, -0.5079027975612510071, 0.2843517202610890138 ) ) ;
#27949=CARTESIAN_POINT ( 'NONE',  ( -57.26476250566310711, 1.946856395439316989, -1.045107959733444281 ) ) ;
#27957=CARTESIAN_POINT ( 'NONE',  ( -24.26619908708080686, 81.70586579672512073, -1.524000000000006239 ) ) ;
#27962=ORIENTED_EDGE ( 'NONE', *, *, #6096, .F. ) ;
#27963=CARTESIAN_POINT ( 'NONE',  ( -58.33482727260577860, 1.278009831242016281, -0.06942977984277290404 ) ) ;
#27964=EDGE_CURVE ( 'NONE', #22515, #8970, #6234, .T. ) ;
#27966=CARTESIAN_POINT ( 'NONE',  ( -47.33874550351251997, 19.91900851598762046, -5.121984950663424740 ) ) ;
#27973=CARTESIAN_POINT ( 'NONE',  ( -49.51384108118372751, 17.06003269541576017, -5.024714039402652155 ) ) ;
#27976=DIRECTION ( 'NONE',  ( -0.8745520943968240202, 0.4849315768086551737, -5.361993529360572958E-16 ) ) ;
#27978=CARTESIAN_POINT ( 'NONE',  ( -48.81575351190421941, 18.06815554827317882, -5.105115732439140963 ) ) ;
#27979=EDGE_CURVE ( 'NONE', #14494, #40718, #9188, .T. ) ;
#27982=CARTESIAN_POINT ( 'NONE',  ( -51.34009458250667279, 14.66650723912346699, -4.800162786360146150 ) ) ;
#27983=EDGE_CURVE ( 'NONE', #4082, #15081, #23881, .T. ) ;
#27989=TOROIDAL_SURFACE ( 'NONE', #9624, 0.3810000000000005604, 0.2540000000000000036 ) ;
#27990=CARTESIAN_POINT ( 'NONE',  ( -57.00508801794419611, 2.691366720778187727, -1.977812201481553567 ) ) ;
#27993=DIRECTION ( 'NONE',  ( -5.188838149069472160E-16, 1.699382548006136559E-16, 1.000000000000000000 ) ) ;
#27997=CARTESIAN_POINT ( 'NONE',  ( -41.05189575270519242, 23.09451173561983239, -5.978253955787443857E-15 ) ) ;
#28001=CARTESIAN_POINT ( 'NONE',  ( -57.56998337575458891, 1.440017903778734176, 1.358936928125925814 ) ) ;
#28002=CARTESIAN_POINT ( 'NONE',  ( -51.34394198884087501, 20.23131347170496142, 0.7795225783603342284 ) ) ;
#28005=CARTESIAN_POINT ( 'NONE',  ( -47.59569394876871229, 21.45978420380969354, -4.300550031832348630 ) ) ;
#28008=ORIENTED_EDGE ( 'NONE', *, *, #32332, .F. ) ;
#28022=ORIENTED_EDGE ( 'NONE', *, *, #39384, .T. ) ;
#28026=CARTESIAN_POINT ( 'NONE',  ( -58.43492521371434378, -0.3997831091937082415, -0.3282367010173031230 ) ) ;
#28033=ORIENTED_EDGE ( 'NONE', *, *, #34877, .T. ) ;
#28036=AXIS2_PLACEMENT_3D ( 'NONE', #8156, #15586, #21126 ) ;
#28042=CARTESIAN_POINT ( 'NONE',  ( -3.831877602099685198, 71.07198261757335445, -1.269999999999993801 ) ) ;
#28043=CARTESIAN_POINT ( 'NONE',  ( -26.51793118801306548, 72.98537704160715123, -1.270000000000006013 ) ) ;
#28044=AXIS2_PLACEMENT_3D ( 'NONE', #15381, #24975, #41393 ) ;
#28048=CARTESIAN_POINT ( 'NONE',  ( -46.60530155212503445, 26.17382724835477958, -1.524000000000008459 ) ) ;
#28051=CARTESIAN_POINT ( 'NONE',  ( -57.98432510407339180, 0.5385510273032687589, 0.8796703754388934815 ) ) ;
#28052=CARTESIAN_POINT ( 'NONE',  ( -29.91360363449003756, 70.04874496952835727, -1.524000000000007349 ) ) ;
#28053=CARTESIAN_POINT ( 'NONE',  ( -18.01920641645600796, 83.84822824455467583, -1.524000000000003352 ) ) ;
#28056=VERTEX_POINT ( 'NONE', #12383 ) ;
#28057=CARTESIAN_POINT ( 'NONE',  ( -53.75224695799815322, 9.373383622779334345, 3.688627211158417296 ) ) ;
#28063=DIRECTION ( 'NONE',  ( -0.1906721105965186736, 0.9816537812491066273, 0.000000000000000000 ) ) ;
#28065=ORIENTED_EDGE ( 'NONE', *, *, #35598, .F. ) ;
#28067=CARTESIAN_POINT ( 'NONE',  ( -29.22020851855505441, 63.09400180734589014, 1.524000000000856669 ) ) ;
#28068=CARTESIAN_POINT ( 'NONE',  ( -6.194847070882102180, 64.72978607931611350, -1.523999999999994026 ) ) ;
#28069=CARTESIAN_POINT ( 'NONE',  ( -22.95370498042275642, 82.54569470718179502, -1.270000000000005791 ) ) ;
#28070=CARTESIAN_POINT ( 'NONE',  ( -48.16751460313091115, 19.56873862626650507, 5.361827705663260168 ) ) ;
#28080=AXIS2_PLACEMENT_3D ( 'NONE', #25196, #28395, #38200 ) ;
#28083=CARTESIAN_POINT ( 'NONE',  ( -56.91016477577836952, 2.896953902749091370, 2.060321699028983211 ) ) ;
#28099=CARTESIAN_POINT ( 'NONE',  ( -15.77830307927088249, 80.39606975582424297, -1.270000000000001572 ) ) ;
#28100=AXIS2_PLACEMENT_3D ( 'NONE', #14852, #27856, #15490 ) ;
#28103=CARTESIAN_POINT ( 'NONE',  ( -14.42383115828894447, 69.61113539875873357, -1.523999999999998911 ) ) ;
#28107=ORIENTED_EDGE ( 'NONE', *, *, #7690, .F. ) ;
#28108=DIRECTION ( 'NONE',  ( -5.188838149069471174E-16, 1.699382548006136313E-16, 1.000000000000000000 ) ) ;
#28114=AXIS2_PLACEMENT_3D ( 'NONE', #39171, #9978, #32784 ) ;
#28142=AXIS2_PLACEMENT_3D ( 'NONE', #21602, #34630, #40607 ) ;
#28148=CIRCLE ( 'NONE', #5730, 0.6350000000000006750 ) ;
#28149=VERTEX_POINT ( 'NONE', #29565 ) ;
#28151=CARTESIAN_POINT ( 'NONE',  ( -16.02764313970816090, 80.34763903973272647, 1.269999999999997353 ) ) ;
#28154=CARTESIAN_POINT ( 'NONE',  ( -54.28468382810394388, 8.706709151474493424, 3.613316249070154473 ) ) ;
#28165=CARTESIAN_POINT ( 'NONE',  ( -57.25386126824266597, 1.903786294961781866, -0.7664973485411553655 ) ) ;
#28170=DIRECTION ( 'NONE',  ( 0.8745520943968235761, -0.4849315768086558398, 0.000000000000000000 ) ) ;
#28173=FACE_BOUND ( 'NONE', #10807, .T. ) ;
#28177=VERTEX_POINT ( 'NONE', #8976 ) ;
#28178=CARTESIAN_POINT ( 'NONE',  ( -58.62011547798931588, 0.4741971735572336755, -0.2911429440373615174 ) ) ;
#28179=ORIENTED_EDGE ( 'NONE', *, *, #24554, .T. ) ;
#28180=CARTESIAN_POINT ( 'NONE',  ( -20.59944062528794362, 79.83666051618703818, 1.269999999999995133 ) ) ;
#28188=CARTESIAN_POINT ( 'NONE',  ( -58.49576617200561657, -0.01047455392627871275, -0.6956555549625097479 ) ) ;
#28189=ORIENTED_EDGE ( 'NONE', *, *, #26963, .F. ) ;
#28191=DIRECTION ( 'NONE',  ( -5.188838149069472160E-16, 1.699382548006136559E-16, 1.000000000000000000 ) ) ;
#28193=CARTESIAN_POINT ( 'NONE',  ( -48.71914655128158245, 18.21236406733019209, -5.124034746316241673 ) ) ;
#28196=CARTESIAN_POINT ( 'NONE',  ( -50.58884987432006852, 15.93229845861179861, -5.010371253631922706 ) ) ;
#28197=EDGE_CURVE ( 'NONE', #25412, #20165, #34972, .T. ) ;
#28203=CARTESIAN_POINT ( 'NONE',  ( -57.52317756609133426, 3.014644041894651405, -1.981665235817958948 ) ) ;
#28206=EDGE_CURVE ( 'NONE', #30025, #32851, #25263, .T. ) ;
#28207=DIRECTION ( 'NONE',  ( -0.8745520943968225769, 0.4849315768086578382, -5.691349986800571545E-16 ) ) ;
#28210=DIRECTION ( 'NONE',  ( 0.7770581983690836303, -0.6294287539884032556, 5.101669463485833779E-16 ) ) ;
#28211=EDGE_CURVE ( 'NONE', #19344, #30808, #8052, .T. ) ;
#28212=CARTESIAN_POINT ( 'NONE',  ( -41.35393432493753352, 22.77111593294431913, -0.9171044195162123547 ) ) ;
#28213=ORIENTED_EDGE ( 'NONE', *, *, #34715, .T. ) ;
#28215=CARTESIAN_POINT ( 'NONE',  ( -58.73801720703743001, -0.4998429216807459552, 0.2437502737749395465 ) ) ;
#28219=CARTESIAN_POINT ( 'NONE',  ( -53.04800011033383811, 17.61732480341419915, 0.3294858417196632749 ) ) ;
#28222=CARTESIAN_POINT ( 'NONE',  ( -49.72500615219620101, 20.62299186128851858, -2.281585690523513232 ) ) ;
#28225=ORIENTED_EDGE ( 'NONE', *, *, #34923, .F. ) ;
#28237=FACE_OUTER_BOUND ( 'NONE', #9649, .T. ) ;
#28239=ORIENTED_EDGE ( 'NONE', *, *, #27964, .F. ) ;
#28240=CIRCLE ( 'NONE', #33030, 0.3810000000000015041 ) ;
#28254=CARTESIAN_POINT ( 'NONE',  ( -41.05189575270516400, 23.09451173561986081, -1.524000000000003130 ) ) ;
#28255=EDGE_CURVE ( 'NONE', #1003, #24894, #4878, .T. ) ;
#28263=CARTESIAN_POINT ( 'NONE',  ( -23.43300365160792964, 82.12916405548841681, -1.524000000000006017 ) ) ;
#28267=CARTESIAN_POINT ( 'NONE',  ( -58.05509315856782848, 0.3850302431961226679, 0.7835795507822739259 ) ) ;
#28269=EDGE_CURVE ( 'NONE', #30709, #27616, #17140, .T. ) ;
#28270=DIRECTION ( 'NONE',  ( -0.1906721105965039909, 0.9816537812491094028, -2.657572025465702696E-16 ) ) ;
#28273=ADVANCED_FACE ( 'NONE', ( #8890 ), #2089, .T. ) ;
#28274=EDGE_LOOP ( 'NONE', ( #16129, #25544, #23136, #34721 ) ) ;
#28275=CARTESIAN_POINT ( 'NONE',  ( -49.01671973967521012, 18.67808020721676954, 5.174630477995038724 ) ) ;
#28280=CARTESIAN_POINT ( 'NONE',  ( -5.684927786827003615, 65.51297084251929448, -1.523999999999993804 ) ) ;
#28283=CARTESIAN_POINT ( 'NONE',  ( -29.91360363449003401, 70.04874496952835727, 1.523999999999991806 ) ) ;
#28285=CARTESIAN_POINT ( 'NONE',  ( -41.77909418349046433, 22.73884196981243377, 1.565812447105980887 ) ) ;
#28298=ORIENTED_EDGE ( 'NONE', *, *, #34244, .F. ) ;
#28299=CARTESIAN_POINT ( 'NONE',  ( -57.23135758994266098, 1.814875683430833275, 0.2588789259697444889 ) ) ;
#28300=AXIS2_PLACEMENT_3D ( 'NONE', #41986, #24941, #6202 ) ;
#28304=ORIENTED_EDGE ( 'NONE', *, *, #26623, .T. ) ;
#28309=ORIENTED_EDGE ( 'NONE', *, *, #24064, .T. ) ;
#28319=CARTESIAN_POINT ( 'NONE',  ( -46.30033180095409762, 21.65562830348028456, 4.292083522273594909 ) ) ;
#28350=ORIENTED_EDGE ( 'NONE', *, *, #28255, .T. ) ;
#28355=DIRECTION ( 'NONE',  ( 0.01731298258488073519, -0.9998501190848635423, 1.788962107505278613E-16 ) ) ;
#28358=VECTOR ( 'NONE', #9966, 999.9999999999998863 ) ;
#28364=AXIS2_PLACEMENT_3D ( 'NONE', #8368, #37339, #27545 ) ;
#28367=CYLINDRICAL_SURFACE ( 'NONE', #24470, 0.2539999999999973390 ) ;
#28369=CARTESIAN_POINT ( 'NONE',  ( -58.63679809531443965, -0.7731007215655836262, -1.422417852365874970E-12 ) ) ;
#28375=AXIS2_PLACEMENT_3D ( 'NONE', #12887, #9693, #25671 ) ;
#28379=CARTESIAN_POINT ( 'NONE',  ( -57.41561397472474937, 1.705883423724310788, -1.231064337386920782 ) ) ;
#28384=CARTESIAN_POINT ( 'NONE',  ( -17.08598887363762131, 83.79821757228496892, 1.269999999999996243 ) ) ;
#28387=FACE_OUTER_BOUND ( 'NONE', #14877, .T. ) ;
#28388=CARTESIAN_POINT ( 'NONE',  ( -58.83227707057485389, -0.08366279997994163775, -1.533110566128065488E-14 ) ) ;
#28391=VECTOR ( 'NONE', #36265, 1000.000000000000114 ) ;
#28395=DIRECTION ( 'NONE',  ( -0.4849315768086535083, -0.8745520943968250194, -1.030032898892974695E-16 ) ) ;
#28402=CARTESIAN_POINT ( 'NONE',  ( -57.58628444390482315, 1.951741080605158718, -1.744151961578425780 ) ) ;
#28403=ORIENTED_EDGE ( 'NONE', *, *, #15276, .F. ) ;
#28407=CARTESIAN_POINT ( 'NONE',  ( -50.96693996911965741, 14.52141170389602998, -4.551080797630170593 ) ) ;
#28410=CARTESIAN_POINT ( 'NONE',  ( -56.82628769568140115, 4.502340570254503405, -2.499646007873257414 ) ) ;
#28417=CARTESIAN_POINT ( 'NONE',  ( -58.70413935429054675, 0.2332485698458008905, -0.6626129746612972049 ) ) ;
#28421=EDGE_CURVE ( 'NONE', #24097, #28898, #17833, .T. ) ;
#28424=CARTESIAN_POINT ( 'NONE',  ( -17.58995245299101029, 75.15621874538170744, 1.523999999999997801 ) ) ;
#28425=CARTESIAN_POINT ( 'NONE',  ( -41.05189575270517111, 23.09451173561986792, -0.08466666666667251040 ) ) ;
#28426=DIRECTION ( 'NONE',  ( -5.188838149069472160E-16, 1.699382548006136559E-16, 1.000000000000000000 ) ) ;
#28427=CARTESIAN_POINT ( 'NONE',  ( -57.67794393518098417, 1.927849678527493449, 1.763631237166035648 ) ) ;
#28428=CARTESIAN_POINT ( 'NONE',  ( -51.14897750729640080, 14.40149654946681501, 4.652905086514556920 ) ) ;
#28429=CARTESIAN_POINT ( 'NONE',  ( -10.18297664959815663, 77.66688486464208552, -1.523999999999998245 ) ) ;
#28430=STYLED_ITEM ( 'NONE', ( #7303 ), #41738 ) ;
#28432=CARTESIAN_POINT ( 'NONE',  ( -52.14602366315243387, 18.74265329119796064, 0.7451446608535526872 ) ) ;
#28436=CARTESIAN_POINT ( 'NONE',  ( -49.25189787529244967, 18.82624764011888630, -4.709232814563292457 ) ) ;
#28448=DIRECTION ( 'NONE',  ( -5.188838149069472160E-16, 1.699382548006136559E-16, 1.000000000000000000 ) ) ;
#28455=DIRECTION ( 'NONE',  ( -5.188838149069472160E-16, 1.699382548006136559E-16, 1.000000000000000000 ) ) ;
#28469=CARTESIAN_POINT ( 'NONE',  ( -43.93316818929329770, 24.49458088220322338, -1.524000000000007349 ) ) ;
#28470=ORIENTED_EDGE ( 'NONE', *, *, #2814, .T. ) ;
#28472=CARTESIAN_POINT ( 'NONE',  ( -28.60507221318228943, 76.72702915747851193, -1.524000000000007793 ) ) ;
#28473=CIRCLE ( 'NONE', #10099, 0.2539999999999998925 ) ;
#28474=CIRCLE ( 'NONE', #6055, 0.2540000000000000036 ) ;
#28480=DIRECTION ( 'NONE',  ( 0.3582377630123958490, -0.9336303900108837706, 3.445432962228686790E-16 ) ) ;
#28481=CARTESIAN_POINT ( 'NONE',  ( -58.29410838023627406, -0.1313788046413840727, 0.3526482289038367912 ) ) ;
#28485=VERTEX_POINT ( 'NONE', #25070 ) ;
#28490=ORIENTED_EDGE ( 'NONE', *, *, #32859, .F. ) ;
#28492=FACE_OUTER_BOUND ( 'NONE', #26716, .T. ) ;
#28495=DIRECTION ( 'NONE',  ( 0.1951894777626611566, 0.9807655518882887336, 0.000000000000000000 ) ) ;
#28501=FACE_OUTER_BOUND ( 'NONE', #15293, .T. ) ;
#28505=AXIS2_PLACEMENT_3D ( 'NONE', #36949, #10944, #7558 ) ;
#28510=CARTESIAN_POINT ( 'NONE',  ( -55.65298819915649631, 5.540485941798498182, 2.823722248809246160 ) ) ;
#28512=EDGE_CURVE ( 'NONE', #41032, #21375, #34888, .T. ) ;
#28523=DIRECTION ( 'NONE',  ( -0.4849315768086535083, -0.8745520943968250194, -1.030032898892974695E-16 ) ) ;
#28531=CARTESIAN_POINT ( 'NONE',  ( -46.95766867967832070, 25.94401225812155332, -8.271762106911890930E-15 ) ) ;
#28533=CARTESIAN_POINT ( 'NONE',  ( -46.20552558087364758, 24.41938074005533466, 2.020549794458497139 ) ) ;
#28536=ORIENTED_EDGE ( 'NONE', *, *, #37840, .T. ) ;
#28537=CARTESIAN_POINT ( 'NONE',  ( -20.56295647043122798, 79.40745607177142062, 1.269999999999995133 ) ) ;
#28544=DIRECTION ( 'NONE',  ( 0.8745520943968243532, -0.4849315768086547296, 6.829619984160642269E-16 ) ) ;
#28559=VERTEX_POINT ( 'NONE', #29053 ) ;
#28561=ORIENTED_EDGE ( 'NONE', *, *, #28983, .T. ) ;
#28562=DIRECTION ( 'NONE',  ( 0.8745520943968221328, -0.4849315768086585043, -5.226292508699494473E-15 ) ) ;
#28565=DIRECTION ( 'NONE',  ( 0.9998501190848636533, 0.01731298258487584674, -2.441448296158442805E-15 ) ) ;
#28570=LINE ( 'NONE', #38379, #5919 ) ;
#28573=DIRECTION ( 'NONE',  ( -0.9734199927291317112, -0.2290273297124542085, -2.993963672467862566E-15 ) ) ;
#28577=ADVANCED_FACE ( 'NONE', ( #19458 ), #33458, .T. ) ;
#28579=CARTESIAN_POINT ( 'NONE',  ( -8.095114962461808616, 74.19100168833409725, -1.523999999999996691 ) ) ;
#28580=CARTESIAN_POINT ( 'NONE',  ( -58.27365357893031472, 0.4699239364188423362, 1.042275140647600296 ) ) ;
#28583=CARTESIAN_POINT ( 'NONE',  ( -19.33375693323417011, 80.42273151551299293, -1.524000000000003574 ) ) ;
#28587=LINE ( 'NONE', #22166, #6265 ) ;
#28592=LINE ( 'NONE', #41600, #21550 ) ;
#28595=DIRECTION ( 'NONE',  ( 0.000000000000000000, 0.000000000000000000, 1.000000000000000000 ) ) ;
#28600=CARTESIAN_POINT ( 'NONE',  ( -7.917360960270783288, 70.00264313970245666, -1.523999999999995802 ) ) ;
#28601=ORIENTED_EDGE ( 'NONE', *, *, #38000, .T. ) ;
#28606=CIRCLE ( 'NONE', #14392, 0.2540000000000008917 ) ;
#28609=CARTESIAN_POINT ( 'NONE',  ( -57.17105480285722763, 2.836315218834683627, -2.065842682462495805 ) ) ;
#28612=CARTESIAN_POINT ( 'NONE',  ( -37.29905550412968296, 27.11271634945815023, -1.270000000000003793 ) ) ;
#28614=FACE_OUTER_BOUND ( 'NONE', #21504, .T. ) ;
#28617=CARTESIAN_POINT ( 'NONE',  ( -52.76912830878634253, 12.08540908813377612, -4.334427935445254398 ) ) ;
#28626=CARTESIAN_POINT ( 'NONE',  ( -46.87302333143581734, 25.14943835889833323, 1.855287453902036310 ) ) ;
#28627=AXIS2_PLACEMENT_3D ( 'NONE', #37567, #21356, #34382 ) ;
#28630=CARTESIAN_POINT ( 'NONE',  ( -49.59816314059867182, 17.91649583374774224, -5.069000701391666475 ) ) ;
#28631=CARTESIAN_POINT ( 'NONE',  ( -48.30662019010082986, 17.20352665082216248, -3.142973069415128329 ) ) ;
#28632=ORIENTED_EDGE ( 'NONE', *, *, #22054, .T. ) ;
#28635=CARTESIAN_POINT ( 'NONE',  ( -58.03414100541874632, 0.4564111095344686175, 0.9708715263941495310 ) ) ;
#28636=CARTESIAN_POINT ( 'NONE',  ( -53.90086641569129711, 9.437825775582018295, 3.763139710719413777 ) ) ;
#28637=DIRECTION ( 'NONE',  ( 0.8745520943968250194, -0.4849315768086535083, 5.361993529360574930E-16 ) ) ;
#28638=B_SPLINE_CURVE_WITH_KNOTS ( 'NONE', 3,
 ( #8150, #25120, #8938, #2566, #21904, #34934, #4769, #5760, #18712, #1572, #12343, #25331, #35341, #38334, #38538, #9152, #5965, #6168, #30516, #1355, #25948, #10400, #6789, #15937, #29582, #39597, #16140, #200, #22945, #19979, #19545, #16570, #12752, #13176, #7010, #16788, #32995, #3175, #26163, #6578 ),
 .UNSPECIFIED., .F., .F.,
 ( 4, 2, 1, 2, 2, 2, 1, 1, 2, 2, 2, 2, 1, 1, 1, 2, 2, 2, 2, 1, 1, 2, 2, 4 ),
 ( 0.000000000000000000, 0.1250000000002643996, 0.1875000000003943790, 0.2187500000004593548, 0.2500000000005243583, 0.3750000000007865375, 0.4375000000009133250, 0.4687500000009737766, 0.4843750000010039192, 0.5000000000010339507, 0.6250000000012972956, 0.6875000000014240831, 0.7187500000014875878, 0.7343750000015164536, 0.7421875000015335511, 0.7460937500015469848, 0.7500000000015603074, 0.8125000000011977086, 0.8437500000010164092, 0.8593750000009239276, 0.8671875000008757439, 0.8710937500008516521, 0.8750000000008275602, 1.000000000000000000 ),
 .UNSPECIFIED. ) ;
#28640=CARTESIAN_POINT ( 'NONE',  ( -53.35592009511452716, 14.94916803242400682, 1.377413129700644889 ) ) ;
#28643=CARTESIAN_POINT ( 'NONE',  ( -48.75318004186330967, 22.89261100037833785, -1.301163434177661893 ) ) ;
#28646=VERTEX_POINT ( 'NONE', #36096 ) ;
#28658=CARTESIAN_POINT ( 'NONE',  ( -17.82828877264048018, 64.92754330167842625, 1.523999999999999355 ) ) ;
#28661=CARTESIAN_POINT ( 'NONE',  ( -58.36509063484196957, -0.2817187151746531337, -0.08504981361425689723 ) ) ;
#28667=CIRCLE ( 'NONE', #16399, 0.5080000000000000071 ) ;
#28668=ADVANCED_FACE ( 'NONE', ( #36308 ), #16898, .F. ) ;
#28676=ORIENTED_EDGE ( 'NONE', *, *, #8361, .T. ) ;
#28679=AXIS2_PLACEMENT_3D ( 'NONE', #17525, #23917, #1365 ) ;
#28680=CARTESIAN_POINT ( 'NONE',  ( -23.62918761621517660, 82.45577215708875940, 1.269999999999993134 ) ) ;
#28686=CIRCLE ( 'NONE', #34145, 0.2540000000000027236 ) ;
#28687=CARTESIAN_POINT ( 'NONE',  ( -58.34582891702650187, -0.2413224179734804187, 0.1928638016484154616 ) ) ;
#28692=ORIENTED_EDGE ( 'NONE', *, *, #34254, .F. ) ;
#28699=ORIENTED_EDGE ( 'NONE', *, *, #27983, .F. ) ;
#28701=CARTESIAN_POINT ( 'NONE',  ( -29.47815206431988599, 60.51098513936971557, 1.269999999999994023 ) ) ;
#28702=DIRECTION ( 'NONE',  ( 5.188838149069472160E-16, -1.699382548006136559E-16, -1.000000000000000000 ) ) ;
#28703=CARTESIAN_POINT ( 'NONE',  ( -42.52099730114425569, 21.88661877469040817, 1.711735796960834666 ) ) ;
#28708=CARTESIAN_POINT ( 'NONE',  ( -5.591535794131392123, 65.03215273817657760, 1.270000000000005569 ) ) ;
#28714=VERTEX_POINT ( 'NONE', #16686 ) ;
#28715=CARTESIAN_POINT ( 'NONE',  ( -57.43854689232674815, 1.757847328446637825, 1.624773336220233011 ) ) ;
#28718=DIRECTION ( 'NONE',  ( -0.8745520943968243532, 0.4849315768086547296, -6.829619984160642269E-16 ) ) ;
#28719=AXIS2_PLACEMENT_3D ( 'NONE', #37759, #21974, #22176 ) ;
#28723=ORIENTED_EDGE ( 'NONE', *, *, #14350, .F. ) ;
#28729=CIRCLE ( 'NONE', #9707, 9.048750000000000071 ) ;
#28731=EDGE_CURVE ( 'NONE', #37020, #5536, #22639, .T. ) ;
#28732=CYLINDRICAL_SURFACE ( 'NONE', #36325, 0.5080000000000000071 ) ;
#28734=CARTESIAN_POINT ( 'NONE',  ( -46.60530155212503445, 26.17382724835477958, -8.082077239948803202E-15 ) ) ;
#28736=CARTESIAN_POINT ( 'NONE',  ( -41.45218294293373162, 22.69057396248467384, 1.547390787314418592 ) ) ;
#28742=EDGE_CURVE ( 'NONE', #30888, #24697, #22557, .T. ) ;
#28764=AXIS2_PLACEMENT_3D ( 'NONE', #38494, #32736, #41694 ) ;
#28766=ORIENTED_EDGE ( 'NONE', *, *, #10562, .T. ) ;
#28769=CARTESIAN_POINT ( 'NONE',  ( -41.05189575270517821, 23.09451173561983950, 1.523999999999993582 ) ) ;
#28770=ADVANCED_FACE ( 'NONE', ( #13291 ), #32772, .T. ) ;
#28778=CARTESIAN_POINT ( 'NONE',  ( -23.69188486464780752, 78.08202335040543574, 1.269999999999993801 ) ) ;
#28783=CARTESIAN_POINT ( 'NONE',  ( -11.24191166894635430, 82.34025985790688651, 1.269999999999999352 ) ) ;
#28784=CIRCLE ( 'NONE', #20608, 0.2540000000000057767 ) ;
#28785=CYLINDRICAL_SURFACE ( 'NONE', #24520, 0.5080000000000007843 ) ;
#28788=CARTESIAN_POINT ( 'NONE',  ( -9.960492004070040650, 64.81807050032566053, -1.523999999999996025 ) ) ;
#28801=DIRECTION ( 'NONE',  ( -0.8745520943968240202, 0.4849315768086551737, -5.361993529360572958E-16 ) ) ;
#28804=EDGE_CURVE ( 'NONE', #19390, #18488, #7332, .T. ) ;
#28810=ORIENTED_EDGE ( 'NONE', *, *, #6119, .F. ) ;
#28813=CARTESIAN_POINT ( 'NONE',  ( -43.16005656664464851, 21.89413631511616032, -2.197846903552944653 ) ) ;
#28819=CARTESIAN_POINT ( 'NONE',  ( -58.13819340830944071, 0.7633750567142213450, -1.210128363568031995 ) ) ;
#28820=CIRCLE ( 'NONE', #4339, 0.2540000000000015024 ) ;
#28821=ORIENTED_EDGE ( 'NONE', *, *, #25333, .F. ) ;
#28822=CARTESIAN_POINT ( 'NONE',  ( -58.44960050528086271, -0.4277149010484683211, -0.3217025345699726646 ) ) ;
#28823=CARTESIAN_POINT ( 'NONE',  ( -3.841520934845505941, 71.62889921741444255, 1.270000000000005125 ) ) ;
#28826=LINE ( 'NONE', #35026, #2099 ) ;
#28829=CARTESIAN_POINT ( 'NONE',  ( -58.03414100541874632, 0.4564111095344686175, -0.9708715263941700702 ) ) ;
#28830=CIRCLE ( 'NONE', #13191, 0.3810000000000015041 ) ;
#28833=EDGE_LOOP ( 'NONE', ( #35364, #6479, #41754, #13271 ) ) ;
#28837=CARTESIAN_POINT ( 'NONE',  ( -58.37116772670351850, -0.2940390518722524327, -2.603646672650065119E-13 ) ) ;
#28840=CARTESIAN_POINT ( 'NONE',  ( -47.00737061383054538, 25.44871393995434872, 1.744193148939842564 ) ) ;
#28841=AXIS2_PLACEMENT_3D ( 'NONE', #35694, #32066, #35909 ) ;
#28845=CARTESIAN_POINT ( 'NONE',  ( -47.64484625134591766, 19.26749830283604936, -4.730721332201286877 ) ) ;
#28846=ORIENTED_EDGE ( 'NONE', *, *, #27268, .F. ) ;
#28847=DIRECTION ( 'NONE',  ( -0.8745520943968245753, 0.4849315768086539524, -5.691349986800526185E-16 ) ) ;
#28849=CARTESIAN_POINT ( 'NONE',  ( -49.57073425708396286, 16.97194942007707752, 5.013496192390408446 ) ) ;
#28852=CARTESIAN_POINT ( 'NONE',  ( -55.80532936045742787, 9.325833942462050885, 0.2199084463661053201 ) ) ;
#28854=VERTEX_POINT ( 'NONE', #324 ) ;
#28855=CARTESIAN_POINT ( 'NONE',  ( -52.96141808003752516, 14.46028723511719960, -2.643142726894160521 ) ) ;
#28857=DIRECTION ( 'NONE',  ( -0.8745520943968235761, 0.4849315768086558398, -5.691349986800547879E-16 ) ) ;
#28858=ORIENTED_EDGE ( 'NONE', *, *, #30810, .F. ) ;
#28861=CIRCLE ( 'NONE', #38395, 0.2539999999999998925 ) ;
#28864=DIRECTION ( 'NONE',  ( -0.8745520943968235761, 0.4849315768086558398, -5.691349986800547879E-16 ) ) ;
#28871=DIRECTION ( 'NONE',  ( -0.8745520943968235761, 0.4849315768086558953, -5.361993529360570985E-16 ) ) ;
#28872=ORIENTED_EDGE ( 'NONE', *, *, #21522, .T. ) ;
#28874=ORIENTED_EDGE ( 'NONE', *, *, #19947, .T. ) ;
#28882=FACE_OUTER_BOUND ( 'NONE', #19126, .T. ) ;
#28886=DIRECTION ( 'NONE',  ( -0.8745520943968361216, 0.4849315768086333023, -6.829619984160648185E-16 ) ) ;
#28887=CARTESIAN_POINT ( 'NONE',  ( -46.67659519887700981, 22.71018310752411651, -3.598098858967615055 ) ) ;
#28888=ORIENTED_EDGE ( 'NONE', *, *, #39258, .T. ) ;
#28896=DIRECTION ( 'NONE',  ( -0.8745520943968225769, 0.4849315768086578382, -5.691349986800571545E-16 ) ) ;
#28898=VERTEX_POINT ( 'NONE', #26276 ) ;
#28906=FACE_OUTER_BOUND ( 'NONE', #40110, .T. ) ;
#28908=CARTESIAN_POINT ( 'NONE',  ( -8.519412162535125788, 69.40335734044577976, -1.523999999999996025 ) ) ;
#28913=FACE_OUTER_BOUND ( 'NONE', #15174, .T. ) ;
#28921=CARTESIAN_POINT ( 'NONE',  ( -26.51793118801306548, 72.98537704160715123, 1.269999999999993134 ) ) ;
#28934=CARTESIAN_POINT ( 'NONE',  ( -46.60530155212504155, 26.17382724835477248, 0.2116666666666584817 ) ) ;
#28936=CARTESIAN_POINT ( 'NONE',  ( -47.61549956331938915, 19.66157307908738261, 5.197827534590556908 ) ) ;
#28937=CARTESIAN_POINT ( 'NONE',  ( -58.65723136083905587, -0.3152049157291291204, 0.3253893282242821261 ) ) ;
#28938=ADVANCED_FACE ( 'NONE', ( #20290 ), #19169, .T. ) ;
#28940=B_SPLINE_SURFACE_WITH_KNOTS ( 'NONE', 3, 3, ( 
 ( #10616, #33424, #23598, #14017, #30213 ),
 ( #30003, #24020, #16797, #20397, #7647 ),
 ( #36619, #7019, #26598, #33216, #13815 ),
 ( #37038, #23163, #36413, #33843, #4042 ),
 ( #4253, #14221, #36829, #7438, #17216 ),
 ( #20605, #1266, #1053, #36198, #13607 ),
 ( #637, #19987, #39605, #7856, #13395 ),
 ( #33637, #10408, #20191, #33004, #27024 ),
 ( #11038, #40032, #10825, #39822, #17003 ),
 ( #842, #23808, #4464, #3833, #17421 ),
 ( #26814, #27230, #40244, #20817, #17627 ),
 ( #425, #26383, #24645, #5298, #38079 ),
 ( #34672, #5718, #24433, #21436, #40857 ),
 ( #8894, #27639, #11660, #14429, #18246 ),
 ( #21862, #24228, #37656, #18461, #28275 ),
 ( #14637, #8480, #18044, #11243, #34465 ),
 ( #5502, #5091, #40652, #31045, #24866 ),
 ( #41280, #27437, #1683, #41066, #34887 ),
 ( #37862, #8686, #17837, #31251, #34052 ),
 ( #34262, #21648, #30629, #1884, #31466 ),
 ( #11445, #2309, #25074, #27850, #14846 ),
 ( #40452, #37438, #1472, #37238, #8260 ),
 ( #28057, #8056, #15269, #11877, #2093 ),
 ( #15057, #21029, #21233, #12086, #4882 ),
 ( #30835, #15486, #115, #10517, #9881 ),
 ( #10094, #33112, #13509, #29485, #36100 ),
 ( #39502, #20089, #23067, #29056, #32471 ),
 ( #6486, #38865, #3301, #26711, #31681 ),
 ( #26498, #19462, #16265, #42075, #6914 ),
 ( #29904, #3731, #13293, #16480, #29268 ),
 ( #13079, #19884, #32899, #12869, #23276 ),
 ( #22852, #19670, #22641, #25857, #35891 ),
 ( #326, #26069, #32684, #39079, #16902 ),
 ( #3519, #9676, #39717, #10308, #3942 ),
 ( #36312, #7132, #6701, #35677, #26279 ),
 ( #39288, #16688, #742, #29694, #2523 ),
 ( #535, #13717, #23488, #36514, #18674 ),
 ( #11354, #23920, #4365, #36936, #1583 ),
 ( #17946, #4149, #20505, #17734, #14750 ) ),
 .UNSPECIFIED., .F., .F., .F.,
 ( 4, 1, 1, 1, 1, 1, 1, 1, 1, 1, 1, 2, 1, 1, 1, 1, 1, 1, 1, 1, 1, 1, 1, 1, 1, 1, 1, 1, 1, 1, 1, 1, 1, 1, 1, 4 ),
 ( 4, 1, 4 ),
 ( 0.000000000000000000, 0.01653533301974152367, 0.03307066603948304734, 0.04960599905922460223, 0.06614133207896609468, 0.08267666509870763569, 0.09921199811844919059, 0.1322826641579321894, 0.1653533301974152714, 0.1984239962368983812, 0.2314946622763813522, 0.2645653283158643787, 0.3105299952961229071, 0.3335123287862520880, 0.3564946622763812689, 0.4024593292566397418, 0.4484239962368982702, 0.4943886632171566875, 0.5403533301974150493, 0.5863179971776735222, 0.6322826641579321061, 0.6782473311381906900, 0.7242119981184491628, 0.7701766650987074136, 0.8161413320789658865, 0.8621059990592241373, 0.8735971658042887000, 0.8850883325493537068, 0.8965794992944182695, 0.9080706660394826102, 0.9195618327845473949, 0.9310529995296121797, 0.9425441662746769644, 0.9540353330197415271, 0.9770176665098706525, 1.000000000000000000 ),
 ( 0.000000000000000000, 0.5000000000000000000, 1.000000000000000000 ),
 .UNSPECIFIED. ) ;
#28941=ORIENTED_EDGE ( 'NONE', *, *, #40560, .T. ) ;
#28953=EDGE_CURVE ( 'NONE', #38617, #14467, #39077, .T. ) ;
#28956=CIRCLE ( 'NONE', #3812, 2.539999999999996483 ) ;
#28960=EDGE_LOOP ( 'NONE', ( #8166, #13120, #29543, #23541 ) ) ;
#28961=DIRECTION ( 'NONE',  ( -0.2883665106726583938, -0.9575201071113210727, 0.000000000000000000 ) ) ;
#28966=ORIENTED_EDGE ( 'NONE', *, *, #10952, .T. ) ;
#28967=ORIENTED_EDGE ( 'NONE', *, *, #22006, .T. ) ;
#28968=CYLINDRICAL_SURFACE ( 'NONE', #16737, 0.2539999999999997260 ) ;
#28974=CARTESIAN_POINT ( 'NONE',  ( -48.03056308610731406, 19.49280019387112972, -5.381938484679579915 ) ) ;
#28977=EDGE_CURVE ( 'NONE', #34270, #3266, #10306, .T. ) ;
#28979=ORIENTED_EDGE ( 'NONE', *, *, #34248, .F. ) ;
#28980=CARTESIAN_POINT ( 'NONE',  ( -17.14500000000466784, 71.11999999999886768, -1.524000000000000909 ) ) ;
#28983=EDGE_CURVE ( 'NONE', #33959, #38171, #41635, .T. ) ;
#28984=VECTOR ( 'NONE', #25411, 1000.000000000000114 ) ;
#28986=AXIS2_PLACEMENT_3D ( 'NONE', #8973, #31542, #21940 ) ;
#29000=CARTESIAN_POINT ( 'NONE',  ( -15.27962295839633811, 80.49293118800726177, -1.524000000000001576 ) ) ;
#29001=DIRECTION ( 'NONE',  ( -0.9998501190848629872, -0.01731298258490734585, -8.537024980200777445E-16 ) ) ;
#29012=CARTESIAN_POINT ( 'NONE',  ( -43.40712238249138011, 21.47926646521734639, -2.288489392298376668 ) ) ;
#29017=CARTESIAN_POINT ( 'NONE',  ( -55.11053650837317974, 7.076797490156363502, -3.243731704390616866 ) ) ;
#29020=CARTESIAN_POINT ( 'NONE',  ( -57.45676042280280171, 1.677525466749221650, -1.437765377950721346 ) ) ;
#29028=CARTESIAN_POINT ( 'NONE',  ( -57.93941708942283952, 2.052042089854988483, -1.628789306319529118 ) ) ;
#29032=VERTEX_POINT ( 'NONE', #26709 ) ;
#29036=VECTOR ( 'NONE', #1761, 1000.000000000000114 ) ;
#29037=EDGE_CURVE ( 'NONE', #29982, #332, #30719, .T. ) ;
#29038=CARTESIAN_POINT ( 'NONE',  ( -57.22211421646275653, 1.778355698664441098, -1.009576694067165286E-14 ) ) ;
#29039=EDGE_CURVE ( 'NONE', #28714, #1088, #38863, .T. ) ;
#29042=CARTESIAN_POINT ( 'NONE',  ( -46.96231544241641842, 24.98353995950040840, 1.991484372665509595 ) ) ;
#29046=DIRECTION ( 'NONE',  ( 5.188838149069472160E-16, -1.699382548006136559E-16, -1.000000000000000000 ) ) ;
#29048=CARTESIAN_POINT ( 'NONE',  ( -45.23155955595164812, 20.39474799592974463, -2.956275845755119924 ) ) ;
#29050=CARTESIAN_POINT ( 'NONE',  ( -46.60530155212503445, 26.17382724835477958, -1.270000000000008233 ) ) ;
#29051=CARTESIAN_POINT ( 'NONE',  ( -51.04632475015682047, 14.57504837431617339, 4.679247123343607484 ) ) ;
#29053=CARTESIAN_POINT ( 'NONE',  ( -27.88833342972739615, 78.11058938209563962, 1.269999999999991580 ) ) ;
#29055=CARTESIAN_POINT ( 'NONE',  ( -56.90576330281450623, 4.524090327013369439, 2.207515467630526196 ) ) ;
#29056=CARTESIAN_POINT ( 'NONE',  ( -56.82628769568140115, 4.502340570254503405, 2.499646007873237430 ) ) ;
#29059=CARTESIAN_POINT ( 'NONE',  ( -53.63638764239521350, 11.23543775674477807, -3.971736527645129744 ) ) ;
#29084=CARTESIAN_POINT ( 'NONE',  ( -13.79703500197642896, 79.79115557309579287, -1.270000000000000462 ) ) ;
#29092=CARTESIAN_POINT ( 'NONE',  ( -46.68395179480138779, 26.03198510454123848, -1.524000000000008459 ) ) ;
#29093=VERTEX_POINT ( 'NONE', #1786 ) ;
#29096=CARTESIAN_POINT ( 'NONE',  ( -10.53334313995851446, 65.32054992887103140, -1.269999999999996465 ) ) ;
#29097=AXIS2_PLACEMENT_3D ( 'NONE', #12217, #31602, #5636 ) ;
#29106=EDGE_LOOP ( 'NONE', ( #26032, #38316, #34800, #29882 ) ) ;
#29111=CARTESIAN_POINT ( 'NONE',  ( -5.878298779570172883, 78.21245918282636467, -1.523999999999996247 ) ) ;
#29113=ORIENTED_EDGE ( 'NONE', *, *, #8114, .F. ) ;
#29118=DIRECTION ( 'NONE',  ( 0.8745520943968240202, -0.4849315768086551182, 4.268512490100404500E-16 ) ) ;
#29127=ORIENTED_EDGE ( 'NONE', *, *, #4770, .F. ) ;
#29130=FACE_OUTER_BOUND ( 'NONE', #4620, .T. ) ;
#29136=AXIS2_PLACEMENT_3D ( 'NONE', #32625, #22378, #28801 ) ;
#29142=CARTESIAN_POINT ( 'NONE',  ( -50.47475848037564816, 15.37778258171979218, 4.692728031515248865 ) ) ;
#29143=CARTESIAN_POINT ( 'NONE',  ( -46.81070079724250377, 25.76746909427398435, 1.215830024444411572 ) ) ;
#29145=CARTESIAN_POINT ( 'NONE',  ( -42.33919149967392315, 22.05006338260229271, 1.842566675324087022 ) ) ;
#29146=DIRECTION ( 'NONE',  ( 5.188838149069472160E-16, -1.699382548006136559E-16, -1.000000000000000000 ) ) ;
#29149=ORIENTED_EDGE ( 'NONE', *, *, #31878, .F. ) ;
#29152=AXIS2_PLACEMENT_3D ( 'NONE', #9669, #41433, #12452 ) ;
#29161=CARTESIAN_POINT ( 'NONE',  ( -47.85244527695896011, 19.39403540832957518, 5.219971639306693056 ) ) ;
#29171=DIRECTION ( 'NONE',  ( 5.188838149069472160E-16, -1.699382548006136559E-16, -1.000000000000000000 ) ) ;
#29179=CARTESIAN_POINT ( 'NONE',  ( -41.98003980773050614, 22.15641273310255954, 0.9734550245784977518 ) ) ;
#29186=CARTESIAN_POINT ( 'NONE',  ( -10.75478607932181241, 82.07015292912137738, -1.523999999999999355 ) ) ;
#29187=ADVANCED_FACE ( 'NONE', ( #7754 ), #27989, .T. ) ;
#29191=ORIENTED_EDGE ( 'NONE', *, *, #24135, .T. ) ;
#29194=CIRCLE ( 'NONE', #12862, 0.2539999999999997260 ) ;
#29200=FACE_OUTER_BOUND ( 'NONE', #19481, .T. ) ;
#29205=EDGE_CURVE ( 'NONE', #21592, #32447, #33743, .T. ) ;
#29214=CARTESIAN_POINT ( 'NONE',  ( -47.04837031381860157, 23.61299024743492581, -3.054033755318078303 ) ) ;
#29221=EDGE_LOOP ( 'NONE', ( #22060, #26285, #41279, #21472 ) ) ;
#29223=AXIS2_PLACEMENT_3D ( 'NONE', #20201, #3629, #39401 ) ;
#29231=CARTESIAN_POINT ( 'NONE',  ( -58.80444036411011410, -0.2843080703047338176, -0.1310653756851450913 ) ) ;
#29232=EDGE_LOOP ( 'NONE', ( #4200, #14517, #30867, #10984 ) ) ;
#29236=LINE ( 'NONE', #6672, #4145 ) ;
#29239=CARTESIAN_POINT ( 'NONE',  ( -57.29531047346088712, 2.067549486662559222, -1.749273462387503031 ) ) ;
#29247=B_SPLINE_CURVE_WITH_KNOTS ( 'NONE', 3,
 ( #21658, #5512, #5728, #14439, #27449, #40464, #11254 ),
 .UNSPECIFIED., .F., .F.,
 ( 4, 3, 4 ),
 ( 0.000000000000000000, 6.533385608969465084E-05, 6.539385608967072667E-05 ),
 .UNSPECIFIED. ) ;
#29252=CARTESIAN_POINT ( 'NONE',  ( -46.60530155212504155, 26.17382724835477958, 1.269999999999990692 ) ) ;
#29255=LINE ( 'NONE', #18823, #18093 ) ;
#29257=CARTESIAN_POINT ( 'NONE',  ( -48.46138709710082537, 15.22468166490328123, -0.8008350491754933076 ) ) ;
#29258=ORIENTED_EDGE ( 'NONE', *, *, #22738, .T. ) ;
#29260=CARTESIAN_POINT ( 'NONE',  ( -47.84356795211461844, 19.38525671449500010, -5.197506975155170572 ) ) ;
#29262=CARTESIAN_POINT ( 'NONE',  ( -33.42971872652992005, 49.93539301574497102, 1.269999999999992468 ) ) ;
#29264=CIRCLE ( 'NONE', #6170, 0.5080000000000000071 ) ;
#29267=CARTESIAN_POINT ( 'NONE',  ( -54.55302389503632554, 12.80492160976152327, 0.5954867740797897824 ) ) ;
#29268=CARTESIAN_POINT ( 'NONE',  ( -57.66338803320029882, 2.692357263605615891, 1.869785753600835987 ) ) ;
#29271=CARTESIAN_POINT ( 'NONE',  ( -55.38777061991515183, 7.924152594517688719, -2.969223861581061996 ) ) ;
#29273=ADVANCED_FACE ( 'NONE', ( #17323 ), #2197, .T. ) ;
#29274=ORIENTED_EDGE ( 'NONE', *, *, #14081, .T. ) ;
#29275=DIRECTION ( 'NONE',  ( 5.188838149069472160E-16, -1.699382548006136559E-16, -1.000000000000000000 ) ) ;
#29276=TOROIDAL_SURFACE ( 'NONE', #10908, 0.3809999999999993947, 0.2540000000000000036 ) ;
#29280=CARTESIAN_POINT ( 'NONE',  ( -31.59722765895411101, 71.22255575826451945, 1.523999999999991140 ) ) ;
#29284=CARTESIAN_POINT ( 'NONE',  ( -41.28107547821696954, 23.22158991241121839, -1.270000000000005125 ) ) ;
#29287=CARTESIAN_POINT ( 'NONE',  ( -17.14500000000466784, 71.11999999999886768, -1.270000000000000684 ) ) ;
#29289=ORIENTED_EDGE ( 'NONE', *, *, #1147, .T. ) ;
#29292=CARTESIAN_POINT ( 'NONE',  ( -58.30309248033832858, -0.1506202810087469701, -0.3290154619008041070 ) ) ;
#29299=AXIS2_PLACEMENT_3D ( 'NONE', #36554, #33357, #17563 ) ;
#29300=DIRECTION ( 'NONE',  ( -0.8745520943968235761, 0.4849315768086558398, -5.691349986800547879E-16 ) ) ;
#29303=ORIENTED_EDGE ( 'NONE', *, *, #35725, .F. ) ;
#29307=TOROIDAL_SURFACE ( 'NONE', #40927, 0.3810000000000001719, 0.2540000000000000036 ) ;
#29308=CARTESIAN_POINT ( 'NONE',  ( -48.16508968810062896, 19.01313136326716347, -5.219744232931991412 ) ) ;
#29310=PRODUCT ( 'Wing Lever', 'Wing Lever', '', ( #37064 ) ) ;
#29313=TOROIDAL_SURFACE ( 'NONE', #10938, 0.3809999999999999498, 0.2540000000000000036 ) ;
#29319=CARTESIAN_POINT ( 'NONE',  ( -17.14500000000466784, 71.11999999999886768, 1.523999999999998689 ) ) ;
#29320=CARTESIAN_POINT ( 'NONE',  ( -11.56352105402813280, 78.55269139521317356, -1.269999999999998908 ) ) ;
#29322=ORIENTED_EDGE ( 'NONE', *, *, #17768, .T. ) ;
#29328=AXIS2_PLACEMENT_3D ( 'NONE', #25573, #28565, #38577 ) ;
#29330=ADVANCED_FACE ( 'NONE', ( #14539 ), #17161, .T. ) ;
#29332=VERTEX_POINT ( 'NONE', #21130 ) ;
#29336=FACE_OUTER_BOUND ( 'NONE', #4342, .T. ) ;
#29343=VECTOR ( 'NONE', #29985, 1000.000000000000000 ) ;
#29346=ORIENTED_EDGE ( 'NONE', *, *, #2160, .T. ) ;
#29356=VECTOR ( 'NONE', #27488, 1000.000000000000227 ) ;
#29362=CARTESIAN_POINT ( 'NONE',  ( -52.36976898921572143, 11.96785871290047787, 4.095024579493532713 ) ) ;
#29363=CARTESIAN_POINT ( 'NONE',  ( -49.10997966587441965, 20.64911895071488956, 3.108984601230522671 ) ) ;
#29365=CARTESIAN_POINT ( 'NONE',  ( -51.81113891419111894, 13.24950054771400332, 4.495723625053109629 ) ) ;
#29369=ORIENTED_EDGE ( 'NONE', *, *, #34191, .T. ) ;
#29375=CARTESIAN_POINT ( 'NONE',  ( -46.60530155212504155, 26.17382724835476537, -0.4656666666666756105 ) ) ;
#29379=DIRECTION ( 'NONE',  ( -0.7308269722843410143, 0.6825627711659222330, -8.537024980200883941E-16 ) ) ;
#29398=CARTESIAN_POINT ( 'NONE',  ( -42.83068693079387401, 21.70476352389080787, 1.889833665869958157 ) ) ;
#29412=CARTESIAN_POINT ( 'NONE',  ( -38.65395868481546415, 29.38327706004843876, -1.524000000000004906 ) ) ;
#29413=CARTESIAN_POINT ( 'NONE',  ( -58.13403979463087268, 0.7724927387386393285, 1.216435378341239382 ) ) ;
#29419=DIRECTION ( 'NONE',  ( 0.9816537812491076265, 0.1906721105965138718, 4.769617732184456426E-16 ) ) ;
#29430=DIRECTION ( 'NONE',  ( -0.4849315768086534528, -0.8745520943968250194, -1.030032898892974942E-16 ) ) ;
#29433=ADVANCED_FACE ( 'NONE', ( #951 ), #864, .T. ) ;
#29437=AXIS2_PLACEMENT_3D ( 'NONE', #33156, #3772, #10972 ) ;
#29440=ORIENTED_EDGE ( 'NONE', *, *, #38665, .T. ) ;
#29441=CARTESIAN_POINT ( 'NONE',  ( -17.64950171984354554, 84.16951713491046405, 1.269999999999996243 ) ) ;
#29446=CARTESIAN_POINT ( 'NONE',  ( -58.72763989320913680, -0.3148928600554901092, -0.2588867910284781138 ) ) ;
#29450=DIRECTION ( 'NONE',  ( -0.01731298258488003436, 0.9998501190848634312, 0.000000000000000000 ) ) ;
#29455=CARTESIAN_POINT ( 'NONE',  ( -57.80205714066466527, 2.371715784325115095, -1.753227392946310470 ) ) ;
#29464=CIRCLE ( 'NONE', #1606, 0.2540000000000000036 ) ;
#29472=DIRECTION ( 'NONE',  ( -0.9575201071113178530, 0.2883665106726683858, -8.537024980200786319E-16 ) ) ;
#29473=CARTESIAN_POINT ( 'NONE',  ( -48.25086062633820916, 17.91646674446130305, -3.976701633436076300 ) ) ;
#29475=DIRECTION ( 'NONE',  ( 0.4849315768086535638, 0.8745520943968251304, 1.030032898892975065E-16 ) ) ;
#29476=CIRCLE ( 'NONE', #19958, 0.2539999999999998925 ) ;
#29477=CARTESIAN_POINT ( 'NONE',  ( -46.77395155747410627, 25.81392106044808799, -1.433409421412224827 ) ) ;
#29478=CARTESIAN_POINT ( 'NONE',  ( -33.42971872652992005, 49.93539301574497102, -1.270000000000005569 ) ) ;
#29481=DIRECTION ( 'NONE',  ( 5.188838149069471174E-16, -1.699382548006136313E-16, -1.000000000000000000 ) ) ;
#29482=DIRECTION ( 'NONE',  ( 5.188838149069472160E-16, -1.699382548006136559E-16, -1.000000000000000000 ) ) ;
#29483=CARTESIAN_POINT ( 'NONE',  ( -56.91937565786339803, 5.591339438888828894, -1.031528444718396757E-14 ) ) ;
#29484=ADVANCED_FACE ( 'NONE', ( #28387 ), #18574, .T. ) ;
#29485=CARTESIAN_POINT ( 'NONE',  ( -56.22331024217277928, 5.808995339285999648, 2.850545730341239814 ) ) ;
#29489=CARTESIAN_POINT ( 'NONE',  ( -54.06930887699937216, 11.98206827348202808, -2.380698788532477295 ) ) ;
#29504=EDGE_CURVE ( 'NONE', #20165, #37020, #8466, .T. ) ;
#29506=ORIENTED_EDGE ( 'NONE', *, *, #4770, .T. ) ;
#29508=ORIENTED_EDGE ( 'NONE', *, *, #38131, .T. ) ;
#29510=CARTESIAN_POINT ( 'NONE',  ( -58.36980953069939915, -0.2915895811168507379, -0.001722197669518234003 ) ) ;
#29519=ORIENTED_EDGE ( 'NONE', *, *, #5838, .F. ) ;
#29524=CARTESIAN_POINT ( 'NONE',  ( -46.97515415817095175, 24.89137758704647396, -2.045406795549908896 ) ) ;
#29526=VECTOR ( 'NONE', #30106, 1000.000000000000000 ) ;
#29529=ADVANCED_FACE ( 'NONE', ( #28173, #31792 ), #31365, .F. ) ;
#29531=VECTOR ( 'NONE', #30882, 1000.000000000000000 ) ;
#29539=CYLINDRICAL_SURFACE ( 'NONE', #35819, 0.2540000000000051106 ) ;
#29542=EDGE_CURVE ( 'NONE', #33508, #35910, #16458, .T. ) ;
#29543=ORIENTED_EDGE ( 'NONE', *, *, #23787, .F. ) ;
#29546=CIRCLE ( 'NONE', #24756, 0.7619999999999984563 ) ;
#29552=EDGE_LOOP ( 'NONE', ( #23461, #35630, #39110, #8378 ) ) ;
#29564=ORIENTED_EDGE ( 'NONE', *, *, #11385, .F. ) ;
#29565=CARTESIAN_POINT ( 'NONE',  ( -19.64403260974359355, 72.50569198072959409, -1.270000000000002238 ) ) ;
#29574=FACE_OUTER_BOUND ( 'NONE', #31201, .T. ) ;
#29579=EDGE_CURVE ( 'NONE', #18130, #24697, #41604, .T. ) ;
#29582=CARTESIAN_POINT ( 'NONE',  ( -46.75382734339789437, 25.86353334213626098, 1.406704986510833866 ) ) ;
#29583=CARTESIAN_POINT ( 'NONE',  ( -48.77319768356018415, 22.00425556813275563, 2.071420771163280605 ) ) ;
#29585=CARTESIAN_POINT ( 'NONE',  ( -53.09398923718962493, 10.65108322687173548, 3.938325876039757478 ) ) ;
#29586=DIRECTION ( 'NONE',  ( -5.188838149069472160E-16, 1.699382548006136559E-16, 1.000000000000000000 ) ) ;
#29588=CARTESIAN_POINT ( 'NONE',  ( -58.37241122568484286, -0.2962816677227336770, -1.028586707908061473E-14 ) ) ;
#29590=VERTEX_POINT ( 'NONE', #9009 ) ;
#29595=CARTESIAN_POINT ( 'NONE',  ( -46.98785713747574277, 25.41845405000909253, -0.7790854875835228066 ) ) ;
#29615=CARTESIAN_POINT ( 'NONE',  ( -46.29506748884626433, 20.38262349295737152, 4.279265904994557168 ) ) ;
#29622=CARTESIAN_POINT ( 'NONE',  ( -9.960492004070040650, 64.81807050032566053, -1.269999999999996021 ) ) ;
#29626=VERTEX_POINT ( 'NONE', #5825 ) ;
#29629=EDGE_CURVE ( 'NONE', #40015, #2780, #36888, .T. ) ;
#29637=VECTOR ( 'NONE', #32320, 1000.000000000000114 ) ;
#29642=CYLINDRICAL_SURFACE ( 'NONE', #38815, 0.2540000000000027236 ) ;
#29646=CARTESIAN_POINT ( 'NONE',  ( -8.095114962461808616, 74.19100168833409725, -1.269999999999996687 ) ) ;
#29647=DIRECTION ( 'NONE',  ( 0.7284927773988636446, 0.6850534820564666560, -1.946650227582177166E-16 ) ) ;
#29653=FACE_OUTER_BOUND ( 'NONE', #34335, .T. ) ;
#29661=FACE_OUTER_BOUND ( 'NONE', #20989, .T. ) ;
#29668=CARTESIAN_POINT ( 'NONE',  ( -58.75009580408200094, 0.1057190229620807997, -0.6617493214611014363 ) ) ;
#29672=ORIENTED_EDGE ( 'NONE', *, *, #35773, .F. ) ;
#29676=CARTESIAN_POINT ( 'NONE',  ( -58.33068375617610002, -0.2093732065610448556, 0.2478323015012930397 ) ) ;
#29683=CARTESIAN_POINT ( 'NONE',  ( -55.66968704194594153, 5.419822863896792242, -2.567922718055084541 ) ) ;
#29686=CARTESIAN_POINT ( 'NONE',  ( -46.70678165893853162, 25.97453801526106787, -1.349345659034532074 ) ) ;
#29688=FACE_OUTER_BOUND ( 'NONE', #2885, .T. ) ;
#29690=FACE_OUTER_BOUND ( 'NONE', #9679, .T. ) ;
#29692=CARTESIAN_POINT ( 'NONE',  ( -57.78866059769681129, 2.451738602565561642, 1.593934435026631347 ) ) ;
#29693=AXIS2_PLACEMENT_3D ( 'NONE', #3683, #33702, #1326 ) ;
#29694=CARTESIAN_POINT ( 'NONE',  ( -58.55221842960730783, 0.5754175076986972615, 0.9757793345693576148 ) ) ;
#29697=CARTESIAN_POINT ( 'NONE',  ( -50.94572941386617515, 18.90544291192138004, -2.223209376321594100 ) ) ;
#29699=ORIENTED_EDGE ( 'NONE', *, *, #8405, .T. ) ;
#29700=DIRECTION ( 'NONE',  ( -0.6294287539884059202, -0.7770581983690814099, -1.945484789722797322E-16 ) ) ;
#29707=CARTESIAN_POINT ( 'NONE',  ( -29.48469873830907417, 60.47150940315087553, 1.269999999999993356 ) ) ;
#29711=CYLINDRICAL_SURFACE ( 'NONE', #28841, 0.2539999999999956737 ) ;
#29713=ORIENTED_EDGE ( 'NONE', *, *, #15168, .T. ) ;
#29715=CARTESIAN_POINT ( 'NONE',  ( -58.06266446028805461, 0.3686289127265512389, -0.7729225178788856621 ) ) ;
#29728=AXIS2_PLACEMENT_3D ( 'NONE', #17819, #30819, #15255 ) ;
#29732=CARTESIAN_POINT ( 'NONE',  ( -44.96292901393739072, 21.56701576681934540, -3.486870777078513228 ) ) ;
#29733=VECTOR ( 'NONE', #40962, 1000.000000000000000 ) ;
#29744=EDGE_LOOP ( 'NONE', ( #29508, #971, #7574, #41867 ) ) ;
#29746=TOROIDAL_SURFACE ( 'NONE', #21535, 8.794749999999998735, 0.2540000000000000036 ) ;
#29748=VERTEX_POINT ( 'NONE', #27957 ) ;
#29749=EDGE_CURVE ( 'NONE', #15081, #21468, #40965, .T. ) ;
#29751=CARTESIAN_POINT ( 'NONE',  ( -46.72577905453591285, 25.95655153957431338, -1.270000040519894347 ) ) ;
#29755=CARTESIAN_POINT ( 'NONE',  ( -41.28107547821698375, 23.22158991241121129, 1.523999999999985366 ) ) ;
#29759=ADVANCED_FACE ( 'NONE', ( #39664 ), #38813, .F. ) ;
#29761=CARTESIAN_POINT ( 'NONE',  ( -41.28107547821692691, 23.22158991241129300, -1.523999999999999355 ) ) ;
#29769=LINE ( 'NONE', #26352, #39269 ) ;
#29773=ORIENTED_EDGE ( 'NONE', *, *, #11795, .T. ) ;
#29774=ORIENTED_EDGE ( 'NONE', *, *, #28421, .T. ) ;
#29777=DIRECTION ( 'NONE',  ( 5.188838149069472160E-16, -1.699382548006136559E-16, -1.000000000000000000 ) ) ;
#29789=CARTESIAN_POINT ( 'NONE',  ( -48.52081263401391453, 18.50387112158377789, 5.159775967924278284 ) ) ;
#29790=CARTESIAN_POINT ( 'NONE',  ( -48.57235503434458224, 24.64055110436136431, 0.2038152558994842933 ) ) ;
#29792=CARTESIAN_POINT ( 'NONE',  ( -52.42133349025997546, 11.92692459785933679, 4.172736198742178715 ) ) ;
#29793=CARTESIAN_POINT ( 'NONE',  ( -57.27125839519965922, 2.624645228885598147, 1.995972916280581710 ) ) ;
#29797=EDGE_LOOP ( 'NONE', ( #1958, #14872, #28699, #40099 ) ) ;
#29823=CARTESIAN_POINT ( 'NONE',  ( -47.44699234454018466, 15.94620872345373108, -6.997593760898217036E-15 ) ) ;
#29829=ADVANCED_FACE ( 'NONE', ( #16855 ), #19415, .F. ) ;
#29851=DIRECTION ( 'NONE',  ( -0.8745520943968229099, 0.4849315768086573386, -4.268512490100424221E-16 ) ) ;
#29859=DIRECTION ( 'NONE',  ( 0.7548010569845216011, 0.6559537821943318692, 2.801824109679581255E-16 ) ) ;
#29860=ORIENTED_EDGE ( 'NONE', *, *, #30470, .T. ) ;
#29862=ORIENTED_EDGE ( 'NONE', *, *, #27378, .F. ) ;
#29882=ORIENTED_EDGE ( 'NONE', *, *, #37318, .F. ) ;
#29885=CARTESIAN_POINT ( 'NONE',  ( -51.89660998226325006, 12.88425699701002003, 4.274492870955763912 ) ) ;
#29892=CIRCLE ( 'NONE', #3387, 8.794749999999995183 ) ;
#29893=CARTESIAN_POINT ( 'NONE',  ( -55.65298819915649631, 5.540485941798498182, -2.823722248809265256 ) ) ;
#29897=LINE ( 'NONE', #36506, #29526 ) ;
#29898=LINE ( 'NONE', #26909, #977 ) ;
#29899=CARTESIAN_POINT ( 'NONE',  ( -30.84292043869464095, 55.46612528701088962, -1.524000000001431099 ) ) ;
#29901=CARTESIAN_POINT ( 'NONE',  ( -26.51793118801306548, 72.98537704160715123, -1.524000000000006017 ) ) ;
#29903=CARTESIAN_POINT ( 'NONE',  ( -58.75091225067960465, 0.1325880516401256592, 0.03773457465073216249 ) ) ;
#29904=CARTESIAN_POINT ( 'NONE',  ( -57.15088083682995546, 2.378576142695001838, 1.865916551128045553 ) ) ;
#29907=CARTESIAN_POINT ( 'NONE',  ( -56.13924587166188473, 7.155854391526911051, -1.290439134121123432 ) ) ;
#29920=CARTESIAN_POINT ( 'NONE',  ( -48.51966762233396935, 18.52674309225730198, -5.186066996718803779 ) ) ;
#29921=CARTESIAN_POINT ( 'NONE',  ( -6.135835944515187101, 77.40800365160224317, -1.269999999999996243 ) ) ;
#29925=CARTESIAN_POINT ( 'NONE',  ( -57.89986051506333098, 0.7216312584049938694, -0.9866875624993080018 ) ) ;
#29931=AXIS2_PLACEMENT_3D ( 'NONE', #15465, #9300, #35286 ) ;
#29939=CARTESIAN_POINT ( 'NONE',  ( -49.39021242113546606, 17.77731941784099234, -5.290631085210052653 ) ) ;
#29942=DIRECTION ( 'NONE',  ( -0.8745520943968235761, 0.4849315768086558398, -5.691349986800547879E-16 ) ) ;
#29948=CARTESIAN_POINT ( 'NONE',  ( -42.19606231239111338, 22.08888036620076889, -1.545000424059316924 ) ) ;
#29952=EDGE_LOOP ( 'NONE', ( #21076, #39262, #41206, #28189, #4788 ) ) ;
#29958=CARTESIAN_POINT ( 'NONE',  ( -27.97106122948731155, 77.87043919753004673, -1.270000000000007345 ) ) ;
#29960=EDGE_CURVE ( 'NONE', #2316, #16908, #36219, .T. ) ;
#29969=CARTESIAN_POINT ( 'NONE',  ( -55.81791661756539469, 5.217579515133088819, -2.786573170153239243 ) ) ;
#29970=DIRECTION ( 'NONE',  ( -0.8745520943968245753, 0.4849315768086539524, -5.691349986800526185E-16 ) ) ;
#29974=TOROIDAL_SURFACE ( 'NONE', #37444, 0.3809999999999999498, 0.2540000000000000036 ) ;
#29978=VECTOR ( 'NONE', #8095, 1000.000000000000000 ) ;
#29979=CARTESIAN_POINT ( 'NONE',  ( -44.21430376968325504, 21.24218795319830022, 2.931160726117570725 ) ) ;
#29982=VERTEX_POINT ( 'NONE', #485 ) ;
#29985=DIRECTION ( 'NONE',  ( -5.188838149069471174E-16, 1.699382548006136313E-16, 1.000000000000000000 ) ) ;
#29988=ADVANCED_FACE ( 'NONE', ( #7078 ), #33060, .F. ) ;
#29993=CARTESIAN_POINT ( 'NONE',  ( -57.93112410002309787, 0.6539490773164662318, 0.9478910564283531404 ) ) ;
#29994=CARTESIAN_POINT ( 'NONE',  ( -49.15418877470109749, 24.05022684412165646, 0.2550087576077032514 ) ) ;
#29995=AXIS2_PLACEMENT_3D ( 'NONE', #32440, #35227, #25425 ) ;
#29997=CARTESIAN_POINT ( 'NONE',  ( -56.82628769568140115, 4.502340570254503405, 2.499646007873237430 ) ) ;
#29998=CARTESIAN_POINT ( 'NONE',  ( -56.63941872605137462, 3.954178040575838882, 2.419973308390618527 ) ) ;
#30000=DIRECTION ( 'NONE',  ( -5.188838149069472160E-16, 1.699382548006136559E-16, 1.000000000000000000 ) ) ;
#30002=ORIENTED_EDGE ( 'NONE', *, *, #21370, .T. ) ;
#30003=CARTESIAN_POINT ( 'NONE',  ( -41.18107378286554621, 22.95619949144852967, 1.523999999999987143 ) ) ;
#30006=VECTOR ( 'NONE', #9147, 1000.000000000000227 ) ;
#30025=VERTEX_POINT ( 'NONE', #32215 ) ;
#30026=ADVANCED_FACE ( 'NONE', ( #34111 ), #41663, .T. ) ;
#30027=CARTESIAN_POINT ( 'NONE',  ( -47.25474348537468927, 18.41641806589853303, 3.087470713317412851 ) ) ;
#30045=LINE ( 'NONE', #33255, #20496 ) ;
#30048=DIRECTION ( 'NONE',  ( -0.9336303900108815501, -0.3582377630124009560, -4.235673982319039874E-16 ) ) ;
#30049=CIRCLE ( 'NONE', #21843, 0.6350000000000014522 ) ;
#30052=DIRECTION ( 'NONE',  ( 5.188838149069472160E-16, -1.699382548006136559E-16, -1.000000000000000000 ) ) ;
#30054=VERTEX_POINT ( 'NONE', #33695 ) ;
#30059=CIRCLE ( 'NONE', #1504, 0.5080000000000000071 ) ;
#30064=CARTESIAN_POINT ( 'NONE',  ( -4.416771755448872128, 71.99420641645033925, -1.523999999999994248 ) ) ;
#30070=CARTESIAN_POINT ( 'NONE',  ( -10.04123483169954234, 65.65183074430956367, 1.270000000000002904 ) ) ;
#30071=DIRECTION ( 'NONE',  ( 0.7770581983690836303, -0.6294287539884032556, 5.101669463485833779E-16 ) ) ;
#30077=EDGE_LOOP ( 'NONE', ( #38666, #40993, #34886, #25659 ) ) ;
#30078=DIRECTION ( 'NONE',  ( -0.8745520943968250194, 0.4849315768086532863, -5.361993529360574930E-16 ) ) ;
#30085=DIRECTION ( 'NONE',  ( 5.188838149069472160E-16, -1.699382548006136559E-16, -1.000000000000000000 ) ) ;
#30090=ORIENTED_EDGE ( 'NONE', *, *, #12295, .T. ) ;
#30094=CARTESIAN_POINT ( 'NONE',  ( -50.51080154062190530, 15.37413104945128595, 4.759117110738762868 ) ) ;
#30102=VECTOR ( 'NONE', #42004, 1000.000000000000227 ) ;
#30103=CARTESIAN_POINT ( 'NONE',  ( -55.69906247323991266, 5.207560852731635492, -2.143283491784350403 ) ) ;
#30105=CARTESIAN_POINT ( 'NONE',  ( -8.095114962461808616, 74.19100168833409725, 1.524000000000002686 ) ) ;
#30106=DIRECTION ( 'NONE',  ( 5.188838149069472160E-16, -1.699382548006136559E-16, -1.000000000000000000 ) ) ;
#30107=DIRECTION ( 'NONE',  ( -5.188838149069471174E-16, 1.699382548006136313E-16, 1.000000000000000000 ) ) ;
#30108=CARTESIAN_POINT ( 'NONE',  ( -32.57812072122469260, 51.47121137444911199, -1.524000000004977373 ) ) ;
#30110=CARTESIAN_POINT ( 'NONE',  ( -46.64075290549589425, 25.58044659150066735, 1.617434478680441767 ) ) ;
#30111=DIRECTION ( 'NONE',  ( -0.8745520943968249084, 0.4849315768086533418, -5.271987356194193006E-16 ) ) ;
#30112=CARTESIAN_POINT ( 'NONE',  ( -58.03428750496626520, 2.144022121626010247, -1.041663317983060951E-14 ) ) ;
#30115=ORIENTED_EDGE ( 'NONE', *, *, #32944, .T. ) ;
#30116=CARTESIAN_POINT ( 'NONE',  ( -55.80532936045742787, 9.325833942462050885, -0.2199084463661266087 ) ) ;
#30118=ORIENTED_EDGE ( 'NONE', *, *, #8613, .T. ) ;
#30124=TOROIDAL_SURFACE ( 'NONE', #9719, 8.794749999999996959, 0.2540000000000000036 ) ;
#30127=CARTESIAN_POINT ( 'NONE',  ( -29.24627908556541200, 62.62042691902884428, 1.269999999999994467 ) ) ;
#30132=VERTEX_POINT ( 'NONE', #41764 ) ;
#30135=CARTESIAN_POINT ( 'NONE',  ( -57.92524306007030077, 0.6666591521451983304, -0.9550055539480221123 ) ) ;
#30140=CARTESIAN_POINT ( 'NONE',  ( -43.87210973174860129, 22.05421410453335795, -2.454571855453439255 ) ) ;
#30141=CIRCLE ( 'NONE', #21964, 0.2539999999999931202 ) ;
#30143=CIRCLE ( 'NONE', #10398, 0.2539999999999973390 ) ;
#30150=CARTESIAN_POINT ( 'NONE',  ( -49.93490050754573417, 16.96705409125581099, -5.170188367178254474 ) ) ;
#30151=DIRECTION ( 'NONE',  ( 5.188838149069472160E-16, -1.699382548006136559E-16, -1.000000000000000000 ) ) ;
#30153=CARTESIAN_POINT ( 'NONE',  ( -7.994219716368544226, 68.36415334912796027, -1.523999999999995580 ) ) ;
#30159=CARTESIAN_POINT ( 'NONE',  ( -43.93237127071142822, 21.31409657049219675, -2.696834577195023286 ) ) ;
#30166=ORIENTED_EDGE ( 'NONE', *, *, #2434, .T. ) ;
#30171=CARTESIAN_POINT ( 'NONE',  ( -46.38316532014830074, 26.05065462784526176, 1.523999999999997357 ) ) ;
#30173=VERTEX_POINT ( 'NONE', #5981 ) ;
#30177=CARTESIAN_POINT ( 'NONE',  ( -46.60530155212503445, 26.17382724835477958, -1.524000000000008459 ) ) ;
#30178=VERTEX_POINT ( 'NONE', #31950 ) ;
#30182=CARTESIAN_POINT ( 'NONE',  ( -58.81784827865733689, -0.2724209480201578160, -0.09409996577202993373 ) ) ;
#30191=VECTOR ( 'NONE', #11081, 1000.000000000000000 ) ;
#30196=AXIS2_PLACEMENT_3D ( 'NONE', #26627, #4493, #10225 ) ;
#30197=CARTESIAN_POINT ( 'NONE',  ( -32.58208212396117176, 51.46406716590541919, -1.270000000000005347 ) ) ;
#30201=LINE ( 'NONE', #1041, #21269 ) ;
#30205=CARTESIAN_POINT ( 'NONE',  ( -57.59772826146109281, 1.374066163636324056, 1.306202371370214443 ) ) ;
#30206=CARTESIAN_POINT ( 'NONE',  ( -48.05877817626803505, 25.10121868647436472, -8.674011749334489717E-15 ) ) ;
#30208=CARTESIAN_POINT ( 'NONE',  ( -55.73247374733729487, 5.492406230130003841, 2.854677165782097514 ) ) ;
#30209=CARTESIAN_POINT ( 'NONE',  ( -58.64175687851415830, -0.3079593361096647497, 0.3457559927878634531 ) ) ;
#30212=ORIENTED_EDGE ( 'NONE', *, *, #2932, .F. ) ;
#30213=CARTESIAN_POINT ( 'NONE',  ( -46.60530155212503445, 26.17382724835477958, 1.523999999999991140 ) ) ;
#30219=CARTESIAN_POINT ( 'NONE',  ( -33.42971872652992005, 49.93539301574497102, 1.269999999999992690 ) ) ;
#30223=FACE_OUTER_BOUND ( 'NONE', #29221, .T. ) ;
#30224=DIRECTION ( 'NONE',  ( 0.7445787077807144438, 0.6675346791887304398, 0.000000000000000000 ) ) ;
#30235=CARTESIAN_POINT ( 'NONE',  ( -48.30662019010082986, 17.20352665082216248, 3.142973069415112786 ) ) ;
#30240=ORIENTED_EDGE ( 'NONE', *, *, #13172, .F. ) ;
#30244=DIRECTION ( 'NONE',  ( -5.188838149069472160E-16, 1.699382548006136559E-16, 1.000000000000000000 ) ) ;
#30246=ORIENTED_EDGE ( 'NONE', *, *, #35994, .F. ) ;
#30250=EDGE_CURVE ( 'NONE', #17866, #37655, #15786, .T. ) ;
#30253=DIRECTION ( 'NONE',  ( -0.8745520943968241312, 0.4849315768086548406, -5.691349986800536046E-16 ) ) ;
#30255=CARTESIAN_POINT ( 'NONE',  ( -23.24761240069422286, 77.83567810938664877, -1.524000000000005128 ) ) ;
#30265=DIRECTION ( 'NONE',  ( -0.8745520943968240202, 0.4849315768086551737, -5.361993529360572958E-16 ) ) ;
#30267=CARTESIAN_POINT ( 'NONE',  ( -4.416771755448872128, 71.99420641645033925, -1.269999999999994245 ) ) ;
#30274=CARTESIAN_POINT ( 'NONE',  ( -27.97106122948731510, 77.87043919753004673, -1.524000000000007571 ) ) ;
#30286=EDGE_CURVE ( 'NONE', #30808, #19349, #26689, .T. ) ;
#30289=DIRECTION ( 'NONE',  ( -5.188838149069472160E-16, 1.699382548006136559E-16, 1.000000000000000000 ) ) ;
#30290=ADVANCED_FACE ( 'NONE', ( #37713 ), #27361, .T. ) ;
#30293=ORIENTED_EDGE ( 'NONE', *, *, #1643, .T. ) ;
#30296=CARTESIAN_POINT ( 'NONE',  ( -58.34386316732113897, -0.2371896724559785508, 0.2005938501613158675 ) ) ;
#30297=CIRCLE ( 'NONE', #11271, 0.3810000000000015041 ) ;
#30304=DIRECTION ( 'NONE',  ( 0.3213437296502684171, -0.9469626219732514283, 0.000000000000000000 ) ) ;
#30305=CARTESIAN_POINT ( 'NONE',  ( -50.34589867275522579, 15.36027825638806910, -4.364407372394879303 ) ) ;
#30307=DIRECTION ( 'NONE',  ( -0.6294287539884060312, -0.7770581983690815209, -1.945484789722797568E-16 ) ) ;
#30310=CARTESIAN_POINT ( 'NONE',  ( -29.37490963522909482, 66.57792725179109539, -1.270000000000101714 ) ) ;
#30313=CARTESIAN_POINT ( 'NONE',  ( -58.55612285180489351, 0.6590214021355567109, -1.048931848374691032E-14 ) ) ;
#30318=CARTESIAN_POINT ( 'NONE',  ( -57.43227285409300009, 3.226759729073131133, -2.064049688025099361 ) ) ;
#30322=DIRECTION ( 'NONE',  ( 0.01731298258488772612, -0.9998501190848634312, 1.788962107505314851E-16 ) ) ;
#30331=AXIS2_PLACEMENT_3D ( 'NONE', #24375, #21169, #5026 ) ;
#30334=CARTESIAN_POINT ( 'NONE',  ( -57.41341003177868885, 1.770451042089750793, -1.474359099879954282 ) ) ;
#30338=CARTESIAN_POINT ( 'NONE',  ( -47.43570116002440784, 20.37060963802031566, -5.342502768866047802 ) ) ;
#30339=EDGE_CURVE ( 'NONE', #1088, #27648, #33482, .T. ) ;
#30343=ORIENTED_EDGE ( 'NONE', *, *, #28269, .F. ) ;
#30348=CARTESIAN_POINT ( 'NONE',  ( -51.58367816905025194, 14.91232437457545146, -4.609044670965841917 ) ) ;
#30357=AXIS2_PLACEMENT_3D ( 'NONE', #5445, #3092, #24807 ) ;
#30359=TOROIDAL_SURFACE ( 'NONE', #22857, 0.7620000000000000107, 0.2540000000000000036 ) ;
#30362=CARTESIAN_POINT ( 'NONE',  ( -58.12768216001780530, 0.1527613808938732554, 0.09815255304908361567 ) ) ;
#30365=CARTESIAN_POINT ( 'NONE',  ( -47.42394374581075311, 23.94708628835674702, -1.773793246466847773 ) ) ;
#30367=CARTESIAN_POINT ( 'NONE',  ( -46.58649794690502688, 25.68081001442151035, -1.571531081469065283 ) ) ;
#30368=ORIENTED_EDGE ( 'NONE', *, *, #20371, .F. ) ;
#30369=CARTESIAN_POINT ( 'NONE',  ( -10.75478607932181241, 82.07015292912137738, -1.269999999999999130 ) ) ;
#30375=ORIENTED_EDGE ( 'NONE', *, *, #13703, .T. ) ;
#30385=CARTESIAN_POINT ( 'NONE',  ( -48.15927431543178727, 19.02058896284062683, -5.220430799464820915 ) ) ;
#30386=AXIS2_PLACEMENT_3D ( 'NONE', #4864, #18026, #11862 ) ;
#30392=ORIENTED_EDGE ( 'NONE', *, *, #40949, .F. ) ;
#30396=CARTESIAN_POINT ( 'NONE',  ( -46.91190649557855608, 20.26356613537080165, 4.963267847375941955 ) ) ;
#30402=AXIS2_PLACEMENT_3D ( 'NONE', #19590, #22989, #35597 ) ;
#30403=AXIS2_PLACEMENT_3D ( 'NONE', #9897, #39736, #23504 ) ;
#30407=DIRECTION ( 'NONE',  ( 0.7770581983690896255, -0.6294287539883961502, 3.619230632976993155E-16 ) ) ;
#30409=DIRECTION ( 'NONE',  ( -0.9816537812491090698, -0.1906721105965062946, 1.718035779124596298E-15 ) ) ;
#30411=CARTESIAN_POINT ( 'NONE',  ( -54.18067209322861544, 8.473630613757585195, 3.385134444937044407 ) ) ;
#30412=CARTESIAN_POINT ( 'NONE',  ( -29.05311006279642427, 61.33684941842457050, -1.524000000000005128 ) ) ;
#30413=CARTESIAN_POINT ( 'NONE',  ( -58.20820809768403592, 1.420579653404085985, 1.355822160094593443 ) ) ;
#30414=CARTESIAN_POINT ( 'NONE',  ( -57.74402180800798590, 1.613328144073144177, 1.607698224923606034 ) ) ;
#30417=AXIS2_PLACEMENT_3D ( 'NONE', #25403, #15587, #29001 ) ;
#30418=ORIENTED_EDGE ( 'NONE', *, *, #34464, .F. ) ;
#30419=FACE_OUTER_BOUND ( 'NONE', #2716, .T. ) ;
#30429=DIRECTION ( 'NONE',  ( -0.8745520943968235761, 0.4849315768086558398, -4.268512490100410909E-16 ) ) ;
#30430=CARTESIAN_POINT ( 'NONE',  ( -47.34495446287813536, 19.93462121982016200, 5.151308439916634008 ) ) ;
#30431=CARTESIAN_POINT ( 'NONE',  ( -30.09725872720941808, 70.36776381375389633, 1.269999999999992024 ) ) ;
#30433=FACE_OUTER_BOUND ( 'NONE', #17799, .T. ) ;
#30440=CIRCLE ( 'NONE', #8003, 0.5080000000000000071 ) ;
#30444=CARTESIAN_POINT ( 'NONE',  ( -47.93564525088164885, 15.36257551998183857, -7.016440965503648149E-15 ) ) ;
#30456=EDGE_LOOP ( 'NONE', ( #14587, #5245, #38780, #19672 ) ) ;
#30466=DIRECTION ( 'NONE',  ( -0.8745520943968249084, 0.4849315768086533418, -5.311926654347176508E-16 ) ) ;
#30470=EDGE_CURVE ( 'NONE', #1690, #13978, #34529, .T. ) ;
#30474=DIRECTION ( 'NONE',  ( -5.188838149069472160E-16, 1.699382548006136559E-16, 1.000000000000000000 ) ) ;
#30477=CYLINDRICAL_SURFACE ( 'NONE', #23745, 0.5080000000000007843 ) ;
#30483=CARTESIAN_POINT ( 'NONE',  ( -4.345705637489792217, 70.43763872253876457, -1.269999999999994023 ) ) ;
#30484=VERTEX_POINT ( 'NONE', #12767 ) ;
#30491=VERTEX_POINT ( 'NONE', #25966 ) ;
#30492=CYLINDRICAL_SURFACE ( 'NONE', #11002, 2.857500000000000817 ) ;
#30499=FACE_BOUND ( 'NONE', #17844, .T. ) ;
#30501=EDGE_CURVE ( 'NONE', #33914, #29626, #32160, .T. ) ;
#30503=EDGE_LOOP ( 'NONE', ( #14794, #8630, #38992, #16147 ) ) ;
#30507=CARTESIAN_POINT ( 'NONE',  ( -57.16742739522810979, 2.298121588018744887, 1.685181603002217310 ) ) ;
#30510=ADVANCED_FACE ( 'NONE', ( #16374 ), #2924, .T. ) ;
#30513=AXIS2_PLACEMENT_3D ( 'NONE', #13241, #13019, #26013 ) ;
#30516=CARTESIAN_POINT ( 'NONE',  ( -46.80150442283247259, 25.73581779614771747, 1.479909221305397704 ) ) ;
#30517=EDGE_CURVE ( 'NONE', #24344, #13695, #33544, .T. ) ;
#30518=CARTESIAN_POINT ( 'NONE',  ( -53.01551111795199489, 8.729259440421063942, -9.365303671399559428E-15 ) ) ;
#30521=CARTESIAN_POINT ( 'NONE',  ( -46.82521090855301082, 25.66317510763838072, -1.525079970390816664 ) ) ;
#30523=CARTESIAN_POINT ( 'NONE',  ( -31.81160528045694846, 53.04071001996608459, -1.269999999999624984 ) ) ;
#30528=CARTESIAN_POINT ( 'NONE',  ( -58.83227707057486811, -0.08366279997995551554, -1.527689555265638282E-14 ) ) ;
#30532=CARTESIAN_POINT ( 'NONE',  ( -58.13344828981739454, 1.721081384412917359, -0.8123818723938636133 ) ) ;
#30536=CARTESIAN_POINT ( 'NONE',  ( -46.48963984823998175, 20.58996865087576111, -4.821990630912100784 ) ) ;
#30545=CARTESIAN_POINT ( 'NONE',  ( -53.34828122837022590, 10.48226620245167773, -3.972818369368981806 ) ) ;
#30550=CARTESIAN_POINT ( 'NONE',  ( -57.55150406752473913, 1.473613606789017316, -1.350324376427143980 ) ) ;
#30554=CARTESIAN_POINT ( 'NONE',  ( -48.59875010875282442, 18.41211343146811785, -5.165832069028398088 ) ) ;
#30557=CARTESIAN_POINT ( 'NONE',  ( -28.42835727709238114, 77.69497285144578314, -1.270000000000007567 ) ) ;
#30558=ORIENTED_EDGE ( 'NONE', *, *, #26070, .T. ) ;
#30561=CYLINDRICAL_SURFACE ( 'NONE', #697, 0.2539999999999992819 ) ;
#30563=CARTESIAN_POINT ( 'NONE',  ( -51.09990735641632398, 14.52648110433587370, -4.713018929684125169 ) ) ;
#30566=CARTESIAN_POINT ( 'NONE',  ( -24.50334120614357403, 81.61487340491997600, 1.269999999999991802 ) ) ;
#30568=VECTOR ( 'NONE', #36465, 1000.000000000000000 ) ;
#30574=DIRECTION ( 'NONE',  ( 5.188838149069472160E-16, -1.699382548006136559E-16, -1.000000000000000000 ) ) ;
#30576=EDGE_CURVE ( 'NONE', #5052, #20172, #25757, .T. ) ;
#30577=CARTESIAN_POINT ( 'NONE',  ( -57.72731561024293967, 0.8685078910841970146, -1.031171003586682213E-14 ) ) ;
#30580=CARTESIAN_POINT ( 'NONE',  ( -47.06635113313992491, 25.00568333085942996, -1.230463370088899389 ) ) ;
#30582=CYLINDRICAL_SURFACE ( 'NONE', #22362, 2.857500000000000817 ) ;
#30583=ORIENTED_EDGE ( 'NONE', *, *, #26007, .F. ) ;
#30593=CARTESIAN_POINT ( 'NONE',  ( -47.61268981845987014, 19.67534100020180077, -5.209569013876577337 ) ) ;
#30596=ORIENTED_EDGE ( 'NONE', *, *, #2746, .F. ) ;
#30601=CARTESIAN_POINT ( 'NONE',  ( -58.71347258052157514, -0.3150591082025228085, -0.2754856216375807243 ) ) ;
#30605=ORIENTED_EDGE ( 'NONE', *, *, #33709, .F. ) ;
#30610=VERTEX_POINT ( 'NONE', #32366 ) ;
#30613=CARTESIAN_POINT ( 'NONE',  ( -30.03765869224011453, 57.96144573378211362, -1.270000000000005347 ) ) ;
#30621=CARTESIAN_POINT ( 'NONE',  ( -56.42582858034832327, 3.870711698533446210, 2.205403966022755124 ) ) ;
#30624=CARTESIAN_POINT ( 'NONE',  ( -58.23017998949752183, 0.6774554162835566551, 1.209604144815701554 ) ) ;
#30625=CARTESIAN_POINT ( 'NONE',  ( -58.64599579737798507, -0.3125068858902338431, 0.3366065011986605349 ) ) ;
#30629=CARTESIAN_POINT ( 'NONE',  ( -52.06546789126484498, 13.38259882428268632, 4.575081192416372566 ) ) ;
#30635=AXIS2_PLACEMENT_3D ( 'NONE', #18688, #25514, #12523 ) ;
#30637=VERTEX_POINT ( 'NONE', #6391 ) ;
#30641=CARTESIAN_POINT ( 'NONE',  ( -45.03191848990698531, 21.16108440570966209, 3.788620003472263242 ) ) ;
#30654=CARTESIAN_POINT ( 'NONE',  ( -49.53550897992070645, 16.97828837979668748, 4.976283659310158924 ) ) ;
#30658=ORIENTED_EDGE ( 'NONE', *, *, #13641, .T. ) ;
#30661=CARTESIAN_POINT ( 'NONE',  ( -13.15921246430372449, 51.38419125632634632, -1.269999999999995355 ) ) ;
#30663=ORIENTED_EDGE ( 'NONE', *, *, #33664, .F. ) ;
#30666=CARTESIAN_POINT ( 'NONE',  ( -6.650126595083637682, 78.47834120613788400, 1.270000000000001572 ) ) ;
#30667=AXIS2_PLACEMENT_3D ( 'NONE', #1649, #1851, #18012 ) ;
#30670=FACE_OUTER_BOUND ( 'NONE', #24991, .T. ) ;
#30671=AXIS2_PLACEMENT_3D ( 'NONE', #9967, #6572, #35334 ) ;
#30674=LINE ( 'NONE', #14478, #29356 ) ;
#30681=CARTESIAN_POINT ( 'NONE',  ( -17.14500000000466784, 71.11999999999886768, -1.270000000000000684 ) ) ;
#30689=ORIENTED_EDGE ( 'NONE', *, *, #22903, .F. ) ;
#30693=VECTOR ( 'NONE', #34882, 1000.000000000000114 ) ;
#30695=ORIENTED_EDGE ( 'NONE', *, *, #7627, .F. ) ;
#30696=ORIENTED_EDGE ( 'NONE', *, *, #35994, .T. ) ;
#30699=SURFACE_SIDE_STYLE ('',( #27518 ) ) ;
#30709=VERTEX_POINT ( 'NONE', #9782 ) ;
#30713=CARTESIAN_POINT ( 'NONE',  ( -57.21909960283011287, 2.250382150482001187, 1.879871960359134286 ) ) ;
#30719=CIRCLE ( 'NONE', #6267, 9.048749999999998295 ) ;
#30723=EDGE_CURVE ( 'NONE', #25607, #37389, #22750, .T. ) ;
#30725=CARTESIAN_POINT ( 'NONE',  ( -58.22824150656796860, 0.01698906185855497686, -0.5964212723216403278 ) ) ;
#30728=DIRECTION ( 'NONE',  ( 0.9816537812491077375, 0.1906721105965138996, 4.769617732184456426E-16 ) ) ;
#30730=DIRECTION ( 'NONE',  ( -5.188838149069471174E-16, 1.699382548006136313E-16, 1.000000000000000000 ) ) ;
#30734=CARTESIAN_POINT ( 'NONE',  ( -58.19197273006702886, 1.486408586729007109, 1.232490673556611016 ) ) ;
#30737=EDGE_LOOP ( 'NONE', ( #27202, #15763, #2173, #16579, #12161 ) ) ;
#30738=CARTESIAN_POINT ( 'NONE',  ( -56.10358335640970751, 6.949471795635917104, -1.762666882438596261 ) ) ;
#30747=CARTESIAN_POINT ( 'NONE',  ( -52.27215747984514138, 12.44583702737001829, -4.333897384857193558 ) ) ;
#30751=CARTESIAN_POINT ( 'NONE',  ( -51.93264227491449248, 12.78224484401628303, -4.246411715856839741 ) ) ;
#30754=CARTESIAN_POINT ( 'NONE',  ( -46.97515415817095175, 24.89137758704647396, -2.045406795549908896 ) ) ;
#30756=ADVANCED_FACE ( 'NONE', ( #23550 ), #1008, .T. ) ;
#30758=ORIENTED_EDGE ( 'NONE', *, *, #7844, .F. ) ;
#30762=CARTESIAN_POINT ( 'NONE',  ( -55.73247374733729487, 5.492406230130003841, -2.854677165782116610 ) ) ;
#30766=DIRECTION ( 'NONE',  ( -5.188838149069472160E-16, 1.699382548006136559E-16, 1.000000000000000000 ) ) ;
#30772=CARTESIAN_POINT ( 'NONE',  ( -58.83227707057486811, -0.08366279997995551554, -1.529465441686574059E-14 ) ) ;
#30773=CARTESIAN_POINT ( 'NONE',  ( -42.09164859969784089, 21.98995510696678934, -0.2271816505417319221 ) ) ;
#30776=CARTESIAN_POINT ( 'NONE',  ( -57.71946847630993460, 1.146847591362354368, 1.351507486235933975 ) ) ;
#30777=EDGE_CURVE ( 'NONE', #15033, #15131, #23288, .T. ) ;
#30779=VERTEX_POINT ( 'NONE', #3194 ) ;
#30780=CARTESIAN_POINT ( 'NONE',  ( -46.72476011081990066, 26.09744872113180847, -0.08471799968940613157 ) ) ;
#30782=DIRECTION ( 'NONE',  ( -0.8745520943968243532, 0.4849315768086547296, -6.829619984160642269E-16 ) ) ;
#30783=ORIENTED_EDGE ( 'NONE', *, *, #19947, .F. ) ;
#30794=CARTESIAN_POINT ( 'NONE',  ( -47.73411473560602047, 19.53609853455933631, -5.217284324479045665 ) ) ;
#30797=DIRECTION ( 'NONE',  ( 0.8572391118119521147, 0.5149185422762083686, 3.573031421855339458E-16 ) ) ;
#30802=CARTESIAN_POINT ( 'NONE',  ( -58.08606908514132527, 0.8771027734565672862, -1.270208019422474743 ) ) ;
#30808=VERTEX_POINT ( 'NONE', #15954 ) ;
#30810=EDGE_CURVE ( 'NONE', #12622, #27053, #31502, .T. ) ;
#30812=AXIS2_PLACEMENT_3D ( 'NONE', #34268, #1889, #34470 ) ;
#30814=AXIS2_PLACEMENT_3D ( 'NONE', #10426, #15963, #28961 ) ;
#30819=DIRECTION ( 'NONE',  ( 5.188838149069472160E-16, -1.699382548006136559E-16, -1.000000000000000000 ) ) ;
#30825=DIRECTION ( 'NONE',  ( 0.3582377630123915746, -0.9336303900108851028, 3.445432962228667069E-16 ) ) ;
#30827=CARTESIAN_POINT ( 'NONE',  ( -26.37263903973852663, 72.23735686029533554, -1.270000000000005791 ) ) ;
#30828=CARTESIAN_POINT ( 'NONE',  ( -56.16899616883418389, 4.407705243674411300, 2.360363118971548158 ) ) ;
#30830=CARTESIAN_POINT ( 'NONE',  ( -50.36571775388629391, 15.70662508241784927, 4.844678386991165375 ) ) ;
#30835=CARTESIAN_POINT ( 'NONE',  ( -55.03109054507046238, 6.816801101491506643, 3.135084751894912980 ) ) ;
#30838=AXIS2_PLACEMENT_3D ( 'NONE', #36785, #27185, #10575 ) ;
#30841=CARTESIAN_POINT ( 'NONE',  ( -29.78720458899295664, 57.91457584460150088, 1.523999999999994692 ) ) ;
#30843=EDGE_LOOP ( 'NONE', ( #9859, #12333, #38016, #13719 ) ) ;
#30846=CARTESIAN_POINT ( 'NONE',  ( -30.09725872720941808, 70.36776381375389633, -1.524000000000007349 ) ) ;
#30848=CARTESIAN_POINT ( 'NONE',  ( -47.35734194465046443, 19.95394279972230578, 5.176037500974643102 ) ) ;
#30861=EDGE_LOOP ( 'NONE', ( #27554, #24865, #33075, #40054 ) ) ;
#30862=CARTESIAN_POINT ( 'NONE',  ( -49.14072577824711630, 13.89916973120783972, -7.393049121003753577E-15 ) ) ;
#30866=CIRCLE ( 'NONE', #36340, 0.2540000000000013913 ) ;
#30867=ORIENTED_EDGE ( 'NONE', *, *, #19889, .F. ) ;
#30869=EDGE_CURVE ( 'NONE', #19961, #6241, #6323, .T. ) ;
#30874=ORIENTED_EDGE ( 'NONE', *, *, #1682, .T. ) ;
#30879=DIRECTION ( 'NONE',  ( -5.188838149069472160E-16, 1.699382548006136559E-16, 1.000000000000000000 ) ) ;
#30882=DIRECTION ( 'NONE',  ( -5.188838149069472160E-16, 1.699382548006136559E-16, 1.000000000000000000 ) ) ;
#30883=AXIS2_PLACEMENT_3D ( 'NONE', #14062, #7693, #40695 ) ;
#30885=LINE ( 'NONE', #41113, #27482 ) ;
#30888=VERTEX_POINT ( 'NONE', #26923 ) ;
#30889=VERTEX_POINT ( 'NONE', #7138 ) ;
#30890=DIRECTION ( 'NONE',  ( -0.8745520943968231320, 0.4849315768086568390, -5.691349986800559712E-16 ) ) ;
#30893=CIRCLE ( 'NONE', #36364, 0.3809999999999984510 ) ;
#30898=CARTESIAN_POINT ( 'NONE',  ( -48.28978369826177186, 19.63653578263565436, 5.206999999995388428 ) ) ;
#30901=B_SPLINE_CURVE_WITH_KNOTS ( 'NONE', 3,
 ( #21866, #34892, #5723, #14643, #25291, #38295, #9115, #22077, #35104, #17842, #30841, #25707, #19098, #171, #26133, #23121 ),
 .UNSPECIFIED., .F., .F.,
 ( 4, 2, 2, 2, 2, 2, 2, 4 ),
 ( 0.000000000000000000, 0.005276917911546602849, 0.006596147389433264403, 0.007915376867319925958, 0.01055383582309329070, 0.01319229477886665544, 0.01583075373464001845, 0.02110767164618673059 ),
 .UNSPECIFIED. ) ;
#30906=ORIENTED_EDGE ( 'NONE', *, *, #27686, .T. ) ;
#30919=ADVANCED_FACE ( 'NONE', ( #39725 ), #10524, .F. ) ;
#30923=ADVANCED_FACE ( 'NONE', ( #36106 ), #30124, .T. ) ;
#30930=CARTESIAN_POINT ( 'NONE',  ( -58.52535285190437975, -0.5719483744759017441, 0.2498204902891903723 ) ) ;
#30938=CARTESIAN_POINT ( 'NONE',  ( -57.34787435976332404, 1.552391619547691004, -1.028525222821079960E-14 ) ) ;
#30943=FACE_OUTER_BOUND ( 'NONE', #41220, .T. ) ;
#30951=FACE_OUTER_BOUND ( 'NONE', #13344, .T. ) ;
#30953=CARTESIAN_POINT ( 'NONE',  ( -46.93088534759994701, 20.29541677029510893, -5.030633991645946601 ) ) ;
#30960=CARTESIAN_POINT ( 'NONE',  ( -50.97644874786027458, 14.69290941399900596, -4.697037614708189146 ) ) ;
#30961=ORIENTED_EDGE ( 'NONE', *, *, #13127, .F. ) ;
#30962=CARTESIAN_POINT ( 'NONE',  ( -29.81357423954495189, 70.62209452652477637, -1.524000000000007349 ) ) ;
#30963=CARTESIAN_POINT ( 'NONE',  ( -30.09725872720941453, 70.36776381375388212, 1.523999999999992250 ) ) ;
#30965=CARTESIAN_POINT ( 'NONE',  ( -56.32662672728373821, 4.077578507741069558, -2.263812825962038033 ) ) ;
#30968=CARTESIAN_POINT ( 'NONE',  ( -43.83556092231052048, 21.45200552150719631, -2.811646013901254015 ) ) ;
#30975=CARTESIAN_POINT ( 'NONE',  ( -57.09878488423309051, 3.216020309495956742, -2.217633722229552351 ) ) ;
#30981=CARTESIAN_POINT ( 'NONE',  ( -57.66338803320029882, 2.692357263605615891, -1.869785753600856637 ) ) ;
#30982=CARTESIAN_POINT ( 'NONE',  ( -33.42971872652992005, 49.93539301574497102, -1.524000000000005572 ) ) ;
#30983=ORIENTED_EDGE ( 'NONE', *, *, #17004, .F. ) ;
#30985=DIRECTION ( 'NONE',  ( 0.8745520943968235761, -0.4849315768086558398, 4.268512490100410909E-16 ) ) ;
#30986=CARTESIAN_POINT ( 'NONE',  ( -57.55293229875817218, 1.419684655164468623, 1.132508401016375288 ) ) ;
#30987=CARTESIAN_POINT ( 'NONE',  ( -50.36444701916330047, 17.30043933429478642, 4.508886934713581596 ) ) ;
#30989=AXIS2_PLACEMENT_3D ( 'NONE', #1228, #20570, #33178 ) ;
#30990=ORIENTED_EDGE ( 'NONE', *, *, #1565, .F. ) ;
#30991=CARTESIAN_POINT ( 'NONE',  ( -48.77319768356018415, 22.00425556813275563, -2.071420771163298813 ) ) ;
#30998=DIRECTION ( 'NONE',  ( -0.9876665170007974393, 0.1565721916417901483, -8.537024980200831679E-16 ) ) ;
#31004=EDGE_CURVE ( 'NONE', #21597, #35463, #17859, .T. ) ;
#31009=DIRECTION ( 'NONE',  ( 0.01876124593811915112, 0.9998239923360757730, 0.000000000000000000 ) ) ;
#31011=CARTESIAN_POINT ( 'NONE',  ( -58.33068375617585133, -0.2093732065605730108, -0.2478323015014812503 ) ) ;
#31024=ADVANCED_FACE ( 'NONE', ( #7550 ), #11753, .T. ) ;
#31025=AXIS2_PLACEMENT_3D ( 'NONE', #38443, #12858, #35043 ) ;
#31037=CARTESIAN_POINT ( 'NONE',  ( -58.36850749721234877, -0.2888827900911983271, 0.04284473868145901448 ) ) ;
#31039=CARTESIAN_POINT ( 'NONE',  ( -49.76517000418316172, 16.66822512019472313, 4.974244438740138108 ) ) ;
#31045=CARTESIAN_POINT ( 'NONE',  ( -50.11792632901008915, 17.09067799859288783, 5.048577231237564966 ) ) ;
#31052=ADVANCED_FACE ( 'NONE', ( #3737 ), #16695, .T. ) ;
#31058=CIRCLE ( 'NONE', #36516, 0.3809999999999984510 ) ;
#31063=CARTESIAN_POINT ( 'NONE',  ( -29.82321757229076908, 71.17901112636586447, -1.270000000000007123 ) ) ;
#31070=VERTEX_POINT ( 'NONE', #26286 ) ;
#31071=CARTESIAN_POINT ( 'NONE',  ( -52.94148447887670272, 9.133269539094115430, 0.6394659809470414347 ) ) ;
#31086=CARTESIAN_POINT ( 'NONE',  ( -4.476425760464393555, 71.61790547347303004, -1.523999999999994248 ) ) ;
#31091=DIRECTION ( 'NONE',  ( -5.188838149069472160E-16, 1.699382548006136559E-16, 1.000000000000000000 ) ) ;
#31093=CARTESIAN_POINT ( 'NONE',  ( -45.67973391888839529, 25.66060799623228661, 1.523999999999991806 ) ) ;
#31097=ORIENTED_EDGE ( 'NONE', *, *, #102, .T. ) ;
#31098=CARTESIAN_POINT ( 'NONE',  ( -16.02764313970816090, 80.34763903973272647, 1.523999999999997579 ) ) ;
#31105=CIRCLE ( 'NONE', #36565, 0.6350000000000014522 ) ;
#31108=CARTESIAN_POINT ( 'NONE',  ( -56.90590057130552282, 4.418898835881354792, 2.427662546266514454 ) ) ;
#31115=ORIENTED_EDGE ( 'NONE', *, *, #4066, .F. ) ;
#31122=ORIENTED_EDGE ( 'NONE', *, *, #33425, .F. ) ;
#31123=PLANE ( 'NONE',  #27621 ) ;
#31124=CIRCLE ( 'NONE', #12663, 0.2540000000000004476 ) ;
#31127=CARTESIAN_POINT ( 'NONE',  ( -25.81615557310160369, 74.46796499802707103, 1.523999999999993582 ) ) ;
#31134=ORIENTED_EDGE ( 'NONE', *, *, #10952, .F. ) ;
#31137=AXIS2_PLACEMENT_3D ( 'NONE', #5421, #28191, #31811 ) ;
#31138=CARTESIAN_POINT ( 'NONE',  ( -58.39415239746359276, -0.3126312442514861401, 0.4522786855634189918 ) ) ;
#31146=CARTESIAN_POINT ( 'NONE',  ( -57.99953387342350908, 0.4830015814202143209, -0.7353922615980251765 ) ) ;
#31149=CARTESIAN_POINT ( 'NONE',  ( -43.82859865241511699, 24.63416949198730421, -1.524000000000006905 ) ) ;
#31150=CARTESIAN_POINT ( 'NONE',  ( -5.591489108514605455, 77.73497692594764885, 1.270000000000002238 ) ) ;
#31152=ADVANCED_FACE ( 'NONE', ( #20935 ), #37555, .T. ) ;
#31155=DIRECTION ( 'NONE',  ( -0.8745520943968250194, 0.4849315768086532863, -5.361993529360574930E-16 ) ) ;
#31158=EDGE_LOOP ( 'NONE', ( #38822, #34002, #30783, #39670 ) ) ;
#31159=CARTESIAN_POINT ( 'NONE',  ( -58.16194989728257525, 1.772972946764567181, -0.08436090182518581060 ) ) ;
#31160=ORIENTED_EDGE ( 'NONE', *, *, #5289, .T. ) ;
#31161=CARTESIAN_POINT ( 'NONE',  ( -46.39387867998599546, 20.78226312412258991, -4.747706454273081356 ) ) ;
#31168=CARTESIAN_POINT ( 'NONE',  ( -50.20358007252900734, 15.96865141398877697, -4.880505329357888833 ) ) ;
#31169=EDGE_LOOP ( 'NONE', ( #13369, #29191, #3423, #22874 ) ) ;
#31173=CARTESIAN_POINT ( 'NONE',  ( -53.66578727863507225, 9.481950398213415454, -3.598112444201927662 ) ) ;
#31176=CARTESIAN_POINT ( 'NONE',  ( -50.11792632901008915, 17.09067799859288783, -5.048577231237582730 ) ) ;
#31182=CARTESIAN_POINT ( 'NONE',  ( -58.33777482027510786, 1.113448835244251756, -1.208045587469442017 ) ) ;
#31190=CARTESIAN_POINT ( 'NONE',  ( -44.27221412529542022, 20.06621383160478445, -0.8981538560692819972 ) ) ;
#31194=CARTESIAN_POINT ( 'NONE',  ( -58.18636467486479091, 0.07352994790495170907, 0.3924542439260513826 ) ) ;
#31195=CARTESIAN_POINT ( 'NONE',  ( -50.72152632752359125, 17.59631655692102470, 3.767527310968340704 ) ) ;
#31198=CARTESIAN_POINT ( 'NONE',  ( -50.10414895690885828, 20.83497401302349061, -1.621381026025509708 ) ) ;
#31201=EDGE_LOOP ( 'NONE', ( #3919, #6523, #30375, #16033 ) ) ;
#31212=CARTESIAN_POINT ( 'NONE',  ( -46.44929266343369534, 20.74717589152057329, -4.783910049210099658 ) ) ;
#31213=FACE_OUTER_BOUND ( 'NONE', #9957, .T. ) ;
#31214=ORIENTED_EDGE ( 'NONE', *, *, #36060, .F. ) ;
#31216=DIRECTION ( 'NONE',  ( -0.8745520943968245753, 0.4849315768086539524, -5.691349986800526185E-16 ) ) ;
#31218=CARTESIAN_POINT ( 'NONE',  ( -48.15691857873192561, 19.01861963077412199, -5.213839621096282961 ) ) ;
#31242=CARTESIAN_POINT ( 'NONE',  ( -58.36779176277465808, -0.2873857612693362373, 0.05403644662055718390 ) ) ;
#31243=DIRECTION ( 'NONE',  ( -5.188838149069471174E-16, 1.699382548006136313E-16, 1.000000000000000000 ) ) ;
#31244=ADVANCED_FACE ( 'NONE', ( #18158 ), #36502, .T. ) ;
#31245=EDGE_CURVE ( 'NONE', #26949, #19837, #21255, .T. ) ;
#31246=DIRECTION ( 'NONE',  ( -5.188838149069471174E-16, 1.699382548006136313E-16, 1.000000000000000000 ) ) ;
#31247=AXIS2_PLACEMENT_3D ( 'NONE', #33354, #1195, #10756 ) ;
#31250=ORIENTED_EDGE ( 'NONE', *, *, #261, .T. ) ;
#31251=CARTESIAN_POINT ( 'NONE',  ( -51.54051843738712080, 14.84038450301108192, 4.692172599169413871 ) ) ;
#31261=DIRECTION ( 'NONE',  ( 5.188838149069472160E-16, -1.699382548006136559E-16, -1.000000000000000000 ) ) ;
#31262=CARTESIAN_POINT ( 'NONE',  ( -25.56614996202194590, 73.65611136973726047, 1.269999999999993578 ) ) ;
#31263=CARTESIAN_POINT ( 'NONE',  ( -41.52577271625691679, 22.97115911878592343, 1.523999999999989807 ) ) ;
#31264=FACE_OUTER_BOUND ( 'NONE', #6259, .T. ) ;
#31276=CARTESIAN_POINT ( 'NONE',  ( -57.41561397472474937, 1.705883423724310788, 1.231064337386900354 ) ) ;
#31280=ORIENTED_EDGE ( 'NONE', *, *, #7178, .T. ) ;
#31287=ORIENTED_EDGE ( 'NONE', *, *, #5270, .F. ) ;
#31290=CARTESIAN_POINT ( 'NONE',  ( -23.75997692595333177, 82.67351089148900201, 1.269999999999992912 ) ) ;
#31291=DIRECTION ( 'NONE',  ( -0.8745520943968235761, 0.4849315768086558398, -5.691349986800547879E-16 ) ) ;
#31296=CARTESIAN_POINT ( 'NONE',  ( -11.53797084252497207, 82.58007221317646440, -1.524000000000000021 ) ) ;
#31298=B_SPLINE_SURFACE_WITH_KNOTS ( 'NONE', 3, 3, ( 
 ( #31456, #2300, #18666, #40848, #28048 ),
 ( #2513, #41057, #11867, #15477, #24856 ),
 ( #39956, #33346, #20744, #27568, #37366 ),
 ( #8185, #1605, #4176, #20319, #1393 ),
 ( #14563, #14349, #17754, #33560, #30754 ),
 ( #17139, #36961, #4803, #13946, #23515 ),
 ( #36749, #30140, #40577, #1186, #24152 ),
 ( #30968, #981, #20531, #26944, #4594 ),
 ( #34183, #10749, #33975, #39748, #23730 ),
 ( #17350, #7570, #10956, #21153, #37161 ),
 ( #11168, #27360, #36543, #14148, #14770 ),
 ( #4394, #40163, #30338, #27151, #40372 ),
 ( #23943, #11374, #24361, #7783, #33769 ),
 ( #17553, #7361, #5009, #17970, #1809 ),
 ( #30554, #7982, #10546, #20951, #19017 ),
 ( #15406, #2017, #41416, #24998, #21782 ),
 ( #21998, #12222, #31390, #31176, #8607 ),
 ( #25428, #15612, #28196, #41202, #34597 ),
 ( #35230, #38429, #27982, #27772, #5850 ),
 ( #24784, #12006, #22201, #14981, #9243 ),
 ( #11581, #5426, #28617, #37782, #40783 ),
 ( #31607, #6057, #31816, #2445, #18805 ),
 ( #2654, #24566, #21359, #37998, #35030 ),
 ( #37570, #21569, #18382, #34385, #5219 ),
 ( #38217, #18173, #2233, #41628, #2861 ),
 ( #32023, #15193, #12435, #8397, #8822 ),
 ( #34808, #5641, #40990, #28410, #18599 ),
 ( #25214, #11793, #9033, #12639, #6675 ),
 ( #19437, #16235, #41843, #25626, #13267 ),
 ( #3701, #7102, #39049, #509, #32443 ),
 ( #29239, #13482, #26251, #294, #29455 ),
 ( #39261, #10278, #36070, #10067, #29028 ),
 ( #3070, #35434, #32655, #6258, #16028 ),
 ( #23039, #42047, #12844, #38636, #38839 ),
 ( #6886, #39473, #32869, #16661, #25829 ),
 ( #28829, #9855, #20063, #9648, #3491 ),
 ( #19855, #13049, #22825, #29668, #22615 ),
 ( #26470, #35862, #19641, #35649, #16449 ),
 ( #6463, #23248, #9441, #26040, #32238 ) ),
 .UNSPECIFIED., .F., .F., .F.,
 ( 4, 1, 1, 1, 1, 1, 1, 1, 1, 1, 1, 2, 1, 1, 1, 1, 1, 1, 1, 1, 1, 1, 1, 1, 1, 1, 1, 1, 1, 1, 1, 1, 1, 1, 1, 4 ),
 ( 4, 1, 4 ),
 ( 0.000000000000000000, 0.01653533301974152367, 0.03307066603948304734, 0.04960599905922460223, 0.06614133207896609468, 0.08267666509870763569, 0.09921199811844919059, 0.1322826641579321894, 0.1653533301974152714, 0.1984239962368983812, 0.2314946622763813522, 0.2645653283158643787, 0.3105299952961229071, 0.3335123287862520880, 0.3564946622763812689, 0.4024593292566397418, 0.4484239962368982702, 0.4943886632171566875, 0.5403533301974150493, 0.5863179971776735222, 0.6322826641579321061, 0.6782473311381906900, 0.7242119981184491628, 0.7701766650987074136, 0.8161413320789658865, 0.8621059990592241373, 0.8735971658042887000, 0.8850883325493537068, 0.8965794992944182695, 0.9080706660394826102, 0.9195618327845473949, 0.9310529995296121797, 0.9425441662746769644, 0.9540353330197415271, 0.9770176665098706525, 1.000000000000000000 ),
 ( 0.000000000000000000, 0.5000000000000000000, 1.000000000000000000 ),
 .UNSPECIFIED. ) ;
#31300=VERTEX_POINT ( 'NONE', #28180 ) ;
#31304=AXIS2_PLACEMENT_3D ( 'NONE', #37478, #27481, #11487 ) ;
#31309=CARTESIAN_POINT ( 'NONE',  ( -17.09698261757901960, 84.43312239790384410, 1.269999999999995355 ) ) ;
#31314=EDGE_CURVE ( 'NONE', #27648, #35654, #21919, .T. ) ;
#31315=DIRECTION ( 'NONE',  ( -0.9998501190848636533, -0.01731298258487590572, 2.898946086000287674E-15 ) ) ;
#31316=DIRECTION ( 'NONE',  ( 5.188838149069472160E-16, -1.699382548006136559E-16, -1.000000000000000000 ) ) ;
#31317=CARTESIAN_POINT ( 'NONE',  ( -48.28978369826177186, 19.63653578263564015, -5.206999999995405304 ) ) ;
#31342=ORIENTED_EDGE ( 'NONE', *, *, #27207, .T. ) ;
#31345=EDGE_CURVE ( 'NONE', #25690, #500, #22616, .T. ) ;
#31346=VECTOR ( 'NONE', #13005, 1000.000000000000000 ) ;
#31347=DIRECTION ( 'NONE',  ( -0.9876665170007974393, 0.1565721916417901483, -8.537024980200831679E-16 ) ) ;
#31348=EDGE_CURVE ( 'NONE', #2461, #40395, #41185, .T. ) ;
#31349=CARTESIAN_POINT ( 'NONE',  ( -49.26674734213751350, 17.44270459986665145, 5.073646373251102126 ) ) ;
#31358=CARTESIAN_POINT ( 'NONE',  ( -57.70855261479918141, 1.142328357490882240, -1.228565355106010504 ) ) ;
#31361=CARTESIAN_POINT ( 'NONE',  ( -6.096037513970403054, 78.08166987308820239, -1.523999999999996247 ) ) ;
#31365=PLANE ( 'NONE',  #38914 ) ;
#31370=CARTESIAN_POINT ( 'NONE',  ( -58.82374062945601167, -0.06097470622967726683, -0.2234658159562166180 ) ) ;
#31372=CARTESIAN_POINT ( 'NONE',  ( -16.71197878298170991, 83.87086364642222236, -1.270000000000002682 ) ) ;
#31381=CARTESIAN_POINT ( 'NONE',  ( -50.27159791831159197, 15.85842796992063164, -4.865305682342245142 ) ) ;
#31382=ADVANCED_FACE ( 'NONE', ( #35215 ), #36946, .T. ) ;
#31383=ORIENTED_EDGE ( 'NONE', *, *, #31589, .F. ) ;
#31387=CARTESIAN_POINT ( 'NONE',  ( -49.16865371179721933, 17.52875052363311070, -5.029076361559855712 ) ) ;
#31390=CARTESIAN_POINT ( 'NONE',  ( -49.93490050754573417, 16.96705409125581099, -5.170188367178254474 ) ) ;
#31398=EDGE_CURVE ( 'NONE', #34293, #2670, #5664, .T. ) ;
#31399=CARTESIAN_POINT ( 'NONE',  ( -57.67794393518098417, 1.927849678527493449, -1.763631237166056520 ) ) ;
#31404=CIRCLE ( 'NONE', #13036, 0.2540000000000000036 ) ;
#31408=CARTESIAN_POINT ( 'NONE',  ( -23.24761240069422286, 77.83567810938664877, -1.270000000000005125 ) ) ;
#31410=CARTESIAN_POINT ( 'NONE',  ( -57.43854689232674815, 1.757847328446624058, 1.624773336220232789 ) ) ;
#31411=PLANE ( 'NONE',  #40627 ) ;
#31413=CARTESIAN_POINT ( 'NONE',  ( -48.88162864671050301, 20.15829640254822408, 3.957548906738488803 ) ) ;
#31416=CARTESIAN_POINT ( 'NONE',  ( -48.20156657701303970, 19.76063879377972654, -5.201425424509408479 ) ) ;
#31418=DIRECTION ( 'NONE',  ( 5.188838149069472160E-16, -1.699382548006136559E-16, -1.000000000000000000 ) ) ;
#31419=EDGE_LOOP ( 'NONE', ( #10145, #34590, #30293, #3492 ) ) ;
#31431=CARTESIAN_POINT ( 'NONE',  ( -42.38674010915296009, 22.29968555344163761, -1.779698089469653466 ) ) ;
#31450=CARTESIAN_POINT ( 'NONE',  ( -17.14500000000466784, 71.11999999999886768, 1.523999999999998689 ) ) ;
#31452=AXIS2_PLACEMENT_3D ( 'NONE', #31372, #21765, #16013 ) ;
#31456=CARTESIAN_POINT ( 'NONE',  ( -41.05189575270516400, 23.09451173561986081, -1.524000000000003130 ) ) ;
#31459=CARTESIAN_POINT ( 'NONE',  ( -58.05678064718770770, 0.3813734126662043922, 0.7812039021332745081 ) ) ;
#31463=CIRCLE ( 'NONE', #32823, 0.6349999999999969003 ) ;
#31466=CARTESIAN_POINT ( 'NONE',  ( -52.30895062419047292, 13.66434875625866674, 4.401212925246481333 ) ) ;
#31472=ORIENTED_EDGE ( 'NONE', *, *, #21654, .F. ) ;
#31474=CARTESIAN_POINT ( 'NONE',  ( -29.04966993605376047, 66.62533279659477614, 1.523999999999992916 ) ) ;
#31475=DIRECTION ( 'NONE',  ( 5.188838149069472160E-16, -1.699382548006136559E-16, -1.000000000000000000 ) ) ;
#31487=CIRCLE ( 'NONE', #2955, 0.7619999999999983453 ) ;
#31490=CARTESIAN_POINT ( 'NONE',  ( -55.81215269371604393, 4.390389611868092068, 0.4227292597524335283 ) ) ;
#31502=B_SPLINE_CURVE_WITH_KNOTS ( 'NONE', 3,
 ( #29161, #7, #34413, #8635 ),
 .UNSPECIFIED., .F., .F.,
 ( 4, 4 ),
 ( 0.000000000000000000, 1.000000000000000000 ),
 .UNSPECIFIED. ) ;
#31503=DIRECTION ( 'NONE',  ( -0.8745520943968251304, 0.4849315768086532863, -5.424246918827961050E-16 ) ) ;
#31509=DIRECTION ( 'NONE',  ( -0.8745520943968225769, 0.4849315768086578382, -5.691349986800571545E-16 ) ) ;
#31511=TOROIDAL_SURFACE ( 'NONE', #24034, 0.7620000000000000107, 0.2540000000000000036 ) ;
#31513=ORIENTED_EDGE ( 'NONE', *, *, #24554, .F. ) ;
#31514=ORIENTED_EDGE ( 'NONE', *, *, #10507, .F. ) ;
#31515=DIRECTION ( 'NONE',  ( -0.7548010569845121642, -0.6559537821943426383, 0.000000000000000000 ) ) ;
#31524=CARTESIAN_POINT ( 'NONE',  ( -5.639506490940112471, 64.42185452804264401, -1.269999999999993578 ) ) ;
#31530=DIRECTION ( 'NONE',  ( -0.1565721916417989190, -0.9876665170007961070, 6.504343050004413423E-15 ) ) ;
#31542=DIRECTION ( 'NONE',  ( 5.188838149069472160E-16, -1.699382548006136559E-16, -1.000000000000000000 ) ) ;
#31548=VECTOR ( 'NONE', #32481, 1000.000000000000000 ) ;
#31551=EDGE_CURVE ( 'NONE', #12215, #21468, #925, .T. ) ;
#31557=DIRECTION ( 'NONE',  ( 5.188838149069472160E-16, -1.699382548006136559E-16, -1.000000000000000000 ) ) ;
#31558=DIRECTION ( 'NONE',  ( -5.188838149069472160E-16, 1.699382548006136559E-16, 1.000000000000000000 ) ) ;
#31560=CIRCLE ( 'NONE', #16588, 0.2540000000000002811 ) ;
#31561=CARTESIAN_POINT ( 'NONE',  ( -57.20860189792659156, 2.757428422320171268, 2.041684569450760822 ) ) ;
#31562=EDGE_CURVE ( 'NONE', #10068, #38754, #19840, .T. ) ;
#31568=AXIS2_PLACEMENT_3D ( 'NONE', #3295, #22845, #3724 ) ;
#31574=CARTESIAN_POINT ( 'NONE',  ( -57.72731561024291125, 0.8685078910842247701, -0.07340608407947644964 ) ) ;
#31578=LINE ( 'NONE', #37543, #40972 ) ;
#31582=CARTESIAN_POINT ( 'NONE',  ( -15.74027684387364978, 85.27021604205610572, -1.270000000000002460 ) ) ;
#31588=CARTESIAN_POINT ( 'NONE',  ( -58.49256177947683000, 0.7572623586737103896, -0.8868308481464118875 ) ) ;
#31589=EDGE_CURVE ( 'NONE', #2780, #18488, #15844, .T. ) ;
#31591=CARTESIAN_POINT ( 'NONE',  ( -41.35912177800447154, 22.76994845978005344, -1.271081184882984383 ) ) ;
#31599=CARTESIAN_POINT ( 'NONE',  ( -58.51381316099766394, -0.04972149827416968287, -0.6596742545330949170 ) ) ;
#31602=DIRECTION ( 'NONE',  ( 5.188838149069472160E-16, -1.699382548006136559E-16, -1.000000000000000000 ) ) ;
#31604=CARTESIAN_POINT ( 'NONE',  ( -55.48157428470955921, 5.837899645253390446, -2.755819015989877663 ) ) ;
#31607=CARTESIAN_POINT ( 'NONE',  ( -53.09398923718962493, 10.65108322687173548, -3.938325876039776574 ) ) ;
#31609=VERTEX_POINT ( 'NONE', #23024 ) ;
#31613=CARTESIAN_POINT ( 'NONE',  ( -58.43690671596436914, -0.4125963578781866037, -1.035377653829272970E-14 ) ) ;
#31616=CARTESIAN_POINT ( 'NONE',  ( -30.09725872720941453, 70.36776381375388212, -1.270000000000007123 ) ) ;
#31619=LINE ( 'NONE', #12020, #22159 ) ;
#31622=VERTEX_POINT ( 'NONE', #32854 ) ;
#31625=CARTESIAN_POINT ( 'NONE',  ( -57.36719850051837000, 1.975114663830185302, 1.756955940785651871 ) ) ;
#31627=CARTESIAN_POINT ( 'NONE',  ( -58.37241122568488549, -0.2962816677227753104, -1.039428729632917149E-14 ) ) ;
#31628=CARTESIAN_POINT ( 'NONE',  ( -52.06588384954375925, 19.72955628912294301, 0.3571238398875058451 ) ) ;
#31630=ORIENTED_EDGE ( 'NONE', *, *, #7183, .F. ) ;
#31631=CARTESIAN_POINT ( 'NONE',  ( -49.01671973967525275, 18.67808020721671625, -5.174630477995055600 ) ) ;
#31633=CARTESIAN_POINT ( 'NONE',  ( -5.639506490940112471, 64.42185452804264401, -1.523999999999993582 ) ) ;
#31643=DIRECTION ( 'NONE',  ( -0.9336303900108928744, -0.3582377630123714241, 0.000000000000000000 ) ) ;
#31646=DIRECTION ( 'NONE',  ( -0.8745520943968246863, 0.4849315768086537859, -5.361993529360573944E-16 ) ) ;
#31648=ORIENTED_EDGE ( 'NONE', *, *, #28983, .F. ) ;
#31673=CIRCLE ( 'NONE', #6506, 0.5079999999999993410 ) ;
#31676=CARTESIAN_POINT ( 'NONE',  ( -58.15532689777176500, 0.1682042465437465772, 0.6324092216884573681 ) ) ;
#31681=CARTESIAN_POINT ( 'NONE',  ( -57.24023649071029496, 3.661034843983918208, 2.195083147259549339 ) ) ;
#31687=EDGE_CURVE ( 'NONE', #35981, #22227, #18555, .T. ) ;
#31690=CARTESIAN_POINT ( 'NONE',  ( -29.47815206463771887, 60.51098513943350810, 1.523999999999992916 ) ) ;
#31691=CARTESIAN_POINT ( 'NONE',  ( -6.194847070882102180, 64.72978607931611350, -1.269999999999994023 ) ) ;
#31692=CARTESIAN_POINT ( 'NONE',  ( -41.35912177800472023, 22.76994845977980120, 1.271081184897154825 ) ) ;
#31695=ADVANCED_FACE ( 'NONE', ( #32639 ), #10891, .T. ) ;
#31706=CARTESIAN_POINT ( 'NONE',  ( -54.16862281694330505, 7.200593192618495841, 0.5614961770967360488 ) ) ;
#31707=AXIS2_PLACEMENT_3D ( 'NONE', #18833, #12243, #2254 ) ;
#31715=ORIENTED_EDGE ( 'NONE', *, *, #20329, .T. ) ;
#31717=LINE ( 'NONE', #21474, #36752 ) ;
#31718=CARTESIAN_POINT ( 'NONE',  ( -6.422645615570758970, 77.88548590848095898, 1.270000000000002682 ) ) ;
#31723=CARTESIAN_POINT ( 'NONE',  ( -47.15184857521119710, 25.06101562935922900, 0.8929867115423234525 ) ) ;
#31725=CARTESIAN_POINT ( 'NONE',  ( -45.45367893016184979, 22.54667639846615046, 3.012003376585078662 ) ) ;
#31729=CIRCLE ( 'NONE', #22854, 0.3810000000000007825 ) ;
#31742=ADVANCED_FACE ( 'NONE', ( #23663 ), #7694, .T. ) ;
#31753=AXIS2_PLACEMENT_3D ( 'NONE', #29186, #32600, #16615 ) ;
#31755=EDGE_LOOP ( 'NONE', ( #7476, #3213, #33969, #32178 ) ) ;
#31756=ORIENTED_EDGE ( 'NONE', *, *, #13641, .F. ) ;
#31763=CIRCLE ( 'NONE', #13385, 8.794749999999998735 ) ;
#31769=TOROIDAL_SURFACE ( 'NONE', #14752, 0.7620000000000000107, 0.2540000000000000036 ) ;
#31773=CARTESIAN_POINT ( 'NONE',  ( -18.58115504727956591, 80.30342350548193053, -1.270000000000003126 ) ) ;
#31774=CARTESIAN_POINT ( 'NONE',  ( -58.63158931450232814, -0.2944865825853931751, 0.3706283016935131847 ) ) ;
#31781=VECTOR ( 'NONE', #20310, 1000.000000000000114 ) ;
#31786=CIRCLE ( 'NONE', #18857, 0.2539999999999998925 ) ;
#31792=FACE_OUTER_BOUND ( 'NONE', #38573, .T. ) ;
#31794=EDGE_CURVE ( 'NONE', #6455, #27023, #3204, .T. ) ;
#31797=AXIS2_PLACEMENT_3D ( 'NONE', #4523, #40093, #23231 ) ;
#31799=CARTESIAN_POINT ( 'NONE',  ( -58.83227707057489653, -0.08366279998001102669, -5.813756590757272400E-15 ) ) ;
#31800=ORIENTED_EDGE ( 'NONE', *, *, #37837, .F. ) ;
#31801=CARTESIAN_POINT ( 'NONE',  ( -42.73979388487836673, 22.09733806376468124, -1.954747716862336171 ) ) ;
#31807=CARTESIAN_POINT ( 'NONE',  ( -58.11310633828895789, 0.8178190558498232843, -1.239050447815041922 ) ) ;
#31808=EDGE_CURVE ( 'NONE', #28149, #514, #25766, .T. ) ;
#31811=DIRECTION ( 'NONE',  ( -0.8745520943968249084, 0.4849315768086533418, -5.271987356194193006E-16 ) ) ;
#31816=CARTESIAN_POINT ( 'NONE',  ( -53.45432727069204759, 10.77832982246877691, -4.078803160923793136 ) ) ;
#31823=CARTESIAN_POINT ( 'NONE',  ( -47.84756666395259117, 19.38928433903615911, -5.209054514891951371 ) ) ;
#31826=CARTESIAN_POINT ( 'NONE',  ( -41.09670346151922615, 23.04688172092959775, 1.270085369932517194 ) ) ;
#31830=CARTESIAN_POINT ( 'NONE',  ( -48.56815661899837977, 19.24492339269602681, -5.224590812749990931 ) ) ;
#31831=CARTESIAN_POINT ( 'NONE',  ( -46.67338572489352089, 16.85372243840493311, -0.3683569569372189823 ) ) ;
#31833=LINE ( 'NONE', #9261, #14861 ) ;
#31834=CARTESIAN_POINT ( 'NONE',  ( -57.52317756609133426, 3.014644041894651405, 1.981665235817938076 ) ) ;
#31835=CARTESIAN_POINT ( 'NONE',  ( -56.55101830787051398, 4.138461899075373651, 2.474321349783852764 ) ) ;
#31836=FACE_OUTER_BOUND ( 'NONE', #16391, .T. ) ;
#31838=CARTESIAN_POINT ( 'NONE',  ( -53.04800011021367112, 17.61732480354184815, -1.032319417969101073E-14 ) ) ;
#31840=VERTEX_POINT ( 'NONE', #16384 ) ;
#31841=CARTESIAN_POINT ( 'NONE',  ( -49.15418877470109749, 24.05022684412165646, -0.2550087576077226803 ) ) ;
#31856=EDGE_CURVE ( 'NONE', #18068, #32282, #23323, .T. ) ;
#31857=CYLINDRICAL_SURFACE ( 'NONE', #39457, 0.2540000000000023350 ) ;
#31858=VERTEX_POINT ( 'NONE', #7035 ) ;
#31860=CARTESIAN_POINT ( 'NONE',  ( -58.36637034709521288, -0.2844058539389027196, -0.07201930941427876764 ) ) ;
#31878=EDGE_CURVE ( 'NONE', #21592, #28149, #34909, .T. ) ;
#31879=CIRCLE ( 'NONE', #13514, 0.2539999999999990599 ) ;
#31883=ADVANCED_FACE ( 'NONE', ( #16813 ), #39406, .F. ) ;
#31888=DIRECTION ( 'NONE',  ( 5.188838149069471174E-16, -1.699382548006136313E-16, -1.000000000000000000 ) ) ;
#31889=CARTESIAN_POINT ( 'NONE',  ( -58.36308127269551704, -0.2775048351947507763, 0.1021033997340303756 ) ) ;
#31893=ORIENTED_EDGE ( 'NONE', *, *, #8457, .T. ) ;
#31898=LINE ( 'NONE', #29111, #10411 ) ;
#31905=DIRECTION ( 'NONE',  ( 0.9336303900108815501, 0.3582377630124009560, 4.235673982319039874E-16 ) ) ;
#31906=CYLINDRICAL_SURFACE ( 'NONE', #5817, 0.5080000000000007843 ) ;
#31908=VECTOR ( 'NONE', #38501, 1000.000000000000000 ) ;
#31915=AXIS2_PLACEMENT_3D ( 'NONE', #36997, #11835, #31643 ) ;
#31920=CARTESIAN_POINT ( 'NONE',  ( -57.22211421646271390, 1.778355698664496609, 0.1074917508089385937 ) ) ;
#31930=EDGE_CURVE ( 'NONE', #31070, #12640, #32195, .T. ) ;
#31935=LINE ( 'NONE', #21478, #34987 ) ;
#31937=CARTESIAN_POINT ( 'NONE',  ( -46.60530155212504155, 26.17382724835476537, 0.4656666666666581800 ) ) ;
#31939=CARTESIAN_POINT ( 'NONE',  ( -48.38589991294942649, 19.15920805527091630, 5.452675306770309760 ) ) ;
#31950=CARTESIAN_POINT ( 'NONE',  ( -4.416771755448872128, 71.99420641645033925, 1.524000000000005128 ) ) ;
#31958=ORIENTED_EDGE ( 'NONE', *, *, #32666, .T. ) ;
#31966=VERTEX_POINT ( 'NONE', #23179 ) ;
#31979=EDGE_LOOP ( 'NONE', ( #33823, #2035, #18318, #9470 ) ) ;
#31981=CYLINDRICAL_SURFACE ( 'NONE', #20359, 0.2540000000000006142 ) ;
#31983=CARTESIAN_POINT ( 'NONE',  ( -58.54549369844274054, -0.1193337916060716042, 0.6006683616752106492 ) ) ;
#31989=CARTESIAN_POINT ( 'NONE',  ( -8.216341275949833545, 69.50096819940942794, -1.269999999999995799 ) ) ;
#32004=CARTESIAN_POINT ( 'NONE',  ( -41.23752580366542730, 23.26788267949596190, 1.523999999999994248 ) ) ;
#32005=ORIENTED_EDGE ( 'NONE', *, *, #22941, .F. ) ;
#32006=CARTESIAN_POINT ( 'NONE',  ( -17.14500000000466784, 71.11999999999886768, 1.269999999999998241 ) ) ;
#32012=CARTESIAN_POINT ( 'NONE',  ( -57.39852392895783595, 2.352836174085538357, -1.895304619997750128 ) ) ;
#32014=CARTESIAN_POINT ( 'NONE',  ( -58.43299954449003764, -0.3955325680175592606, -0.3375922266956626894 ) ) ;
#32016=CARTESIAN_POINT ( 'NONE',  ( -3.911441847776591985, 70.75305732235845824, -1.269999999999993801 ) ) ;
#32019=DIRECTION ( 'NONE',  ( -0.8745520943968235761, 0.4849315768086558398, -5.691349986800547879E-16 ) ) ;
#32021=CIRCLE ( 'NONE', #3448, 0.2540000000000045555 ) ;
#32023=CARTESIAN_POINT ( 'NONE',  ( -55.65298819915649631, 5.540485941798511504, -2.823722248809264368 ) ) ;
#32031=CARTESIAN_POINT ( 'NONE',  ( -58.28497307353767809, -0.1385909279409680561, -1.048413496073990905E-14 ) ) ;
#32034=CARTESIAN_POINT ( 'NONE',  ( -17.14500000000466784, 71.11999999999886768, -1.524000000000000909 ) ) ;
#32038=LINE ( 'NONE', #22215, #18765 ) ;
#32039=CARTESIAN_POINT ( 'NONE',  ( -49.09053848811835508, 14.44377425990215436, -0.7907028275641611037 ) ) ;
#32042=CARTESIAN_POINT ( 'NONE',  ( -46.67299067999364581, 26.04487158941909897, -1.318362843711971211 ) ) ;
#32043=CARTESIAN_POINT ( 'NONE',  ( -49.89905798257149883, 16.45710724715066320, 4.946581931842602309 ) ) ;
#32046=CARTESIAN_POINT ( 'NONE',  ( -56.07077906059188166, 6.725046902222183931, 2.233835758070424671 ) ) ;
#32048=ORIENTED_EDGE ( 'NONE', *, *, #7941, .F. ) ;
#32049=CARTESIAN_POINT ( 'NONE',  ( -54.68491514712287227, 9.937145987696780480, -2.757516356780049804 ) ) ;
#32051=PLANE ( 'NONE',  #38722 ) ;
#32052=ORIENTED_EDGE ( 'NONE', *, *, #38139, .F. ) ;
#32057=CARTESIAN_POINT ( 'NONE',  ( -22.95370498042275642, 82.54569470718179502, -1.524000000000005794 ) ) ;
#32062=EDGE_CURVE ( 'NONE', #3374, #23884, #31487, .T. ) ;
#32065=DIRECTION ( 'NONE',  ( -0.8745520943968243532, 0.4849315768086547296, -6.829619984160642269E-16 ) ) ;
#32066=DIRECTION ( 'NONE',  ( 0.8572391118119511155, 0.5149185422762101449, 3.573031421855331076E-16 ) ) ;
#32069=VERTEX_POINT ( 'NONE', #39620 ) ;
#32070=CARTESIAN_POINT ( 'NONE',  ( -58.36783630777247822, -0.2874788285674993449, -0.05365640064145733856 ) ) ;
#32081=AXIS2_PLACEMENT_3D ( 'NONE', #8041, #33406, #4865 ) ;
#32083=EDGE_CURVE ( 'NONE', #2129, #16441, #19251, .T. ) ;
#32084=CARTESIAN_POINT ( 'NONE',  ( -47.61549956331938205, 19.66157307908738261, -5.197827534590572895 ) ) ;
#32085=ORIENTED_EDGE ( 'NONE', *, *, #22477, .F. ) ;
#32089=CARTESIAN_POINT ( 'NONE',  ( -20.05275907367747124, 79.68882802557934042, 1.269999999999994467 ) ) ;
#32093=EDGE_CURVE ( 'NONE', #31609, #31858, #22553, .T. ) ;
#32096=CARTESIAN_POINT ( 'NONE',  ( -17.99070523305417169, 61.93444992276926797, 1.269999999999999574 ) ) ;
#32098=DIRECTION ( 'NONE',  ( 5.188838149069472160E-16, -1.699382548006136559E-16, -1.000000000000000000 ) ) ;
#32100=UNCERTAINTY_MEASURE_WITH_UNIT (LENGTH_MEASURE( 1.000000000000000082E-05 ), #40319, 'distance_accuracy_value', 'NONE');
#32103=ORIENTED_EDGE ( 'NONE', *, *, #30517, .F. ) ;
#32112=CARTESIAN_POINT ( 'NONE',  ( -29.24370919313948036, 62.65993627036882430, 1.269999999999993801 ) ) ;
#32116=EDGE_CURVE ( 'NONE', #7000, #18324, #33653, .T. ) ;
#32129=AXIS2_PLACEMENT_3D ( 'NONE', #13246, #23437, #3048 ) ;
#32132=ORIENTED_EDGE ( 'NONE', *, *, #9989, .T. ) ;
#32138=AXIS2_PLACEMENT_3D ( 'NONE', #21580, #37583, #28207 ) ;
#32142=CARTESIAN_POINT ( 'NONE',  ( -52.53071462815427850, 11.66508355409500908, 4.037383736418494351 ) ) ;
#32143=CARTESIAN_POINT ( 'NONE',  ( -46.68395179480138779, 26.03198510454123848, 1.523999999999990695 ) ) ;
#32145=CARTESIAN_POINT ( 'NONE',  ( -46.68395179480138779, 26.03198510454123848, 1.523999999999991140 ) ) ;
#32146=CARTESIAN_POINT ( 'NONE',  ( -58.66687843194859653, -0.3140260920009522727, 0.3203103694181388961 ) ) ;
#32149=ORIENTED_EDGE ( 'NONE', *, *, #6882, .T. ) ;
#32150=ORIENTED_EDGE ( 'NONE', *, *, #34923, .T. ) ;
#32160=LINE ( 'NONE', #35782, #13090 ) ;
#32173=EDGE_CURVE ( 'NONE', #1003, #1503, #11055, .T. ) ;
#32178=ORIENTED_EDGE ( 'NONE', *, *, #3012, .F. ) ;
#32179=CARTESIAN_POINT ( 'NONE',  ( -41.05189575270515689, 23.09451173561988924, 0.6632222222222170505 ) ) ;
#32187=CARTESIAN_POINT ( 'NONE',  ( -33.20758249455312239, 49.81222039523557044, -1.270000000000005569 ) ) ;
#32191=EDGE_LOOP ( 'NONE', ( #32052, #2890, #8667, #41724 ) ) ;
#32195=CIRCLE ( 'NONE', #1593, 9.048749999999998295 ) ;
#32201=VECTOR ( 'NONE', #34654, 1000.000000000000000 ) ;
#32203=CARTESIAN_POINT ( 'NONE',  ( -32.51099854767154085, 68.28336360077705081, 1.523999999999991140 ) ) ;
#32214=CYLINDRICAL_SURFACE ( 'NONE', #24585, 9.048749999999998295 ) ;
#32215=CARTESIAN_POINT ( 'NONE',  ( -26.01970228765382132, 72.88622078690372064, 1.269999999999992468 ) ) ;
#32222=VERTEX_POINT ( 'NONE', #4061 ) ;
#32223=CARTESIAN_POINT ( 'NONE',  ( -42.18235783619700641, 22.15054559413666624, -1.778153187291473758 ) ) ;
#32224=CIRCLE ( 'NONE', #40419, 0.2539999999999998925 ) ;
#32228=ADVANCED_FACE ( 'NONE', ( #24246 ), #17020, .T. ) ;
#32230=CARTESIAN_POINT ( 'NONE',  ( -58.04839436022131594, 0.9580029038198520919, -1.310276026340456479 ) ) ;
#32232=CARTESIAN_POINT ( 'NONE',  ( -58.16644339752609483, 0.1874380212898556775, -0.9010643026010315415 ) ) ;
#32238=CARTESIAN_POINT ( 'NONE',  ( -58.83227707057486811, -0.08366279997995551554, -1.273395421382134774E-15 ) ) ;
#32239=AXIS2_PLACEMENT_3D ( 'NONE', #7899, #4298, #40494 ) ;
#32248=CARTESIAN_POINT ( 'NONE',  ( -57.34787435976332404, 1.552391619547691004, -1.028525222821079960E-14 ) ) ;
#32252=AXIS2_PLACEMENT_3D ( 'NONE', #22371, #23209, #6224 ) ;
#32256=CARTESIAN_POINT ( 'NONE',  ( -47.25474348537468927, 18.41641806589853303, -3.087470713317427506 ) ) ;
#32257=EDGE_LOOP ( 'NONE', ( #30658, #9565, #187, #17736 ) ) ;
#32259=CARTESIAN_POINT ( 'NONE',  ( -48.20156657701304681, 19.76063879377972654, 5.201425424509390716 ) ) ;
#32260=CARTESIAN_POINT ( 'NONE',  ( -49.26208180856533403, 17.44698433589570641, 5.073594244243587958 ) ) ;
#32263=CARTESIAN_POINT ( 'NONE',  ( -56.26154134543016738, 7.775270144418325202, 0.1976385065555384957 ) ) ;
#32266=CARTESIAN_POINT ( 'NONE',  ( -54.50298212578950796, 9.515077312548310573, -3.630897911711918002 ) ) ;
#32268=ORIENTED_EDGE ( 'NONE', *, *, #32458, .F. ) ;
#32279=DIRECTION ( 'NONE',  ( 5.188838149069472160E-16, -1.699382548006136559E-16, -1.000000000000000000 ) ) ;
#32281=DIRECTION ( 'NONE',  ( -0.8745520943968162486, 0.4849315768086691625, -5.424246918827962036E-16 ) ) ;
#32282=VERTEX_POINT ( 'NONE', #41298 ) ;
#32285=CARTESIAN_POINT ( 'NONE',  ( -58.36986766252679359, -0.2916724680131291825, -0.008878031541896621096 ) ) ;
#32296=CARTESIAN_POINT ( 'NONE',  ( -47.67648637180143822, 19.71513033058998232, -5.327979952964785326 ) ) ;
#32297=VERTEX_POINT ( 'NONE', #2540 ) ;
#32305=DIRECTION ( 'NONE',  ( -5.188838149069471174E-16, 1.699382548006136313E-16, 1.000000000000000000 ) ) ;
#32306=LINE ( 'NONE', #41911, #35855 ) ;
#32307=EDGE_CURVE ( 'NONE', #25039, #30173, #19834, .T. ) ;
#32309=EDGE_LOOP ( 'NONE', ( #35303, #11102, #26500, #20448 ) ) ;
#32320=DIRECTION ( 'NONE',  ( -0.1906721105965039909, 0.9816537812491094028, -2.657572025465702696E-16 ) ) ;
#32321=CARTESIAN_POINT ( 'NONE',  ( -17.14500000000466784, 71.11999999999886768, 1.523999999999998689 ) ) ;
#32322=LINE ( 'NONE', #2536, #39217 ) ;
#32331=ORIENTED_EDGE ( 'NONE', *, *, #40180, .F. ) ;
#32332=EDGE_CURVE ( 'NONE', #14467, #6398, #40179, .T. ) ;
#32338=EDGE_CURVE ( 'NONE', #1116, #38737, #36095, .T. ) ;
#32347=CARTESIAN_POINT ( 'NONE',  ( -48.84023001699601707, 18.03124979360562463, 5.100068162039153918 ) ) ;
#32348=CARTESIAN_POINT ( 'NONE',  ( -46.60530155212503445, 26.17382724835477958, 1.523999999999990917 ) ) ;
#32352=CARTESIAN_POINT ( 'NONE',  ( -47.07934102874904170, 22.98505637820369429, 3.579966862081928713 ) ) ;
#32357=ORIENTED_EDGE ( 'NONE', *, *, #16771, .F. ) ;
#32366=CARTESIAN_POINT ( 'NONE',  ( -23.16987411132078023, 77.52691185402750307, -1.524000000000004906 ) ) ;
#32370=AXIS2_PLACEMENT_3D ( 'NONE', #26776, #16755, #13981 ) ;
#32371=FACE_OUTER_BOUND ( 'NONE', #1430, .T. ) ;
#32374=ORIENTED_EDGE ( 'NONE', *, *, #38050, .T. ) ;
#32383=CARTESIAN_POINT ( 'NONE',  ( -44.27221412529542022, 20.06621383160478445, 0.8981538560692690076 ) ) ;
#32390=CARTESIAN_POINT ( 'NONE',  ( -9.960492004070044203, 64.81807050032566053, 1.524000000000003352 ) ) ;
#32394=ADVANCED_FACE ( 'NONE', ( #28501 ), #29974, .T. ) ;
#32398=DIRECTION ( 'NONE',  ( 0.9816537812491089587, 0.1906721105965065444, 4.769617732184475162E-16 ) ) ;
#32400=CARTESIAN_POINT ( 'NONE',  ( -58.68272167409660511, -0.3140646606565877796, 0.3072153925275410424 ) ) ;
#32402=DIRECTION ( 'NONE',  ( -0.8745520943968241312, 0.4849315768086548406, -5.691349986800536046E-16 ) ) ;
#32404=AXIS2_PLACEMENT_3D ( 'NONE', #40291, #27487, #34513 ) ;
#32405=ADVANCED_FACE ( 'NONE', ( #18060 ), #8495, .T. ) ;
#32407=EDGE_CURVE ( 'NONE', #16319, #1811, #12280, .T. ) ;
#32416=DIRECTION ( 'NONE',  ( 5.188838149069472160E-16, -1.699382548006136559E-16, -1.000000000000000000 ) ) ;
#32420=FACE_OUTER_BOUND ( 'NONE', #14774, .T. ) ;
#32425=ORIENTED_EDGE ( 'NONE', *, *, #26363, .T. ) ;
#32426=CARTESIAN_POINT ( 'NONE',  ( -23.62918761621517660, 82.45577215708875940, -1.524000000000006017 ) ) ;
#32427=ORIENTED_EDGE ( 'NONE', *, *, #38572, .T. ) ;
#32428=DIRECTION ( 'NONE',  ( -0.8745520943968005945, 0.4849315768086974732, -6.829619984160627478E-16 ) ) ;
#32433=CARTESIAN_POINT ( 'NONE',  ( -58.46831931685589723, 0.04886852696691689618, -0.7470671021170768311 ) ) ;
#32434=ORIENTED_EDGE ( 'NONE', *, *, #21007, .F. ) ;
#32435=CARTESIAN_POINT ( 'NONE',  ( -58.58343337229877079, -0.6799398409036180313, -0.1767901212656000642 ) ) ;
#32440=CARTESIAN_POINT ( 'NONE',  ( -10.75478607932181241, 82.07015292912137738, 1.524000000000000243 ) ) ;
#32443=CARTESIAN_POINT ( 'NONE',  ( -57.66338803320029882, 2.692357263605615891, -1.869785753600856637 ) ) ;
#32447=VERTEX_POINT ( 'NONE', #16335 ) ;
#32452=TOROIDAL_SURFACE ( 'NONE', #5954, 0.3810000000000014486, 0.2540000000000000036 ) ;
#32453=CARTESIAN_POINT ( 'NONE',  ( -47.93564525088164885, 15.36257551998183857, -8.154853246613427015E-15 ) ) ;
#32458=EDGE_CURVE ( 'NONE', #21262, #702, #29264, .T. ) ;
#32461=DIRECTION ( 'NONE',  ( -0.8745520943968249084, 0.4849315768086533418, -5.271987356194193006E-16 ) ) ;
#32463=CARTESIAN_POINT ( 'NONE',  ( -46.36222913602039597, 19.75614878210438263, -3.583538483381434325 ) ) ;
#32465=CARTESIAN_POINT ( 'NONE',  ( -46.96327221648714101, 24.95754849389490815, 2.007562630684373239 ) ) ;
#32466=CARTESIAN_POINT ( 'NONE',  ( -28.74159376897886276, 60.61225341505600284, -1.270000000000005125 ) ) ;
#32468=CARTESIAN_POINT ( 'NONE',  ( -58.37116772670351850, -0.2940390518722524327, -2.603646672650065119E-13 ) ) ;
#32470=CARTESIAN_POINT ( 'NONE',  ( -56.90265763162630464, 5.074588416753345044, 1.064700026618647266 ) ) ;
#32471=CARTESIAN_POINT ( 'NONE',  ( -56.80697847991661575, 4.636179106009441497, 2.484889565616565488 ) ) ;
#32474=CARTESIAN_POINT ( 'NONE',  ( -51.75204694603132083, 19.49597778360960021, -0.7628839639000161155 ) ) ;
#32481=DIRECTION ( 'NONE',  ( -5.188838149069471174E-16, 1.699382548006136313E-16, 1.000000000000000000 ) ) ;
#32485=CARTESIAN_POINT ( 'NONE',  ( -19.64403260974359355, 72.50569198072959409, 1.269999999999996909 ) ) ;
#32489=DIRECTION ( 'NONE',  ( 0.8745520943968235761, -0.4849315768086558398, 8.537024980200821818E-16 ) ) ;
#32490=EDGE_LOOP ( 'NONE', ( #1497, #39129, #41859, #9652 ) ) ;
#32493=CARTESIAN_POINT ( 'NONE',  ( -58.30426395036794673, -0.1531247907950611109, -0.3258712918401721059 ) ) ;
#32508=CARTESIAN_POINT ( 'NONE',  ( -47.04837031381860157, 23.61299024743492581, -3.054033755318078303 ) ) ;
#32511=CARTESIAN_POINT ( 'NONE',  ( -33.20758249455312239, 49.81222039523557044, 1.269999999999993578 ) ) ;
#32531=CARTESIAN_POINT ( 'NONE',  ( -17.14500000000466784, 71.11999999999886768, -1.524000000000000909 ) ) ;
#32536=DIRECTION ( 'NONE',  ( 5.188838149069472160E-16, -1.699382548006136559E-16, -1.000000000000000000 ) ) ;
#32541=EDGE_LOOP ( 'NONE', ( #6131, #23849, #25229, #11635, #18245 ) ) ;
#32555=CARTESIAN_POINT ( 'NONE',  ( -47.84356795211458291, 19.38525671449504983, 5.197506975155153697 ) ) ;
#32557=DIRECTION ( 'NONE',  ( -0.8745520943968249084, 0.4849315768086533418, -5.271987356194193006E-16 ) ) ;
#32558=CARTESIAN_POINT ( 'NONE',  ( -46.81005371095109524, 25.73327194510133253, 1.583310528698471664 ) ) ;
#32562=ORIENTED_EDGE ( 'NONE', *, *, #31345, .T. ) ;
#32565=AXIS2_PLACEMENT_3D ( 'NONE', #2878, #41860, #733 ) ;
#32569=TOROIDAL_SURFACE ( 'NONE', #42115, 0.3809999999999990616, 0.2540000000000000036 ) ;
#32570=CARTESIAN_POINT ( 'NONE',  ( -47.48049929620759002, 23.18975938597035125, -2.730405167055939497 ) ) ;
#32574=DIRECTION ( 'NONE',  ( 0.1906721105965055174, -0.9816537812491091808, 0.000000000000000000 ) ) ;
#32591=ORIENTED_EDGE ( 'NONE', *, *, #37363, .F. ) ;
#32593=CARTESIAN_POINT ( 'NONE',  ( -46.49274047292066570, 18.53875678104565594, 2.063467562158682433 ) ) ;
#32600=DIRECTION ( 'NONE',  ( 5.188838149069472160E-16, -1.699382548006136559E-16, -1.000000000000000000 ) ) ;
#32605=ORIENTED_EDGE ( 'NONE', *, *, #5289, .F. ) ;
#32613=DIRECTION ( 'NONE',  ( 0.9454731675810308378, -0.3256999990547930213, -6.328166980064887941E-15 ) ) ;
#32617=LINE ( 'NONE', #32203, #1975 ) ;
#32625=CARTESIAN_POINT ( 'NONE',  ( -10.84307050033138786, 78.30450799593342026, 1.270000000000000240 ) ) ;
#32626=DIRECTION ( 'NONE',  ( -0.8745520943968249084, 0.4849315768086533418, -5.271987356194193006E-16 ) ) ;
#32629=CARTESIAN_POINT ( 'NONE',  ( -28.76494711669534610, 76.52965637509277030, 1.269999999999990470 ) ) ;
#32636=CARTESIAN_POINT ( 'NONE',  ( -24.50334120614357047, 81.61487340491997600, -1.524000000000006461 ) ) ;
#32637=AXIS2_PLACEMENT_3D ( 'NONE', #20360, #7610, #36581 ) ;
#32639=FACE_OUTER_BOUND ( 'NONE', #35980, .T. ) ;
#32644=CARTESIAN_POINT ( 'NONE',  ( -58.57514867739262598, -0.1811137290223177321, -0.5238340084838408739 ) ) ;
#32646=CARTESIAN_POINT ( 'NONE',  ( -58.34765594471348749, -0.2451624547642194951, -0.1853313705893772922 ) ) ;
#32651=ADVANCED_FACE ( 'NONE', ( #28913 ), #42141, .T. ) ;
#32655=CARTESIAN_POINT ( 'NONE',  ( -57.95878807693440393, 1.295030275130740094, -1.504629864475988787 ) ) ;
#32656=ADVANCED_FACE ( 'NONE', ( #25926 ), #39490, .T. ) ;
#32665=AXIS2_PLACEMENT_3D ( 'NONE', #18082, #15094, #25113 ) ;
#32666=EDGE_CURVE ( 'NONE', #6241, #40015, #8971, .T. ) ;
#32672=CARTESIAN_POINT ( 'NONE',  ( -53.68435271313694557, 11.12367579685427721, -3.945100831076026715 ) ) ;
#32673=CARTESIAN_POINT ( 'NONE',  ( -45.30933510662926977, 19.89173180141312614, -2.333898071402948027 ) ) ;
#32674=ORIENTED_EDGE ( 'NONE', *, *, #31562, .F. ) ;
#32677=DIRECTION ( 'NONE',  ( 0.9336303900108852138, 0.3582377630123916301, 4.235673982319075372E-16 ) ) ;
#32681=CARTESIAN_POINT ( 'NONE',  ( -8.480639930781094904, 68.51064353654967931, -1.523999999999995802 ) ) ;
#32683=CARTESIAN_POINT ( 'NONE',  ( -54.50298212578950796, 9.515077312548310573, 3.630897911711898018 ) ) ;
#32684=CARTESIAN_POINT ( 'NONE',  ( -57.95878807693440393, 1.295030275130740094, 1.504629864475967915 ) ) ;
#32688=CARTESIAN_POINT ( 'NONE',  ( -54.55302389503632554, 12.80492160976152327, -0.5954867740798109876 ) ) ;
#32696=CARTESIAN_POINT ( 'NONE',  ( -17.32429653712378936, 61.56493206124108042, 1.524000000000000243 ) ) ;
#32702=CARTESIAN_POINT ( 'NONE',  ( -48.55954782883388532, 18.47106080339405310, -5.181360474636990787 ) ) ;
#32706=VERTEX_POINT ( 'NONE', #287 ) ;
#32708=DIRECTION ( 'NONE',  ( -0.8745520943968235761, 0.4849315768086558398, -4.268512490100410909E-16 ) ) ;
#32714=ADVANCED_FACE ( 'NONE', ( #23241 ), #7510, .T. ) ;
#32715=CIRCLE ( 'NONE', #25886, 0.3810000000000015041 ) ;
#32723=CARTESIAN_POINT ( 'NONE',  ( -25.56614996202194590, 73.65611136973726047, 1.523999999999993804 ) ) ;
#32724=TOROIDAL_SURFACE ( 'NONE', #12956, 8.794749999999996959, 0.2540000000000000036 ) ;
#32725=CARTESIAN_POINT ( 'NONE',  ( -48.53848336910535011, 19.22582880449973075, -5.323527254358048744 ) ) ;
#32726=ORIENTED_EDGE ( 'NONE', *, *, #4291, .F. ) ;
#32736=DIRECTION ( 'NONE',  ( -5.188838149069471174E-16, 1.699382548006136313E-16, 1.000000000000000000 ) ) ;
#32744=DIRECTION ( 'NONE',  ( 5.188838149069472160E-16, -1.699382548006136559E-16, -1.000000000000000000 ) ) ;
#32756=DIRECTION ( 'NONE',  ( 5.188838149069472160E-16, -1.699382548006136559E-16, -1.000000000000000000 ) ) ;
#32772=TOROIDAL_SURFACE ( 'NONE', #39590, 3.111499999999999488, 0.2540000000000000036 ) ;
#32775=AXIS2_PLACEMENT_3D ( 'NONE', #3693, #10483, #7300 ) ;
#32777=CARTESIAN_POINT ( 'NONE',  ( -11.53797084252497562, 82.58007221317646440, 1.523999999999999577 ) ) ;
#32779=CARTESIAN_POINT ( 'NONE',  ( -50.22242345129090779, 22.76272812237061771, -9.508731853559545367E-15 ) ) ;
#32781=CARTESIAN_POINT ( 'NONE',  ( -52.06546789126484498, 13.38259882428268632, 4.575081192416372566 ) ) ;
#32782=CARTESIAN_POINT ( 'NONE',  ( -58.72811565343341300, -0.3134725424711655162, 0.2575438388786236987 ) ) ;
#32784=DIRECTION ( 'NONE',  ( 0.8572391118119472297, 0.5149185422762166953, 0.000000000000000000 ) ) ;
#32791=CARTESIAN_POINT ( 'NONE',  ( -46.81330379368907302, 25.73549360603863434, -1.450859712031395521 ) ) ;
#32803=CARTESIAN_POINT ( 'NONE',  ( -4.377002418771855474, 72.24507371176854065, -1.523999999999994248 ) ) ;
#32808=AXIS2_PLACEMENT_3D ( 'NONE', #8955, #21922, #8745 ) ;
#32810=ORIENTED_EDGE ( 'NONE', *, *, #4075, .T. ) ;
#32811=VERTEX_POINT ( 'NONE', #39042 ) ;
#32812=CARTESIAN_POINT ( 'NONE',  ( -44.40685758373553682, 19.43703734468912714, 0.2085933842879050815 ) ) ;
#32819=DIRECTION ( 'NONE',  ( -0.8745520943968235761, 0.4849315768086558953, -5.361993529360570985E-16 ) ) ;
#32823=AXIS2_PLACEMENT_3D ( 'NONE', #1818, #30766, #34396 ) ;
#32827=CARTESIAN_POINT ( 'NONE',  ( -28.65049350906917880, 77.81814547195517662, 1.269999999999991136 ) ) ;
#32828=DIRECTION ( 'NONE',  ( -0.8745520943968243532, 0.4849315768086547296, -5.361993529360573944E-16 ) ) ;
#32831=AXIS2_PLACEMENT_3D ( 'NONE', #30369, #10777, #7387 ) ;
#32840=DIRECTION ( 'NONE',  ( -0.8745520943968235761, 0.4849315768086558398, -4.268512490100410909E-16 ) ) ;
#32841=DIRECTION ( 'NONE',  ( -5.188838149069471174E-16, 1.699382548006136313E-16, 1.000000000000000000 ) ) ;
#32851=VERTEX_POINT ( 'NONE', #23031 ) ;
#32854=CARTESIAN_POINT ( 'NONE',  ( -15.42835734045148577, 79.74558783746837776, 1.523999999999998023 ) ) ;
#32859=EDGE_CURVE ( 'NONE', #8461, #8441, #35854, .T. ) ;
#32860=CARTESIAN_POINT ( 'NONE',  ( -58.79373602274613830, -0.2918016666370280565, -0.1550872664390397226 ) ) ;
#32862=DIRECTION ( 'NONE',  ( 5.188838149069472160E-16, -1.699382548006136559E-16, -1.000000000000000000 ) ) ;
#32869=CARTESIAN_POINT ( 'NONE',  ( -58.23017998949752183, 0.6774554162835566551, -1.209604144815722426 ) ) ;
#32871=ORIENTED_EDGE ( 'NONE', *, *, #41808, .F. ) ;
#32886=ADVANCED_FACE ( 'NONE', ( #29661 ), #3442, .T. ) ;
#32887=EDGE_CURVE ( 'NONE', #37020, #20172, #28606, .T. ) ;
#32888=CARTESIAN_POINT ( 'NONE',  ( -52.94148447887670272, 9.133269539094115430, -0.6394659809470596423 ) ) ;
#32890=CARTESIAN_POINT ( 'NONE',  ( -5.591489108514605455, 77.73497692594764885, -1.523999999999996025 ) ) ;
#32891=CYLINDRICAL_SURFACE ( 'NONE', #20650, 0.2539999999999998925 ) ;
#32892=CARTESIAN_POINT ( 'NONE',  ( -30.15519950990045572, 69.97033940222175374, 1.269999999999990692 ) ) ;
#32894=EDGE_CURVE ( 'NONE', #18166, #4212, #3482, .T. ) ;
#32897=DIRECTION ( 'NONE',  ( -0.1565721916418034432, -0.9876665170007953298, 8.659954811667511346E-17 ) ) ;
#32898=CARTESIAN_POINT ( 'NONE',  ( -57.70501761738805158, 2.967533670478833763, 0.5494564739991059099 ) ) ;
#32899=CARTESIAN_POINT ( 'NONE',  ( -57.67794393518098417, 1.927849678527493449, 1.763631237166035648 ) ) ;
#32902=ORIENTED_EDGE ( 'NONE', *, *, #2504, .F. ) ;
#32903=CARTESIAN_POINT ( 'NONE',  ( -51.68405183998543606, 20.46365084016696301, -1.077913170022978826E-14 ) ) ;
#32911=CIRCLE ( 'NONE', #1625, 0.2539999999999986158 ) ;
#32917=CARTESIAN_POINT ( 'NONE',  ( -48.32642138504052554, 18.79167496732631548, -5.205639462496891134 ) ) ;
#32919=EDGE_LOOP ( 'NONE', ( #26917, #15485, #16833, #17117 ) ) ;
#32923=CARTESIAN_POINT ( 'NONE',  ( -57.77469323499624920, 0.9920357466726326123, -1.126265832864315808 ) ) ;
#32926=AXIS2_PLACEMENT_3D ( 'NONE', #17105, #7328, #36093 ) ;
#32933=VERTEX_POINT ( 'NONE', #6876 ) ;
#32936=AXIS2_PLACEMENT_3D ( 'NONE', #33376, #23554, #13976 ) ;
#32937=CARTESIAN_POINT ( 'NONE',  ( -58.85382722430585289, -0.1409386484715794419, -5.573042720897973618E-15 ) ) ;
#32939=CARTESIAN_POINT ( 'NONE',  ( -47.19936399096371105, 20.24790404726484283, -5.251082349106865443 ) ) ;
#32943=FACE_OUTER_BOUND ( 'NONE', #2308, .T. ) ;
#32944=EDGE_CURVE ( 'NONE', #4212, #26041, #12378, .T. ) ;
#32946=AXIS2_PLACEMENT_3D ( 'NONE', #26855, #10869, #30048 ) ;
#32954=DIRECTION ( 'NONE',  ( 0.8745520943968230210, -0.4849315768086570611, 6.829619984160674809E-16 ) ) ;
#32955=ADVANCED_FACE ( 'NONE', ( #4532 ), #30492, .F. ) ;
#32957=ORIENTED_EDGE ( 'NONE', *, *, #34303, .T. ) ;
#32959=CARTESIAN_POINT ( 'NONE',  ( -17.14500000000466784, 71.11999999999886768, 1.523999999999998689 ) ) ;
#32960=AXIS2_PLACEMENT_3D ( 'NONE', #19480, #13098, #32489 ) ;
#32970=CARTESIAN_POINT ( 'NONE',  ( -46.60530155212503445, 26.17382724835477958, 1.269999999999988916 ) ) ;
#32975=DIRECTION ( 'NONE',  ( 5.188838149069472160E-16, -1.699382548006136559E-16, -1.000000000000000000 ) ) ;
#32979=EDGE_LOOP ( 'NONE', ( #2040, #5371, #41753, #20558 ) ) ;
#32986=VERTEX_POINT ( 'NONE', #24099 ) ;
#32995=CARTESIAN_POINT ( 'NONE',  ( -46.68567580513006732, 26.01863749727769104, 1.329804637746865081 ) ) ;
#32996=CARTESIAN_POINT ( 'NONE',  ( -47.97936104919185851, 23.38005451144316993, 1.568716696360799912 ) ) ;
#32997=CARTESIAN_POINT ( 'NONE',  ( -17.14500000000466784, 71.11999999999886768, 1.269999999999998241 ) ) ;
#32999=CARTESIAN_POINT ( 'NONE',  ( -54.98111839650035648, 8.542840639972862249, 3.427624633821322320 ) ) ;
#33000=CARTESIAN_POINT ( 'NONE',  ( -17.14500000000466784, 71.11999999999886768, -1.524000000000000909 ) ) ;
#33004=CARTESIAN_POINT ( 'NONE',  ( -46.52557095416602806, 23.25943309041075224, 3.047882326417268750 ) ) ;
#33027=CARTESIAN_POINT ( 'NONE',  ( -42.88395384449221126, 21.55219572468337219, 1.583305067638063779 ) ) ;
#33030=AXIS2_PLACEMENT_3D ( 'NONE', #12097, #38092, #8907 ) ;
#33050=CIRCLE ( 'NONE', #18070, 0.2539999999999960067 ) ;
#33059=DIRECTION ( 'NONE',  ( -5.188838149069471174E-16, 1.699382548006136313E-16, 1.000000000000000000 ) ) ;
#33060=CYLINDRICAL_SURFACE ( 'NONE', #17822, 0.5080000000000000071 ) ;
#33066=DIRECTION ( 'NONE',  ( -0.9454731675810326141, 0.3256999990547876367, -5.459396135145336213E-16 ) ) ;
#33069=DIRECTION ( 'NONE',  ( 0.9876665170007974393, -0.1565721916417901483, 8.537024980200831679E-16 ) ) ;
#33074=CARTESIAN_POINT ( 'NONE',  ( -58.82991074935231524, -0.2577531494038359794, -1.058401375502683064E-14 ) ) ;
#33075=ORIENTED_EDGE ( 'NONE', *, *, #33091, .F. ) ;
#33078=DIRECTION ( 'NONE',  ( -0.9998501190848636533, -0.01731298258487879230, 2.441448296158441227E-15 ) ) ;
#33081=DIRECTION ( 'NONE',  ( -0.8745520943968245753, 0.4849315768086539524, -5.691349986800526185E-16 ) ) ;
#33085=ORIENTED_EDGE ( 'NONE', *, *, #30869, .F. ) ;
#33088=AXIS2_PLACEMENT_3D ( 'NONE', #15837, #6274, #22013 ) ;
#33091=EDGE_CURVE ( 'NONE', #37691, #8945, #11110, .T. ) ;
#33092=DIRECTION ( 'NONE',  ( -0.8745520943968243532, 0.4849315768086547296, -5.361993529360573944E-16 ) ) ;
#33093=CARTESIAN_POINT ( 'NONE',  ( -58.36720124622708994, -0.2861505079046616773, 0.06388190288942181827 ) ) ;
#33100=LINE ( 'NONE', #36709, #19498 ) ;
#33101=CARTESIAN_POINT ( 'NONE',  ( -50.43530108972998960, 14.71354995532366594, -3.653486772774936053 ) ) ;
#33103=FACE_OUTER_BOUND ( 'NONE', #28833, .T. ) ;
#33104=CARTESIAN_POINT ( 'NONE',  ( -46.93285886088614234, 25.18477106413915934, -1.854137101283168887 ) ) ;
#33105=CARTESIAN_POINT ( 'NONE',  ( -5.525052883313952279, 65.71034362490503611, 1.270000000000004459 ) ) ;
#33106=CARTESIAN_POINT ( 'NONE',  ( -29.43804252118301079, 67.00854438735578356, -1.269999999999767981 ) ) ;
#33108=FACE_OUTER_BOUND ( 'NONE', #29744, .T. ) ;
#33110=CARTESIAN_POINT ( 'NONE',  ( -58.40930376703802551, 1.028767233150276628, 0.4283228411258263035 ) ) ;
#33111=TOROIDAL_SURFACE ( 'NONE', #26960, 0.3810000000000002829, 0.2540000000000000036 ) ;
#33112=CARTESIAN_POINT ( 'NONE',  ( -55.73247374733729487, 5.492406230130003841, 2.854677165782097514 ) ) ;
#33116=CARTESIAN_POINT ( 'NONE',  ( -58.07447437077728125, 1.735896131820596766, -1.499107834811110873 ) ) ;
#33129=LINE ( 'NONE', #10738, #31781 ) ;
#33130=CARTESIAN_POINT ( 'NONE',  ( -11.56352105402813280, 78.55269139521317356, 1.270000000000000018 ) ) ;
#33131=ORIENTED_EDGE ( 'NONE', *, *, #20419, .F. ) ;
#33134=CARTESIAN_POINT ( 'NONE',  ( -58.20606554041528824, 0.05853145357879600830, -0.5431157087058823274 ) ) ;
#33152=CARTESIAN_POINT ( 'NONE',  ( -52.97391985390434144, 12.30611266682019789, -4.247241762254921227 ) ) ;
#33153=VECTOR ( 'NONE', #26492, 1000.000000000000000 ) ;
#33156=CARTESIAN_POINT ( 'NONE',  ( -17.32429653712378936, 61.56493206124108042, -1.523999999999999355 ) ) ;
#33164=TOROIDAL_SURFACE ( 'NONE', #37894, 2.286000000000000032, 0.2540000000000000036 ) ;
#33165=ADVANCED_FACE ( 'NONE', ( #37513 ), #1547, .F. ) ;
#33169=CYLINDRICAL_SURFACE ( 'NONE', #25786, 9.048749999999998295 ) ;
#33173=CARTESIAN_POINT ( 'NONE',  ( -41.06677624517575964, 23.07857903943748212, 1.269999999996107354 ) ) ;
#33178=DIRECTION ( 'NONE',  ( -0.9998501190848640974, -0.01731298258485272981, -8.537024980200786319E-16 ) ) ;
#33180=CIRCLE ( 'NONE', #5296, 0.6350000000000014522 ) ;
#33185=CARTESIAN_POINT ( 'NONE',  ( -58.68272167409650564, -0.3140646606568653354, -0.3072153925272262387 ) ) ;
#33192=ADVANCED_FACE ( 'NONE', ( #40524 ), #31123, .F. ) ;
#33196=EDGE_CURVE ( 'NONE', #20421, #26517, #37309, .T. ) ;
#33198=ORIENTED_EDGE ( 'NONE', *, *, #24135, .F. ) ;
#33200=CARTESIAN_POINT ( 'NONE',  ( -8.265412277504241345, 72.86149316418863009, -1.523999999999996469 ) ) ;
#33201=CARTESIAN_POINT ( 'NONE',  ( -31.81551635377703136, 53.03133741989296368, -1.270000000000005347 ) ) ;
#33205=ADVANCED_FACE ( 'NONE', ( #8125 ), #16055, .T. ) ;
#33208=CARTESIAN_POINT ( 'NONE',  ( -57.66147120254575498, 1.236620361205436502, 1.243523781513556914 ) ) ;
#33209=CARTESIAN_POINT ( 'NONE',  ( -47.36536141536632982, 24.59964078100214380, 1.062456689557159439 ) ) ;
#33211=CARTESIAN_POINT ( 'NONE',  ( -54.97180548219925100, 8.422794459035404913, 3.467293221275778325 ) ) ;
#33212=CARTESIAN_POINT ( 'NONE',  ( -56.97070633664897343, 3.259530599714575150, 2.205540024717516090 ) ) ;
#33214=DIRECTION ( 'NONE',  ( 5.188838149069472160E-16, -1.699382548006136559E-16, -1.000000000000000000 ) ) ;
#33215=EDGE_LOOP ( 'NONE', ( #31630, #30118, #34388, #892 ) ) ;
#33216=CARTESIAN_POINT ( 'NONE',  ( -45.91718695868514288, 25.22619731686664224, 1.578102078770057037 ) ) ;
#33240=CARTESIAN_POINT ( 'NONE',  ( -41.90039389258884484, 22.27519970079744382, 1.481527307957004602 ) ) ;
#33255=CARTESIAN_POINT ( 'NONE',  ( -17.09258512000246100, 84.17916046765628835, -1.524000000000002908 ) ) ;
#33257=CIRCLE ( 'NONE', #37324, 0.5080000000000000071 ) ;
#33269=CYLINDRICAL_SURFACE ( 'NONE', #22891, 9.048749999999998295 ) ;
#33270=CARTESIAN_POINT ( 'NONE',  ( -8.744179778605065678, 67.99101067706818924, 1.270000000000003348 ) ) ;
#33272=DIRECTION ( 'NONE',  ( 0.8745520943968243532, -0.4849315768086547296, 6.829619984160642269E-16 ) ) ;
#33277=DIRECTION ( 'NONE',  ( 0.3256999990547836399, 0.9454731675810339464, 0.000000000000000000 ) ) ;
#33278=CARTESIAN_POINT ( 'NONE',  ( -8.428339483816529309, 74.57444062528223583, -1.269999999999996909 ) ) ;
#33280=VERTEX_POINT ( 'NONE', #22141 ) ;
#33285=CARTESIAN_POINT ( 'NONE',  ( -58.62772660637192956, -0.2868617839840607586, -0.3825110252948605849 ) ) ;
#33286=ORIENTED_EDGE ( 'NONE', *, *, #39881, .T. ) ;
#33287=CARTESIAN_POINT ( 'NONE',  ( -11.56352105402813280, 78.55269139521317356, -1.523999999999999133 ) ) ;
#33296=FACE_OUTER_BOUND ( 'NONE', #16691, .T. ) ;
#33309=AXIS2_PLACEMENT_3D ( 'NONE', #22466, #35497, #19290 ) ;
#33310=CARTESIAN_POINT ( 'NONE',  ( -50.29507671575589001, 15.72791930032348873, -4.796563717952116335 ) ) ;
#33315=CARTESIAN_POINT ( 'NONE',  ( -30.55042969354924765, 56.28656473928203496, -1.524000000000195421 ) ) ;
#33317=CARTESIAN_POINT ( 'NONE',  ( -46.78334400223545231, 25.31617564245998508, 1.751383154100511597 ) ) ;
#33319=CARTESIAN_POINT ( 'NONE',  ( -58.05614784158871799, 2.052449344323428626, 0.2046694337772680672 ) ) ;
#33322=ORIENTED_EDGE ( 'NONE', *, *, #20858, .T. ) ;
#33323=CARTESIAN_POINT ( 'NONE',  ( -57.92473815682701144, 2.127617342915319565, -1.480748064241608430 ) ) ;
#33325=ORIENTED_EDGE ( 'NONE', *, *, #6096, .T. ) ;
#33341=CARTESIAN_POINT ( 'NONE',  ( -57.98023336920307003, 0.5472916609800171361, -0.8843171072923534659 ) ) ;
#33346=CARTESIAN_POINT ( 'NONE',  ( -42.34481381083929818, 23.19759442052183473, -1.554397948409621755 ) ) ;
#33348=AXIS2_PLACEMENT_3D ( 'NONE', #28980, #36022, #41796 ) ;
#33351=ORIENTED_EDGE ( 'NONE', *, *, #20338, .F. ) ;
#33354=CARTESIAN_POINT ( 'NONE',  ( -24.24369025645184905, 82.02711331519694227, -1.270000000000006457 ) ) ;
#33356=CARTESIAN_POINT ( 'NONE',  ( -49.01671973967521012, 18.67808020721676954, -5.174630477995056488 ) ) ;
#33357=DIRECTION ( 'NONE',  ( -0.8572391118119521147, -0.5149185422762083686, 1.001946476563074719E-16 ) ) ;
#33364=CARTESIAN_POINT ( 'NONE',  ( -41.35619903644352036, 22.77303286471995136, -1.271070091490047238 ) ) ;
#33370=FACE_OUTER_BOUND ( 'NONE', #21868, .T. ) ;
#33372=CARTESIAN_POINT ( 'NONE',  ( -36.79765817521327165, 27.64956762128696610, 1.269999999999995577 ) ) ;
#33376=CARTESIAN_POINT ( 'NONE',  ( -16.71197878298170991, 83.87086364642222236, 1.269999999999996687 ) ) ;
#33378=ORIENTED_EDGE ( 'NONE', *, *, #16727, .T. ) ;
#33381=DIRECTION ( 'NONE',  ( -0.7517731442105904938, 0.6594218222380290317, 3.321276712443281495E-16 ) ) ;
#33384=ORIENTED_EDGE ( 'NONE', *, *, #3870, .F. ) ;
#33388=CARTESIAN_POINT ( 'NONE',  ( -57.74919803515421535, 1.101601998901122537, -1.404840701337578990 ) ) ;
#33389=DIRECTION ( 'NONE',  ( 0.8745520943968260186, -0.4849315768086515099, 8.537024980200745890E-16 ) ) ;
#33402=ADVANCED_FACE ( 'NONE', ( #38574 ), #28968, .T. ) ;
#33406=DIRECTION ( 'NONE',  ( -0.7548010569845284845, -0.6559537821943240976, -2.801824109679630066E-16 ) ) ;
#33410=LINE ( 'NONE', #33832, #39668 ) ;
#33412=CARTESIAN_POINT ( 'NONE',  ( -5.885917553499152355, 77.12042444889114279, 1.524000000000003352 ) ) ;
#33413=CARTESIAN_POINT ( 'NONE',  ( -57.83161538119274070, 0.8690275533227826976, 1.064493502049185025 ) ) ;
#33414=CARTESIAN_POINT ( 'NONE',  ( -47.91671457320775573, 24.98613645765719582, 0.3547230740385100556 ) ) ;
#33416=B_SPLINE_CURVE_WITH_KNOTS ( 'NONE', 3,
 ( #27863, #24878, #40665, #5310, #33855, #21245, #28070, #37875, #21660, #21042 ),
 .UNSPECIFIED., .F., .F.,
 ( 4, 2, 2, 2, 4 ),
 ( 1.502521540412022121E-05, 0.0001716267095962864064, 0.0003282282037884526001, 0.0004848296979806188210, 0.0006414311921727849876 ),
 .UNSPECIFIED. ) ;
#33417=CARTESIAN_POINT ( 'NONE',  ( -53.83456308493991571, 9.379524109395250164, 3.755176697756422044 ) ) ;
#33418=CARTESIAN_POINT ( 'NONE',  ( -58.45888099891715228, 0.06908990101018230856, 0.7635323682102057585 ) ) ;
#33423=ORIENTED_EDGE ( 'NONE', *, *, #22462, .F. ) ;
#33424=CARTESIAN_POINT ( 'NONE',  ( -41.97746338594183868, 23.60773098774231826, 1.523999999999994026 ) ) ;
#33425=EDGE_CURVE ( 'NONE', #30178, #27616, #9385, .T. ) ;
#33437=CARTESIAN_POINT ( 'NONE',  ( -43.33782384755379269, 21.60941887711892306, 2.445739413452193478 ) ) ;
#33440=CARTESIAN_POINT ( 'NONE',  ( -17.14500000000466784, 71.11999999999886768, -1.270000000000000684 ) ) ;
#33449=CARTESIAN_POINT ( 'NONE',  ( -49.96466797210978683, 13.31430344189337589, 0.7651684107024910864 ) ) ;
#33458=TOROIDAL_SURFACE ( 'NONE', #27324, 0.7620000000000000107, 0.2540000000000000036 ) ;
#33462=EDGE_LOOP ( 'NONE', ( #6419, #37046, #5035, #32591, #34638, #27435 ) ) ;
#33467=DIRECTION ( 'NONE',  ( -0.8745520943968240202, 0.4849315768086551737, -5.361993529360572958E-16 ) ) ;
#33470=CARTESIAN_POINT ( 'NONE',  ( -41.05189575270519242, 23.09451173561980042, -1.270000000000005125 ) ) ;
#33475=ORIENTED_EDGE ( 'NONE', *, *, #5549, .F. ) ;
#33482=CIRCLE ( 'NONE', #15088, 0.6350000000000014522 ) ;
#33484=EDGE_CURVE ( 'NONE', #41561, #18870, #9929, .T. ) ;
#33491=DIRECTION ( 'NONE',  ( -5.188838149069472160E-16, 1.699382548006136559E-16, 1.000000000000000000 ) ) ;
#33498=CARTESIAN_POINT ( 'NONE',  ( -58.35999251409288036, -0.2710268728051273834, -0.1245515173812772602 ) ) ;
#33501=CARTESIAN_POINT ( 'NONE',  ( -6.194847070882102180, 64.72978607931611350, -1.523999999999994026 ) ) ;
#33502=TOROIDAL_SURFACE ( 'NONE', #20544, 0.3810000000000001719, 0.2540000000000000036 ) ;
#33508=VERTEX_POINT ( 'NONE', #12163 ) ;
#33512=CARTESIAN_POINT ( 'NONE',  ( -58.36915991843477514, -0.2902476589043412325, 0.03232548579181320630 ) ) ;
#33519=AXIS2_PLACEMENT_3D ( 'NONE', #6424, #5604, #32402 ) ;
#33520=ADVANCED_FACE ( 'NONE', ( #12380 ), #35373, .T. ) ;
#33521=( BOUNDED_SURFACE ( )  B_SPLINE_SURFACE ( 3, 2, ( 
 ( #5928, #41917, #41705 ),
 ( #2938, #14385, #33173 ),
 ( #19945, #10782, #26980 ),
 ( #29755, #17172, #23976 ) ),
 .UNSPECIFIED., .F., .F., .T. ) 
 B_SPLINE_SURFACE_WITH_KNOTS ( ( 4, 4 ),
 ( 3, 3 ),
 ( 8.673617379884035472E-19, 6.346505048319266184E-05 ),
 ( 0.000000000000000000, 1.000000000000000000 ),
 .UNSPECIFIED. ) 
 GEOMETRIC_REPRESENTATION_ITEM ( )  RATIONAL_B_SPLINE_SURFACE ( (
 ( 1.000000000000000000, 0.7071067811865690000, 1.000000000000000000),
 ( 1.000000000000000000, 0.7071067753522035648, 1.000000000000000000),
 ( 1.000000000000000000, 0.7071464246557217503, 1.000000000000000000),
 ( 1.000000000000000000, 0.7072256012392765800, 1.000000000000000000) ) ) 
 REPRESENTATION_ITEM ( '' )  SURFACE ( )  );
#33522=CARTESIAN_POINT ( 'NONE',  ( -56.39145920764457287, 3.696195836928164891, -1.449839391286715573 ) ) ;
#33525=CARTESIAN_POINT ( 'NONE',  ( -46.94649113550044461, 25.08650387525446845, -1.922972035666928203 ) ) ;
#33526=FACE_OUTER_BOUND ( 'NONE', #34207, .T. ) ;
#33527=CARTESIAN_POINT ( 'NONE',  ( -30.55042969390685315, 56.28656473939154381, -1.270000000000100160 ) ) ;
#33532=CARTESIAN_POINT ( 'NONE',  ( -58.70413935429054675, 0.2332485698458008905, 0.6626129746612758886 ) ) ;
#33536=CARTESIAN_POINT ( 'NONE',  ( -57.78866059769681129, 2.451738602565561642, -1.593934435026652219 ) ) ;
#33538=ORIENTED_EDGE ( 'NONE', *, *, #8613, .F. ) ;
#33539=CARTESIAN_POINT ( 'NONE',  ( -45.03191848990922352, 21.16108440571266414, -3.788620003469220343 ) ) ;
#33544=CIRCLE ( 'NONE', #38279, 0.2539999999999981717 ) ;
#33548=CARTESIAN_POINT ( 'NONE',  ( -29.35823734812138852, 61.32503332634691873, 1.269999999999994245 ) ) ;
#33555=CARTESIAN_POINT ( 'NONE',  ( -58.13670558675570987, 0.2084532747741471848, -0.6632339434594649585 ) ) ;
#33560=CARTESIAN_POINT ( 'NONE',  ( -46.20552558087364758, 24.41938074005533466, -2.020549794458512682 ) ) ;
#33561=CIRCLE ( 'NONE', #15155, 0.7620000000000015650 ) ;
#33570=CARTESIAN_POINT ( 'NONE',  ( -54.34142964503966056, 9.837102586603037935, -3.694930414371515148 ) ) ;
#33579=LINE ( 'NONE', #1208, #2960 ) ;
#33581=CARTESIAN_POINT ( 'NONE',  ( -58.20750686534850615, 0.04498437427168100466, 0.4973296020553291119 ) ) ;
#33582=ADVANCED_FACE ( 'NONE', ( #15766 ), #19763, .T. ) ;
#33584=EDGE_LOOP ( 'NONE', ( #33792, #20354, #28810, #35563 ) ) ;
#33585=CARTESIAN_POINT ( 'NONE',  ( -46.67361288142431164, 26.04169289900193363, -0.9171659260646428669 ) ) ;
#33587=CARTESIAN_POINT ( 'NONE',  ( -17.14500000000466784, 71.11999999999886768, -1.524000000000000909 ) ) ;
#33588=DIRECTION ( 'NONE',  ( -0.3256999990547775337, -0.9454731675810359448, 0.000000000000000000 ) ) ;
#33594=EDGE_LOOP ( 'NONE', ( #33325, #24053, #20848, #37898 ) ) ;
#33603=CARTESIAN_POINT ( 'NONE',  ( -57.99063839910062512, 1.082714195263373425, -1.370926835928584664 ) ) ;
#33608=VERTEX_POINT ( 'NONE', #22430 ) ;
#33610=AXIS2_PLACEMENT_3D ( 'NONE', #16473, #32677, #35250 ) ;
#33613=TOROIDAL_SURFACE ( 'NONE', #13860, 0.7620000000000000107, 0.2540000000000000036 ) ;
#33618=CIRCLE ( 'NONE', #32926, 0.6350000000000014522 ) ;
#33620=PLANE ( 'NONE',  #32081 ) ;
#33625=EDGE_CURVE ( 'NONE', #27874, #14494, #23535, .T. ) ;
#33629=CARTESIAN_POINT ( 'NONE',  ( -56.15333643087780047, 4.440440768670265825, 2.369795045322684590 ) ) ;
#33630=CARTESIAN_POINT ( 'NONE',  ( -48.26009918843825375, 20.16784055841990764, 4.711418872450271245 ) ) ;
#33631=CARTESIAN_POINT ( 'NONE',  ( -57.97566020452313040, 1.918554019021911916, 1.632400077439698061 ) ) ;
#33632=CARTESIAN_POINT ( 'NONE',  ( -58.63629444759789777, -0.3008185210916128893, 0.3590172183976028664 ) ) ;
#33637=CARTESIAN_POINT ( 'NONE',  ( -43.83556092231052048, 21.45200552150719631, 2.811646013901242025 ) ) ;
#33647=DIRECTION ( 'NONE',  ( -5.188838149069472160E-16, 1.699382548006136559E-16, 1.000000000000000000 ) ) ;
#33653=LINE ( 'NONE', #27658, #4998 ) ;
#33659=ORIENTED_EDGE ( 'NONE', *, *, #7627, .T. ) ;
#33660=CARTESIAN_POINT ( 'NONE',  ( -51.51920269172890698, 12.50394502492935978, 2.730133853924309850 ) ) ;
#33664=EDGE_CURVE ( 'NONE', #26949, #28714, #19464, .T. ) ;
#33671=CARTESIAN_POINT ( 'NONE',  ( -18.83202234259777441, 80.34319284215894186, 1.523999999999995358 ) ) ;
#33674=ORIENTED_EDGE ( 'NONE', *, *, #13078, .F. ) ;
#33677=DIRECTION ( 'NONE',  ( -0.1906721105965039909, 0.9816537812491094028, -2.657572025465702696E-16 ) ) ;
#33679=DIRECTION ( 'NONE',  ( -0.8745520943968243532, 0.4849315768086547296, -5.361993529360573944E-16 ) ) ;
#33681=DIRECTION ( 'NONE',  ( -5.188838149069471174E-16, 1.699382548006136313E-16, 1.000000000000000000 ) ) ;
#33691=DIRECTION ( 'NONE',  ( 0.9816537812491126225, 0.1906721105964872265, 8.537024980200846470E-16 ) ) ;
#33694=LINE ( 'NONE', #7912, #30568 ) ;
#33695=CARTESIAN_POINT ( 'NONE',  ( -5.684927786827005392, 65.51297084251929448, 1.524000000000005572 ) ) ;
#33699=ADVANCED_FACE ( 'NONE', ( #9467 ), #15363, .T. ) ;
#33702=DIRECTION ( 'NONE',  ( 0.7517731442105899387, -0.6594218222380295868, -3.321276712443281495E-16 ) ) ;
#33709=EDGE_CURVE ( 'NONE', #17866, #36699, #37800, .T. ) ;
#33713=( NAMED_UNIT ( * ) SI_UNIT ( $, .STERADIAN. ) SOLID_ANGLE_UNIT ( ) );
#33715=CARTESIAN_POINT ( 'NONE',  ( -46.04356016636307203, 20.98312584903309386, 4.505114195460657278 ) ) ;
#33721=ORIENTED_EDGE ( 'NONE', *, *, #4742, .T. ) ;
#33726=CARTESIAN_POINT ( 'NONE',  ( -58.01460528358251878, 0.4727233027791988285, 0.8404818439586951850 ) ) ;
#33734=CARTESIAN_POINT ( 'NONE',  ( -8.576171974424218192, 74.02775907367175989, -1.523999999999996913 ) ) ;
#33735=CARTESIAN_POINT ( 'NONE',  ( -56.42856387642239469, 3.193865871111076338, -9.978765949893178940E-15 ) ) ;
#33737=DIRECTION ( 'NONE',  ( -5.188838149069471174E-16, 1.699382548006136313E-16, 1.000000000000000000 ) ) ;
#33740=CARTESIAN_POINT ( 'NONE',  ( -9.712308604790303335, 65.53852105402241079, 1.524000000000003352 ) ) ;
#33742=CARTESIAN_POINT ( 'NONE',  ( -23.91048590848665967, 81.84235438443283783, 1.269999999999992912 ) ) ;
#33743=LINE ( 'NONE', #7542, #38893 ) ;
#33744=CARTESIAN_POINT ( 'NONE',  ( -58.83227707057486811, -0.08366279997995551554, -1.533110566128066119E-14 ) ) ;
#33745=DIRECTION ( 'NONE',  ( 0.5149185422762213582, -0.8572391118119444542, -8.916573780366528208E-15 ) ) ;
#33748=CARTESIAN_POINT ( 'NONE',  ( -56.90590057130552282, 4.418898835881354792, -2.427662546266534438 ) ) ;
#33751=CARTESIAN_POINT ( 'NONE',  ( -47.61073963480660609, 19.67761866751718713, -5.209507068503004490 ) ) ;
#33759=CARTESIAN_POINT ( 'NONE',  ( -52.42485476335930628, 12.17260451344640693, -4.286044700273143881 ) ) ;
#33762=CIRCLE ( 'NONE', #11998, 0.2539999999999931202 ) ;
#33765=CARTESIAN_POINT ( 'NONE',  ( -57.60835131062518855, 1.351182788547599545, -1.295948770129724315 ) ) ;
#33769=CARTESIAN_POINT ( 'NONE',  ( -48.08949201794742123, 19.91830422262442468, -5.194343260851647770 ) ) ;
#33770=CARTESIAN_POINT ( 'NONE',  ( -8.519412162535127564, 69.40335734044576554, 1.270000000000003348 ) ) ;
#33772=DIRECTION ( 'NONE',  ( -0.4849315768086451817, -0.8745520943968297933, 3.311806702191035794E-15 ) ) ;
#33773=ORIENTED_EDGE ( 'NONE', *, *, #10577, .F. ) ;
#33776=CARTESIAN_POINT ( 'NONE',  ( -19.86616884172038766, 72.62886460123898758, 1.269999999999996687 ) ) ;
#33778=EDGE_CURVE ( 'NONE', #41143, #10068, #33762, .T. ) ;
#33779=CARTESIAN_POINT ( 'NONE',  ( -52.30895062419047292, 13.66434875625866674, -4.401212925246500873 ) ) ;
#33786=AXIS2_PLACEMENT_3D ( 'NONE', #10296, #10919, #30304 ) ;
#33788=CARTESIAN_POINT ( 'NONE',  ( -41.23752580366539888, 23.26788267949599742, -1.524000000000005128 ) ) ;
#33790=CARTESIAN_POINT ( 'NONE',  ( -57.84361080044246251, 0.8513586351276830611, 1.093731309501891458 ) ) ;
#33792=ORIENTED_EDGE ( 'NONE', *, *, #32083, .T. ) ;
#33793=CARTESIAN_POINT ( 'NONE',  ( -46.93986413309943373, 25.37947832266650039, -1.074976477481977222 ) ) ;
#33795=CARTESIAN_POINT ( 'NONE',  ( -46.81030548986653628, 25.80411194895076221, -1.573461678945251130 ) ) ;
#33806=LINE ( 'NONE', #11206, #3922 ) ;
#33807=CARTESIAN_POINT ( 'NONE',  ( -36.79765817521327165, 27.64956762128696610, -1.524000000000003574 ) ) ;
#33808=EDGE_LOOP ( 'NONE', ( #25431, #36592, #15813, #29113 ) ) ;
#33812=CARTESIAN_POINT ( 'NONE',  ( -49.24775882307794461, 17.43196194297031454, -5.046047204416971965 ) ) ;
#33817=VERTEX_POINT ( 'NONE', #18398 ) ;
#33818=AXIS2_PLACEMENT_3D ( 'NONE', #18778, #9216, #32626 ) ;
#33821=CARTESIAN_POINT ( 'NONE',  ( -25.83700401581416628, 71.09321415394998667, 1.523999999999994026 ) ) ;
#33823=ORIENTED_EDGE ( 'NONE', *, *, #30517, .T. ) ;
#33825=DIRECTION ( 'NONE',  ( -0.1565721916417935344, -0.9876665170007969952, 8.659954811668054921E-17 ) ) ;
#33826=CARTESIAN_POINT ( 'NONE',  ( -29.14852920558610450, 63.08767140637714022, -1.270000000000006013 ) ) ;
#33828=AXIS2_PLACEMENT_3D ( 'NONE', #21975, #15382, #37343 ) ;
#33832=CARTESIAN_POINT ( 'NONE',  ( -18.83202234259777086, 80.34319284215895607, -1.270000000000003126 ) ) ;
#33835=CARTESIAN_POINT ( 'NONE',  ( -57.58811225465035477, 1.394777090889576909, 1.315424955976544297 ) ) ;
#33837=CARTESIAN_POINT ( 'NONE',  ( -57.00508801794419611, 2.691366720778187727, 1.977812201481533583 ) ) ;
#33838=CARTESIAN_POINT ( 'NONE',  ( -58.61692577976591423, -0.2667954925353184237, 0.4132871861646182365 ) ) ;
#33843=CARTESIAN_POINT ( 'NONE',  ( -46.07906060731711761, 24.80782705053048076, 1.769089518195985367 ) ) ;
#33848=SURFACE_STYLE_USAGE ( .BOTH. , #37043 ) ;
#33850=ORIENTED_EDGE ( 'NONE', *, *, #30501, .T. ) ;
#33855=CARTESIAN_POINT ( 'NONE',  ( -48.02918200001371218, 19.49203439357020429, 5.381710552009359994 ) ) ;
#33865=AXIS2_PLACEMENT_3D ( 'NONE', #16022, #33078, #29450 ) ;
#33868=CARTESIAN_POINT ( 'NONE',  ( -48.50421218116022004, 14.67712143704007133, 0.4105607596417898408 ) ) ;
#33873=ORIENTED_EDGE ( 'NONE', *, *, #28977, .T. ) ;
#33876=EDGE_CURVE ( 'NONE', #41261, #27727, #31619, .T. ) ;
#33896=DIRECTION ( 'NONE',  ( 0.6294287539884060312, 0.7770581983690815209, 1.945484789722797568E-16 ) ) ;
#33902=CARTESIAN_POINT ( 'NONE',  ( -28.65049350906917880, 77.81814547195517662, -1.524000000000008015 ) ) ;
#33905=EDGE_CURVE ( 'NONE', #25505, #31858, #20798, .T. ) ;
#33909=EDGE_LOOP ( 'NONE', ( #6917, #17663, #15823, #12643 ) ) ;
#33914=VERTEX_POINT ( 'NONE', #1621 ) ;
#33915=ORIENTED_EDGE ( 'NONE', *, *, #4507, .T. ) ;
#33919=CARTESIAN_POINT ( 'NONE',  ( -42.38674052981945550, 22.29968528929560989, 1.779698276446733507 ) ) ;
#33923=CARTESIAN_POINT ( 'NONE',  ( -11.24191166894635074, 82.34025985790688651, -1.523999999999999799 ) ) ;
#33924=ORIENTED_EDGE ( 'NONE', *, *, #2760, .F. ) ;
#33933=CARTESIAN_POINT ( 'NONE',  ( -57.40739589891827421, 2.334961046639910442, 1.895125133209311308 ) ) ;
#33942=CARTESIAN_POINT ( 'NONE',  ( -56.90807066679607829, 2.849439543264234320, -1.873271221587442081 ) ) ;
#33944=FACE_OUTER_BOUND ( 'NONE', #17247, .T. ) ;
#33945=DIRECTION ( 'NONE',  ( 5.188838149069472160E-16, -1.699382548006136559E-16, -1.000000000000000000 ) ) ;
#33950=CARTESIAN_POINT ( 'NONE',  ( -23.43300365160793319, 82.12916405548841681, 1.269999999999993134 ) ) ;
#33951=CARTESIAN_POINT ( 'NONE',  ( -58.18408008067591197, 1.689533369873860824, 0.1826487275623747131 ) ) ;
#33952=EDGE_CURVE ( 'NONE', #10652, #7720, #37154, .T. ) ;
#33955=ORIENTED_EDGE ( 'NONE', *, *, #19071, .T. ) ;
#33956=CARTESIAN_POINT ( 'NONE',  ( -56.01560174880540188, 6.374421267034191985, -2.942705720416971094 ) ) ;
#33957=EDGE_CURVE ( 'NONE', #30054, #20091, #27787, .T. ) ;
#33959=VERTEX_POINT ( 'NONE', #17774 ) ;
#33960=CARTESIAN_POINT ( 'NONE',  ( -44.75127360237845409, 21.22985803518790604, -3.557274316436290995 ) ) ;
#33964=EDGE_CURVE ( 'NONE', #28056, #37511, #38314, .T. ) ;
#33966=CARTESIAN_POINT ( 'NONE',  ( -29.88361747175496319, 69.13349703878448338, 1.269999999999992024 ) ) ;
#33968=CARTESIAN_POINT ( 'NONE',  ( -49.52080500732375867, 17.04929614760187917, -5.023366860225153552 ) ) ;
#33969=ORIENTED_EDGE ( 'NONE', *, *, #13568, .F. ) ;
#33972=CARTESIAN_POINT ( 'NONE',  ( -55.84895358435638713, 5.076860723676236198, -2.553460122158255796 ) ) ;
#33975=CARTESIAN_POINT ( 'NONE',  ( -45.82931853585289872, 22.14969803457954356, -3.600065900675656128 ) ) ;
#33983=CARTESIAN_POINT ( 'NONE',  ( -56.04137470801128273, 5.508142037592367757, -2.879222540163135058 ) ) ;
#33986=CARTESIAN_POINT ( 'NONE',  ( -28.42835727709238114, 77.69497285144578314, 1.523999999999991806 ) ) ;
#33988=CIRCLE ( 'NONE', #12205, 0.5080000000000004512 ) ;
#33993=EDGE_CURVE ( 'NONE', #14172, #537, #35667, .T. ) ;
#33994=CARTESIAN_POINT ( 'NONE',  ( -46.47694366848682535, 20.52739116796101726, -4.723822614978507417 ) ) ;
#33996=CARTESIAN_POINT ( 'NONE',  ( -57.70855261479918141, 1.142328357490882240, 1.228565355105990298 ) ) ;
#33998=ORIENTED_EDGE ( 'NONE', *, *, #37840, .F. ) ;
#33999=CARTESIAN_POINT ( 'NONE',  ( -48.05877817626803505, 25.10121868647436472, -9.935001874592197936E-15 ) ) ;
#34002=ORIENTED_EDGE ( 'NONE', *, *, #39644, .F. ) ;
#34007=LINE ( 'NONE', #38033, #34265 ) ;
#34009=EDGE_CURVE ( 'NONE', #28646, #3540, #32038, .T. ) ;
#34011=ORIENTED_EDGE ( 'NONE', *, *, #3872, .F. ) ;
#34015=CARTESIAN_POINT ( 'NONE',  ( -41.61051026975745515, 22.90141404205858677, -1.547907765227501953 ) ) ;
#34017=ORIENTED_EDGE ( 'NONE', *, *, #34061, .F. ) ;
#34019=ADVANCED_FACE ( 'NONE', ( #12654 ), #2667, .T. ) ;
#34020=ORIENTED_EDGE ( 'NONE', *, *, #9989, .F. ) ;
#34024=CARTESIAN_POINT ( 'NONE',  ( -58.78565887484196395, -0.2971860671469456205, -0.1726678976672988974 ) ) ;
#34032=CARTESIAN_POINT ( 'NONE',  ( -6.401666570281882684, 64.12941061790216679, -1.269999999999994023 ) ) ;
#34044=CARTESIAN_POINT ( 'NONE',  ( -56.13560805112248175, 4.477488644328690981, 2.380442300579769910 ) ) ;
#34045=CARTESIAN_POINT ( 'NONE',  ( -27.88833342972739970, 78.11058938209563962, -1.270000000000007345 ) ) ;
#34046=CARTESIAN_POINT ( 'NONE',  ( -57.29531047346088712, 2.067549486662559222, 1.749273462387482603 ) ) ;
#34047=CARTESIAN_POINT ( 'NONE',  ( -57.66714133758789274, 1.778435395999748536, 1.675315631185262166 ) ) ;
#34052=CARTESIAN_POINT ( 'NONE',  ( -51.58367816905025194, 14.91232437457545146, 4.609044670965822377 ) ) ;
#34058=( NAMED_UNIT ( * ) PLANE_ANGLE_UNIT ( ) SI_UNIT ( $, .RADIAN. ) );
#34059=VECTOR ( 'NONE', #3907, 1000.000000000000000 ) ;
#34061=EDGE_CURVE ( 'NONE', #23452, #29626, #9269, .T. ) ;
#34062=ORIENTED_EDGE ( 'NONE', *, *, #26384, .F. ) ;
#34066=CARTESIAN_POINT ( 'NONE',  ( -47.84356795211436264, 19.38525671449518128, 5.197506975154978726 ) ) ;
#34074=AXIS2_PLACEMENT_3D ( 'NONE', #2820, #22363, #35388 ) ;
#34079=ORIENTED_EDGE ( 'NONE', *, *, #18274, .F. ) ;
#34080=CARTESIAN_POINT ( 'NONE',  ( -48.96835380800505533, 15.76965437727898056, 2.261121166259635107 ) ) ;
#34089=ORIENTED_EDGE ( 'NONE', *, *, #33091, .T. ) ;
#34092=DIRECTION ( 'NONE',  ( -0.9816537812491095139, -0.1906721105965040186, -4.769617732184484037E-16 ) ) ;
#34093=AXIS2_PLACEMENT_3D ( 'NONE', #41715, #1899, #21450 ) ;
#34096=CARTESIAN_POINT ( 'NONE',  ( -10.84307050033138786, 78.30450799593342026, 1.524000000000000687 ) ) ;
#34097=CIRCLE ( 'NONE', #6884, 2.285999999999999588 ) ;
#34102=EDGE_LOOP ( 'NONE', ( #1178, #1539, #33773, #32048 ) ) ;
#34111=FACE_OUTER_BOUND ( 'NONE', #16237, .T. ) ;
#34116=ORIENTED_EDGE ( 'NONE', *, *, #14373, .F. ) ;
#34120=AXIS2_PLACEMENT_3D ( 'NONE', #6460, #3271, #79 ) ;
#34123=ORIENTED_EDGE ( 'NONE', *, *, #7190, .T. ) ;
#34124=CARTESIAN_POINT ( 'NONE',  ( -5.861642722916909243, 64.54502714855203749, -1.523999999999993804 ) ) ;
#34127=CARTESIAN_POINT ( 'NONE',  ( -4.394136353581303389, 70.68697878297604120, 1.270000000000005347 ) ) ;
#34132=CARTESIAN_POINT ( 'NONE',  ( -23.69188486464780752, 78.08202335040543574, 1.269999999999993801 ) ) ;
#34136=ORIENTED_EDGE ( 'NONE', *, *, #1643, .F. ) ;
#34140=CARTESIAN_POINT ( 'NONE',  ( -55.81791661756895451, 5.217579515125359002, 2.786573170145867806 ) ) ;
#34145=AXIS2_PLACEMENT_3D ( 'NONE', #39386, #41955, #41750 ) ;
#34150=EDGE_CURVE ( 'NONE', #29590, #34241, #4509, .T. ) ;
#34151=CARTESIAN_POINT ( 'NONE',  ( -57.97703582661664967, 0.5002880090035632943, -0.5798895178195351274 ) ) ;
#34153=CARTESIAN_POINT ( 'NONE',  ( -6.422645615570758970, 77.88548590848095898, -1.269999999999996465 ) ) ;
#34154=CARTESIAN_POINT ( 'NONE',  ( -20.21600168833980149, 80.16988503754176065, 1.269999999999995355 ) ) ;
#34156=CARTESIAN_POINT ( 'NONE',  ( -8.095114962461808616, 74.19100168833409725, -1.523999999999996691 ) ) ;
#34162=CARTESIAN_POINT ( 'NONE',  ( -5.809227842914839179, 77.60418761620948658, 1.270000000000003126 ) ) ;
#34164=EDGE_LOOP ( 'NONE', ( #15451, #13814, #11251, #27924, #1801 ) ) ;
#34165=CARTESIAN_POINT ( 'NONE',  ( -58.18408008067591197, 1.689533369873860824, -0.1826487275623958351 ) ) ;
#34167=CARTESIAN_POINT ( 'NONE',  ( -44.26155013454958720, 21.23036713625713290, -2.970720547513511889 ) ) ;
#34174=CARTESIAN_POINT ( 'NONE',  ( -49.53032856719786992, 17.03460727780356265, -5.021522771277230568 ) ) ;
#34176=EDGE_LOOP ( 'NONE', ( #2982, #9603, #21099, #29440 ) ) ;
#34177=DIRECTION ( 'NONE',  ( -5.188838149069471174E-16, 1.699382548006136313E-16, 1.000000000000000000 ) ) ;
#34183=CARTESIAN_POINT ( 'NONE',  ( -44.55074271434504851, 21.27721161058206789, -3.389857510897070547 ) ) ;
#34186=EDGE_CURVE ( 'NONE', #19839, #27753, #20137, .T. ) ;
#34187=EDGE_LOOP ( 'NONE', ( #17948, #31250, #19709, #28033 ) ) ;
#34191=EDGE_CURVE ( 'NONE', #30888, #31300, #29255, .T. ) ;
#34192=CARTESIAN_POINT ( 'NONE',  ( -57.22363667057550884, 2.289652018204080264, -1.875138655370660379 ) ) ;
#34193=AXIS2_PLACEMENT_3D ( 'NONE', #995, #4610, #27578 ) ;
#34196=DIRECTION ( 'NONE',  ( 5.188838149069472160E-16, -1.699382548006136559E-16, -1.000000000000000000 ) ) ;
#34202=CARTESIAN_POINT ( 'NONE',  ( -43.02406770836220318, 21.15087974136648086, -0.6363192884524098147 ) ) ;
#34204=CARTESIAN_POINT ( 'NONE',  ( -57.82296528090891030, 0.8544030886276504644, 0.9114307699690248343 ) ) ;
#34205=CARTESIAN_POINT ( 'NONE',  ( -51.38196307026375820, 20.99359797579823805, -9.826526185745439485E-15 ) ) ;
#34207=EDGE_LOOP ( 'NONE', ( #34412, #16860, #25983, #41611 ) ) ;
#34208=CARTESIAN_POINT ( 'NONE',  ( -49.93085365557847410, 21.08514737284949803, -1.613137678015130305 ) ) ;
#34221=CARTESIAN_POINT ( 'NONE',  ( -20.59944062528794362, 79.83666051618703818, -1.270000000000004015 ) ) ;
#34224=CARTESIAN_POINT ( 'NONE',  ( -8.594951744493888768, 74.76616009375631222, 1.270000000000002238 ) ) ;
#34225=EDGE_LOOP ( 'NONE', ( #7162, #37237, #29862, #16820 ) ) ;
#34227=CARTESIAN_POINT ( 'NONE',  ( -28.09515292912719175, 77.51021392068167870, -1.524000000000007571 ) ) ;
#34229=CARTESIAN_POINT ( 'NONE',  ( -57.69387532515962391, 1.166760082113346808, -1.211409762388148792 ) ) ;
#34237=EDGE_CURVE ( 'NONE', #21262, #33817, #9456, .T. ) ;
#34239=AXIS2_PLACEMENT_3D ( 'NONE', #9634, #35633, #32428 ) ;
#34241=VERTEX_POINT ( 'NONE', #19245 ) ;
#34244=EDGE_CURVE ( 'NONE', #8945, #28854, #12700, .T. ) ;
#34246=CIRCLE ( 'NONE', #13837, 0.3810000000000032250 ) ;
#34248=EDGE_CURVE ( 'NONE', #18759, #31609, #12021, .T. ) ;
#34254=EDGE_CURVE ( 'NONE', #30484, #22227, #39068, .T. ) ;
#34255=CARTESIAN_POINT ( 'NONE',  ( -58.36799900954421361, -0.2878193565351589989, 0.05096520709193082949 ) ) ;
#34256=CARTESIAN_POINT ( 'NONE',  ( -28.89366501109621410, 63.08038031665430623, -1.524000000000005350 ) ) ;
#34257=CARTESIAN_POINT ( 'NONE',  ( -52.24107345384238954, 12.50354915519380583, 4.344814160204590436 ) ) ;
#34261=ORIENTED_EDGE ( 'NONE', *, *, #36293, .T. ) ;
#34262=CARTESIAN_POINT ( 'NONE',  ( -51.73272837791831336, 13.19950324185369794, 4.393710239503571202 ) ) ;
#34265=VECTOR ( 'NONE', #24600, 1000.000000000000000 ) ;
#34268=CARTESIAN_POINT ( 'NONE',  ( -24.26619908708081041, 81.70586579672512073, 1.269999999999992912 ) ) ;
#34270=VERTEX_POINT ( 'NONE', #6690 ) ;
#34273=CARTESIAN_POINT ( 'NONE',  ( -8.095114962461808616, 74.19100168833409725, 1.270000000000002460 ) ) ;
#34274=CARTESIAN_POINT ( 'NONE',  ( -43.44488126592214883, 21.78892034651229181, 2.392822157539306271 ) ) ;
#34288=CARTESIAN_POINT ( 'NONE',  ( -47.93564525088159201, 15.36257551998192916, 0.4079155175245546272 ) ) ;
#34293=VERTEX_POINT ( 'NONE', #12236 ) ;
#34303=EDGE_CURVE ( 'NONE', #6455, #4992, #25227, .T. ) ;
#34310=CARTESIAN_POINT ( 'NONE',  ( -41.25198653392084935, 23.25239942703034401, -1.524000000000005128 ) ) ;
#34312=EDGE_LOOP ( 'NONE', ( #19859, #40776, #30689, #31472 ) ) ;
#34329=TOROIDAL_SURFACE ( 'NONE', #15930, 0.3809999999999995057, 0.2540000000000000036 ) ;
#34335=EDGE_LOOP ( 'NONE', ( #17327, #38291, #27046, #21655 ) ) ;
#34343=CARTESIAN_POINT ( 'NONE',  ( -4.377002418771855474, 72.24507371176854065, -1.269999999999994245 ) ) ;
#34349=CARTESIAN_POINT ( 'NONE',  ( -56.42349525705669322, 3.945591430476133255, 2.427201670075267881 ) ) ;
#34357=CARTESIAN_POINT ( 'NONE',  ( -57.68935019796909813, 1.134378438699040759, -1.023808352551158318 ) ) ;
#34359=DIRECTION ( 'NONE',  ( -0.1951894777626611566, -0.9807655518882887336, 0.000000000000000000 ) ) ;
#34360=LINE ( 'NONE', #31149, #36648 ) ;
#34368=CARTESIAN_POINT ( 'NONE',  ( -58.70413935429054675, 0.2332485698458008905, -0.6626129746612970939 ) ) ;
#34369=VERTEX_POINT ( 'NONE', #6902 ) ;
#34370=CARTESIAN_POINT ( 'NONE',  ( -46.78765925927731217, 20.34570826442521962, -4.900687844021752504 ) ) ;
#34377=CARTESIAN_POINT ( 'NONE',  ( -52.67526711997813749, 11.72273190574651913, -4.206385566853321656 ) ) ;
#34378=VERTEX_POINT ( 'NONE', #26484 ) ;
#34382=DIRECTION ( 'NONE',  ( -0.3213437296502684171, 0.9469626219732514283, 0.000000000000000000 ) ) ;
#34385=CARTESIAN_POINT ( 'NONE',  ( -54.97180548219925100, 8.422794459035404913, -3.467293221275798309 ) ) ;
#34387=CIRCLE ( 'NONE', #17354, 9.048749999999998295 ) ;
#34388=ORIENTED_EDGE ( 'NONE', *, *, #41542, .F. ) ;
#34392=EDGE_CURVE ( 'NONE', #12640, #16254, #23264, .T. ) ;
#34393=CARTESIAN_POINT ( 'NONE',  ( -57.24023649071029496, 3.661034843983918208, -2.195083147259570211 ) ) ;
#34396=DIRECTION ( 'NONE',  ( -0.8745520943968223548, 0.4849315768086582268, -6.829619984160691573E-16 ) ) ;
#34400=CARTESIAN_POINT ( 'NONE',  ( -44.22601141000046709, 20.28211486706537414, -1.272444536529930836 ) ) ;
#34401=ORIENTED_EDGE ( 'NONE', *, *, #11859, .T. ) ;
#34404=CARTESIAN_POINT ( 'NONE',  ( -58.22824150656796860, 0.01698906185855497686, 0.5964212723216197887 ) ) ;
#34405=CARTESIAN_POINT ( 'NONE',  ( -51.75204694603132083, 19.49597778360960021, 0.7628839638999955763 ) ) ;
#34409=CARTESIAN_POINT ( 'NONE',  ( -47.91489772873670461, 20.73163290703075745, -4.601312741205012991 ) ) ;
#34412=ORIENTED_EDGE ( 'NONE', *, *, #17757, .T. ) ;
#34413=CARTESIAN_POINT ( 'NONE',  ( -47.84623148323176878, 19.38793950428539503, 5.205198760075354869 ) ) ;
#34423=EDGE_CURVE ( 'NONE', #14494, #18759, #4557, .T. ) ;
#34425=CARTESIAN_POINT ( 'NONE',  ( -41.06677624538381366, 23.07857903911209974, -1.524000000001595856 ) ) ;
#34426=DIRECTION ( 'NONE',  ( 0.5149185422762101449, -0.8572391118119511155, 4.128606161907551211E-16 ) ) ;
#34427=VERTEX_POINT ( 'NONE', #16678 ) ;
#34429=DIRECTION ( 'NONE',  ( -0.8745520943968235761, 0.4849315768086558398, -4.268512490100410909E-16 ) ) ;
#34431=CARTESIAN_POINT ( 'NONE',  ( -54.51629495444830553, 7.799846118215131519, -3.232377281229704025 ) ) ;
#34443=AXIS2_PLACEMENT_3D ( 'NONE', #24036, #18055, #8275 ) ;
#34458=CARTESIAN_POINT ( 'NONE',  ( -57.96289673749877380, 0.5850535986806209010, 0.9075947480399308986 ) ) ;
#34464=EDGE_CURVE ( 'NONE', #30173, #30054, #31729, .T. ) ;
#34465=CARTESIAN_POINT ( 'NONE',  ( -49.59816314059867182, 17.91649583374774224, 5.069000701391649599 ) ) ;
#34470=DIRECTION ( 'NONE',  ( 0.9336303900108928744, 0.3582377630123714241, 0.000000000000000000 ) ) ;
#34474=CARTESIAN_POINT ( 'NONE',  ( -30.59449053071180558, 55.40488188707849559, 1.523999999999994692 ) ) ;
#34475=FACE_OUTER_BOUND ( 'NONE', #7817, .T. ) ;
#34477=CIRCLE ( 'NONE', #23571, 0.6350000000000006750 ) ;
#34491=CARTESIAN_POINT ( 'NONE',  ( -54.85284047870325708, 7.073525668766899699, 2.945785012852135676 ) ) ;
#34498=ORIENTED_EDGE ( 'NONE', *, *, #17066, .F. ) ;
#34502=EDGE_CURVE ( 'NONE', #19961, #14753, #40591, .T. ) ;
#34513=DIRECTION ( 'NONE',  ( -0.8745520943968243532, 0.4849315768086547296, -6.829619984160642269E-16 ) ) ;
#34518=ORIENTED_EDGE ( 'NONE', *, *, #26363, .F. ) ;
#34519=ORIENTED_EDGE ( 'NONE', *, *, #11795, .F. ) ;
#34520=DIRECTION ( 'NONE',  ( -5.188838149069471174E-16, 1.699382548006136313E-16, 1.000000000000000000 ) ) ;
#34529=LINE ( 'NONE', #5355, #887 ) ;
#34537=ORIENTED_EDGE ( 'NONE', *, *, #25378, .F. ) ;
#34542=EDGE_CURVE ( 'NONE', #40365, #29748, #33100, .T. ) ;
#34544=ORIENTED_EDGE ( 'NONE', *, *, #30250, .F. ) ;
#34546=DIRECTION ( 'NONE',  ( -6.829619984160660610E-15, 0.000000000000000000, -1.000000000000000000 ) ) ;
#34547=CIRCLE ( 'NONE', #20894, 0.2540000000000012248 ) ;
#34550=CARTESIAN_POINT ( 'NONE',  ( -42.24009424636936672, 22.39526031405182849, 1.717801471214081444 ) ) ;
#34554=CARTESIAN_POINT ( 'NONE',  ( -14.53564353655538000, 79.78436006922240153, -1.270000000000000906 ) ) ;
#34555=CARTESIAN_POINT ( 'NONE',  ( -19.15923810799328209, 79.68098548105338352, -1.270000000000003348 ) ) ;
#34560=AXIS2_PLACEMENT_3D ( 'NONE', #36798, #20161, #10380 ) ;
#34561=CARTESIAN_POINT ( 'NONE',  ( -58.63691926681516975, -0.7730888055359085298, 0.03927874230119918209 ) ) ;
#34569=CARTESIAN_POINT ( 'NONE',  ( -56.90438685736649660, 2.765855619508456265, -1.561774844827678033 ) ) ;
#34572=CARTESIAN_POINT ( 'NONE',  ( -17.09698261757901960, 84.43312239790384410, -1.524000000000002908 ) ) ;
#34573=FACE_OUTER_BOUND ( 'NONE', #8423, .T. ) ;
#34576=DIRECTION ( 'NONE',  ( -0.9998501190848635423, -0.01731298258487451447, -5.158639060800523934E-16 ) ) ;
#34581=CARTESIAN_POINT ( 'NONE',  ( -58.76922381231047865, 0.08391971067571446508, -0.07695160083613393487 ) ) ;
#34589=CARTESIAN_POINT ( 'NONE',  ( -52.06727285681002115, 12.81026601648138019, -4.396686699310198954 ) ) ;
#34590=ORIENTED_EDGE ( 'NONE', *, *, #22473, .T. ) ;
#34592=DIRECTION ( 'NONE',  ( 0.8745520943968246863, -0.4849315768086538414, 5.122214988120500191E-16 ) ) ;
#34594=CARTESIAN_POINT ( 'NONE',  ( -57.04684799334965106, 2.555418974455772041, -1.775728233086056873 ) ) ;
#34597=CARTESIAN_POINT ( 'NONE',  ( -50.82551848962686591, 16.13924203555649228, -4.804203053272171786 ) ) ;
#34604=CARTESIAN_POINT ( 'NONE',  ( -58.24002838079472610, 0.001074765447070524793, -0.6562585879479864159 ) ) ;
#34607=DIRECTION ( 'NONE',  ( -0.6594218222380264782, -0.7517731442105928252, -1.663245240604415392E-15 ) ) ;
#34611=CARTESIAN_POINT ( 'NONE',  ( -58.20820809768403592, 1.420579653404085985, -1.355822160094614759 ) ) ;
#34612=AXIS2_PLACEMENT_3D ( 'NONE', #41008, #23590, #16790 ) ;
#34618=CARTESIAN_POINT ( 'NONE',  ( -11.17805678602830355, 77.92260723867444483, -1.523999999999998911 ) ) ;
#34619=CARTESIAN_POINT ( 'NONE',  ( -50.06424591225965059, 20.16147316606144813, 2.291703678227654972 ) ) ;
#34621=ORIENTED_EDGE ( 'NONE', *, *, #311, .T. ) ;
#34622=CARTESIAN_POINT ( 'NONE',  ( -47.99264284736476327, 22.55967899981254376, -2.517363275470477113 ) ) ;
#34630=DIRECTION ( 'NONE',  ( -0.3086833358528130455, 0.9511648638205574269, -1.501066210750425580E-13 ) ) ;
#34636=CARTESIAN_POINT ( 'NONE',  ( -47.23734572760722017, 20.07943206202290298, -5.152903761255795523 ) ) ;
#34637=CARTESIAN_POINT ( 'NONE',  ( -17.64290547347870941, 83.78857423953914463, -1.270000000000003126 ) ) ;
#34638=ORIENTED_EDGE ( 'NONE', *, *, #39902, .T. ) ;
#34654=DIRECTION ( 'NONE',  ( -0.3256999990547876367, -0.9454731675810326141, -8.328397965208553695E-18 ) ) ;
#34655=ORIENTED_EDGE ( 'NONE', *, *, #20890, .T. ) ;
#34657=DIRECTION ( 'NONE',  ( -0.3256999990547836399, -0.9454731675810339464, 0.000000000000000000 ) ) ;
#34665=CARTESIAN_POINT ( 'NONE',  ( -58.33727096013997482, -0.2232939613935198409, 0.2257470585846221012 ) ) ;
#34667=DIRECTION ( 'NONE',  ( 0.1951894777626589361, 0.9807655518882891776, -6.538892540527331846E-17 ) ) ;
#34671=ORIENTED_EDGE ( 'NONE', *, *, #4075, .F. ) ;
#34672=CARTESIAN_POINT ( 'NONE',  ( -47.61549956331938915, 19.66157307908738261, 5.197827534590556908 ) ) ;
#34679=EDGE_CURVE ( 'NONE', #26041, #16908, #15400, .T. ) ;
#34680=VERTEX_POINT ( 'NONE', #13282 ) ;
#34683=DIRECTION ( 'NONE',  ( 0.2883665106726619465, 0.9575201071113199625, 6.014747832865860437E-16 ) ) ;
#34684=CARTESIAN_POINT ( 'NONE',  ( -42.07367843439215704, 22.17357734922920187, 1.489526742669803783 ) ) ;
#34698=CARTESIAN_POINT ( 'NONE',  ( -57.29531047346088712, 2.067549486662559222, 1.749273462387482381 ) ) ;
#34706=ORIENTED_EDGE ( 'NONE', *, *, #21414, .F. ) ;
#34709=DIRECTION ( 'NONE',  ( 0.8572391118119510045, 0.5149185422762100339, 3.573031421855330583E-16 ) ) ;
#34710=EDGE_CURVE ( 'NONE', #18324, #19839, #34477, .T. ) ;
#34714=DIRECTION ( 'NONE',  ( -0.8745520943968347893, 0.4849315768086356893, -6.829619984160681712E-16 ) ) ;
#34715=EDGE_CURVE ( 'NONE', #27671, #22599, #28638, .T. ) ;
#34718=DIRECTION ( 'NONE',  ( -5.188838149069472160E-16, 1.699382548006136559E-16, 1.000000000000000000 ) ) ;
#34721=ORIENTED_EDGE ( 'NONE', *, *, #20371, .T. ) ;
#34722=CYLINDRICAL_SURFACE ( 'NONE', #23410, 0.2540000000000031677 ) ;
#34740=ORIENTED_EDGE ( 'NONE', *, *, #27268, .T. ) ;
#34756=LINE ( 'NONE', #5591, #29036 ) ;
#34757=VECTOR ( 'NONE', #27037, 1000.000000000000114 ) ;
#34764=DIRECTION ( 'NONE',  ( 0.9454731675810332803, -0.3256999990547855828, 8.537024980200802097E-16 ) ) ;
#34766=VECTOR ( 'NONE', #34709, 1000.000000000000114 ) ;
#34768=CARTESIAN_POINT ( 'NONE',  ( -57.79860935920279275, 1.496589803099593219, 1.561213607911194901 ) ) ;
#34777=CARTESIAN_POINT ( 'NONE',  ( -57.82296528090891030, 0.8544030886276504644, -0.9114307699690453735 ) ) ;
#34780=CARTESIAN_POINT ( 'NONE',  ( -10.75478607932181241, 82.07015292912137738, 1.269999999999999796 ) ) ;
#34784=DIRECTION ( 'NONE',  ( -0.8745520943968249084, 0.4849315768086534528, -5.361993529360573944E-16 ) ) ;
#34788=ORIENTED_EDGE ( 'NONE', *, *, #13898, .T. ) ;
#34789=CARTESIAN_POINT ( 'NONE',  ( -58.83227707057485389, -0.08366279997994163775, -5.898546760656774196E-15 ) ) ;
#34791=CARTESIAN_POINT ( 'NONE',  ( -41.34781391883380053, 22.78346824044358954, -1.529410470714712700 ) ) ;
#34792=AXIS2_PLACEMENT_3D ( 'NONE', #41266, #14622, #12287 ) ;
#34799=CARTESIAN_POINT ( 'NONE',  ( -57.92803731934569811, 1.218056268468654002, -1.434962409700567987 ) ) ;
#34800=ORIENTED_EDGE ( 'NONE', *, *, #25087, .F. ) ;
#34802=DIRECTION ( 'NONE',  ( 0.6825627711659328911, 0.7308269722843309113, 2.299753143848213649E-16 ) ) ;
#34806=TOROIDAL_SURFACE ( 'NONE', #19814, 0.3809999999999999498, 0.2540000000000000036 ) ;
#34808=CARTESIAN_POINT ( 'NONE',  ( -56.26318288983030413, 4.268071985104968213, -2.480832006587858185 ) ) ;
#34810=ORIENTED_EDGE ( 'NONE', *, *, #29749, .T. ) ;
#34816=CARTESIAN_POINT ( 'NONE',  ( -58.75009580408200094, 0.1057190229620807997, -0.6617493214611014363 ) ) ;
#34821=EDGE_CURVE ( 'NONE', #27053, #21375, #17988, .T. ) ;
#34825=CARTESIAN_POINT ( 'NONE',  ( -55.60486134785667645, 7.243031971518515633, -3.140198620020504094 ) ) ;
#34826=DIRECTION ( 'NONE',  ( -5.188838149069471174E-16, 1.699382548006136313E-16, 1.000000000000000000 ) ) ;
#34829=DIRECTION ( 'NONE',  ( 0.7308269722843147020, -0.6825627711659504326, 8.537024980200894788E-16 ) ) ;
#34831=CARTESIAN_POINT ( 'NONE',  ( -58.37241122568489970, -0.2962816677228030660, -1.043042736874535760E-14 ) ) ;
#34832=CARTESIAN_POINT ( 'NONE',  ( -49.81807968324856972, 18.07223176367294570, 4.612844822355046226 ) ) ;
#34834=ORIENTED_EDGE ( 'NONE', *, *, #10562, .F. ) ;
#34835=CARTESIAN_POINT ( 'NONE',  ( -49.29989578322635424, 20.38947471906982756, -3.123819567266207464 ) ) ;
#34848=CARTESIAN_POINT ( 'NONE',  ( -10.93398011767285283, 82.89560043784887000, -1.269999999999999352 ) ) ;
#34851=LINE ( 'NONE', #2486, #26330 ) ;
#34862=CIRCLE ( 'NONE', #27372, 0.2539999999999983937 ) ;
#34867=CARTESIAN_POINT ( 'NONE',  ( -46.60530155212503445, 26.17382724835477958, -1.524000000000008459 ) ) ;
#34871=CARTESIAN_POINT ( 'NONE',  ( -27.97106122948731155, 77.87043919753004673, 1.523999999999992028 ) ) ;
#34877=EDGE_CURVE ( 'NONE', #41561, #40395, #32306, .T. ) ;
#34880=CARTESIAN_POINT ( 'NONE',  ( -58.24403404964675701, -0.02353476031055234952, 0.4695906566965602491 ) ) ;
#34881=DIRECTION ( 'NONE',  ( -5.188838149069472160E-16, 1.699382548006136559E-16, 1.000000000000000000 ) ) ;
#34882=DIRECTION ( 'NONE',  ( 0.1565721916418034432, 0.9876665170007953298, -8.659954811667511346E-17 ) ) ;
#34885=DIRECTION ( 'NONE',  ( -0.8745520943968235761, 0.4849315768086558953, -5.361993529360570985E-16 ) ) ;
#34886=ORIENTED_EDGE ( 'NONE', *, *, #26690, .F. ) ;
#34887=CARTESIAN_POINT ( 'NONE',  ( -50.82551848962686591, 16.13924203555649228, 4.804203053272154911 ) ) ;
#34888=( BOUNDED_CURVE ( )  B_SPLINE_CURVE ( 2, ( #16261, #3726, #32468 ),
 .UNSPECIFIED., .F., .T. ) 
 B_SPLINE_CURVE_WITH_KNOTS ( ( 3, 3 ),
 ( 0.000000000000000000, 1.000000000000000000 ),
 .UNSPECIFIED. ) 
 CURVE ( )  GEOMETRIC_REPRESENTATION_ITEM ( )  RATIONAL_B_SPLINE_CURVE ( ( 1.000000000000000000, 0.4190531958282215919, 1.000000000000000000 ) ) 
 REPRESENTATION_ITEM ( '' )  );
#34892=CARTESIAN_POINT ( 'NONE',  ( -29.36432400326824066, 68.35621600878259585, 1.523999999999992916 ) ) ;
#34896=CARTESIAN_POINT ( 'NONE',  ( -29.22020851875563352, 63.09400180735026709, 1.270000000000041540 ) ) ;
#34897=CARTESIAN_POINT ( 'NONE',  ( -3.911441847776591985, 70.75305732235845824, 1.270000000000006235 ) ) ;
#34898=CYLINDRICAL_SURFACE ( 'NONE', #15596, 0.2540000000000052771 ) ;
#34899=CARTESIAN_POINT ( 'NONE',  ( -23.62918761621517305, 82.45577215708875940, -1.270000000000006013 ) ) ;
#34901=DIRECTION ( 'NONE',  ( -0.01731298258488817021, 0.9998501190848633202, 8.235542606122962463E-15 ) ) ;
#34909=CIRCLE ( 'NONE', #16523, 2.857500000000000817 ) ;
#34912=ORIENTED_EDGE ( 'NONE', *, *, #37945, .F. ) ;
#34913=CARTESIAN_POINT ( 'NONE',  ( -55.10067240196883631, 5.634149028679341420, 0.4880682687715845458 ) ) ;
#34915=ADVANCED_FACE ( 'NONE', ( #23113 ), #13132, .F. ) ;
#34921=ORIENTED_EDGE ( 'NONE', *, *, #31930, .T. ) ;
#34923=EDGE_CURVE ( 'NONE', #37655, #8441, #18129, .T. ) ;
#34933=( GEOMETRIC_REPRESENTATION_CONTEXT ( 3 ) GLOBAL_UNCERTAINTY_ASSIGNED_CONTEXT ( ( #15482 ) ) GLOBAL_UNIT_ASSIGNED_CONTEXT ( ( #14434, #34058, #13613 ) ) REPRESENTATION_CONTEXT ( 'NONE', 'WORKASPACE' ) );
#34934=CARTESIAN_POINT ( 'NONE',  ( -46.92362637188625740, 25.23517642483339074, 1.818802264970843519 ) ) ;
#34937=CARTESIAN_POINT ( 'NONE',  ( -46.40591231939538375, 23.70796668624020853, 2.618124260499386402 ) ) ;
#34940=TOROIDAL_SURFACE ( 'NONE', #36314, 8.794749999999996959, 0.2540000000000000036 ) ;
#34943=CARTESIAN_POINT ( 'NONE',  ( -7.772068811996249771, 69.25462295839062676, -1.523999999999995580 ) ) ;
#34949=AXIS2_PLACEMENT_3D ( 'NONE', #21231, #10823, #24018 ) ;
#34951=CARTESIAN_POINT ( 'NONE',  ( -58.83227707057486811, -0.08366279997995551554, -1.529465441686574059E-14 ) ) ;
#34957=CARTESIAN_POINT ( 'NONE',  ( -6.135835944515187101, 77.40800365160224317, -1.523999999999996247 ) ) ;
#34969=DIRECTION ( 'NONE',  ( 0.1565721916417901483, 0.9876665170007974393, 0.000000000000000000 ) ) ;
#34972=LINE ( 'NONE', #21432, #22491 ) ;
#34975=AXIS2_PLACEMENT_3D ( 'NONE', #29958, #20777, #3790 ) ;
#34978=ADVANCED_FACE ( 'NONE', ( #39126 ), #29539, .T. ) ;
#34982=CIRCLE ( 'NONE', #2321, 0.5080000000000000071 ) ;
#34984=FACE_OUTER_BOUND ( 'NONE', #1718, .T. ) ;
#34985=DIRECTION ( 'NONE',  ( 0.1906721105965040186, -0.9816537812491095139, 2.657572025465703189E-16 ) ) ;
#34987=VECTOR ( 'NONE', #22108, 1000.000000000000000 ) ;
#34994=VECTOR ( 'NONE', #6776, 1000.000000000000000 ) ;
#35001=AXIS2_PLACEMENT_3D ( 'NONE', #33130, #23295, #7773 ) ;
#35003=DIRECTION ( 'NONE',  ( 0.7258741224862652608, -0.6878275643682757456, 8.537024980200906621E-16 ) ) ;
#35006=CARTESIAN_POINT ( 'NONE',  ( -41.26650320839694785, 23.23696823412479873, 1.523999999999994248 ) ) ;
#35011=ADVANCED_FACE ( 'NONE', ( #6749 ), #12916, .T. ) ;
#35012=CARTESIAN_POINT ( 'NONE',  ( -58.73915225836899623, 0.1638436772961326948, -0.01855759196812271222 ) ) ;
#35013=EDGE_LOOP ( 'NONE', ( #4109, #30212, #6304, #4881 ) ) ;
#35014=CARTESIAN_POINT ( 'NONE',  ( -41.09676540851936011, 23.04694042099055196, -1.523999999999985588 ) ) ;
#35021=CARTESIAN_POINT ( 'NONE',  ( -58.15941753978571427, 0.7172703587996687169, -1.185050425798436891 ) ) ;
#35024=CYLINDRICAL_SURFACE ( 'NONE', #17508, 2.539999999999996483 ) ;
#35026=CARTESIAN_POINT ( 'NONE',  ( -25.97603047661466036, 74.27059221564131519, 1.523999999999992694 ) ) ;
#35030=CARTESIAN_POINT ( 'NONE',  ( -54.34142964503966056, 9.837102586603037935, -3.694930414371515148 ) ) ;
#35037=CARTESIAN_POINT ( 'NONE',  ( -57.97566020452313040, 1.918554019021911916, -1.632400077439718933 ) ) ;
#35043=DIRECTION ( 'NONE',  ( -0.8572391118119488951, -0.5149185422762135866, 0.000000000000000000 ) ) ;
#35044=CARTESIAN_POINT ( 'NONE',  ( -41.93982928939168175, 22.21638423992008882, -1.241790202385191666 ) ) ;
#35046=CARTESIAN_POINT ( 'NONE',  ( -58.37241122568488549, -0.2962816677227753104, 0.2416009568453807987 ) ) ;
#35047=CARTESIAN_POINT ( 'NONE',  ( -54.13734601216691544, 8.984237177898892313, 3.668503415557924363 ) ) ;
#35050=CARTESIAN_POINT ( 'NONE',  ( -52.46220839783629941, 13.84563717269405458, 4.010158452165631715 ) ) ;
#35051=EDGE_CURVE ( 'NONE', #40169, #19837, #31058, .T. ) ;
#35054=CARTESIAN_POINT ( 'NONE',  ( -47.99025707952956310, 21.67807857130912907, -3.596429695783045055 ) ) ;
#35068=FACE_OUTER_BOUND ( 'NONE', #27385, .T. ) ;
#35069=DIRECTION ( 'NONE',  ( 0.3582377630123915746, -0.9336303900108851028, 3.445432962228667069E-16 ) ) ;
#35070=EDGE_LOOP ( 'NONE', ( #25765, #3947, #3916, #7699 ) ) ;
#35071=AXIS2_PLACEMENT_3D ( 'NONE', #9106, #9872, #10084 ) ;
#35089=CARTESIAN_POINT ( 'NONE',  ( -46.49070643682303938, 25.85670910372597220, -1.524000000000008459 ) ) ;
#35093=AXIS2_PLACEMENT_3D ( 'NONE', #18053, #18258, #18470 ) ;
#35096=CARTESIAN_POINT ( 'NONE',  ( -58.02663847586048718, 0.4467317610142895745, 0.8231150145234874538 ) ) ;
#35100=ORIENTED_EDGE ( 'NONE', *, *, #2127, .F. ) ;
#35104=CARTESIAN_POINT ( 'NONE',  ( -29.22735587826698378, 60.46978361828900006, 1.523999999999993804 ) ) ;
#35110=FACE_OUTER_BOUND ( 'NONE', #19327, .T. ) ;
#35121=VERTEX_POINT ( 'NONE', #20341 ) ;
#35122=CARTESIAN_POINT ( 'NONE',  ( -56.88731995051696089, 2.378615435641953546, 0.1283520312635431648 ) ) ;
#35127=DIRECTION ( 'NONE',  ( 5.188838149069472160E-16, -1.699382548006136559E-16, -1.000000000000000000 ) ) ;
#35137=DIRECTION ( 'NONE',  ( -5.188838149069471174E-16, 1.699382548006136313E-16, 1.000000000000000000 ) ) ;
#35139=CARTESIAN_POINT ( 'NONE',  ( -47.53841933257975683, 25.36174273411122115, 0.2940116119274914785 ) ) ;
#35141=CARTESIAN_POINT ( 'NONE',  ( -48.16508968810062896, 19.01313136326716347, 5.219744232931976313 ) ) ;
#35142=CARTESIAN_POINT ( 'NONE',  ( -41.28107547821692691, 23.22158991241129300, -1.523999999999999355 ) ) ;
#35144=VECTOR ( 'NONE', #525, 1000.000000000000000 ) ;
#35145=ORIENTED_EDGE ( 'NONE', *, *, #26636, .T. ) ;
#35147=DIRECTION ( 'NONE',  ( 5.188838149069472160E-16, -1.699382548006136559E-16, -1.000000000000000000 ) ) ;
#35154=DIRECTION ( 'NONE',  ( 5.188838149069471174E-16, -1.699382548006136313E-16, -1.000000000000000000 ) ) ;
#35162=ORIENTED_EDGE ( 'NONE', *, *, #34542, .T. ) ;
#35167=CIRCLE ( 'NONE', #13207, 0.5080000000000000071 ) ;
#35169=EDGE_CURVE ( 'NONE', #16326, #30173, #7182, .T. ) ;
#35170=ORIENTED_EDGE ( 'NONE', *, *, #34303, .F. ) ;
#35172=DIRECTION ( 'NONE',  ( -0.9876665170007969952, 0.1565721916417935344, -5.390917751951444915E-16 ) ) ;
#35180=DIRECTION ( 'NONE',  ( 5.188838149069472160E-16, -1.699382548006136559E-16, -1.000000000000000000 ) ) ;
#35184=CIRCLE ( 'NONE', #5273, 0.2539999999999997260 ) ;
#35187=FACE_OUTER_BOUND ( 'NONE', #5552, .T. ) ;
#35189=DIRECTION ( 'NONE',  ( -5.188838149069471174E-16, 1.699382548006136313E-16, 1.000000000000000000 ) ) ;
#35195=AXIS2_PLACEMENT_3D ( 'NONE', #16070, #42092, #38258 ) ;
#35215=FACE_OUTER_BOUND ( 'NONE', #6285, .T. ) ;
#35221=CARTESIAN_POINT ( 'NONE',  ( -56.87050244847664260, 3.471200836702969195, -2.275408806060764455 ) ) ;
#35223=CARTESIAN_POINT ( 'NONE',  ( -58.34429324193579447, -0.2380942604817831709, -0.1989150628791391540 ) ) ;
#35227=DIRECTION ( 'NONE',  ( -5.188838149069472160E-16, 1.699382548006136559E-16, 1.000000000000000000 ) ) ;
#35230=CARTESIAN_POINT ( 'NONE',  ( -51.02479983779974049, 14.46739584830851477, -4.600955224801065668 ) ) ;
#35238=FACE_OUTER_BOUND ( 'NONE', #13850, .T. ) ;
#35245=CARTESIAN_POINT ( 'NONE',  ( -25.56614996202194590, 73.65611136973726047, -1.270000000000005569 ) ) ;
#35247=ADVANCED_FACE ( 'NONE', ( #4198 ), #468, .T. ) ;
#35248=CARTESIAN_POINT ( 'NONE',  ( -47.79679003974130325, 17.22715854250130718, -2.282645788202384729 ) ) ;
#35249=CARTESIAN_POINT ( 'NONE',  ( -5.591535794131392123, 65.03215273817657760, -1.523999999999993804 ) ) ;
#35250=DIRECTION ( 'NONE',  ( 0.3582377630123915746, -0.9336303900108851028, 3.445432962228667069E-16 ) ) ;
#35251=CARTESIAN_POINT ( 'NONE',  ( -52.89566005465288612, 11.31963682940546789, 4.132128454502246306 ) ) ;
#35252=EDGE_CURVE ( 'NONE', #19839, #35748, #26761, .T. ) ;
#35254=CARTESIAN_POINT ( 'NONE',  ( -57.93941708942283952, 2.052042089854988483, 1.628789306319508023 ) ) ;
#35257=CARTESIAN_POINT ( 'NONE',  ( -52.70911355518960306, 14.14937146821753444, -3.349573991549135155 ) ) ;
#35260=ORIENTED_EDGE ( 'NONE', *, *, #40233, .F. ) ;
#35265=DIRECTION ( 'NONE',  ( -0.3582377630123966261, 0.9336303900108832154, 0.000000000000000000 ) ) ;
#35271=DIRECTION ( 'NONE',  ( -0.8745520943968243532, 0.4849315768086547296, -5.361993529360573944E-16 ) ) ;
#35275=EDGE_LOOP ( 'NONE', ( #40067, #16665, #8018, #9641 ) ) ;
#35276=CARTESIAN_POINT ( 'NONE',  ( -58.32396914991895898, -0.1951167097209117463, -0.2694727270791387186 ) ) ;
#35286=DIRECTION ( 'NONE',  ( -0.8745520943968235761, 0.4849315768086558398, -5.691349986800547879E-16 ) ) ;
#35287=CARTESIAN_POINT ( 'NONE',  ( -47.43570116002440784, 20.37060963802031566, -5.342502768866047802 ) ) ;
#35289=ORIENTED_EDGE ( 'NONE', *, *, #3821, .T. ) ;
#35300=ADVANCED_FACE ( 'NONE', ( #37799 ), #26998, .T. ) ;
#35302=ADVANCED_FACE ( 'NONE', ( #18831 ), #5869, .F. ) ;
#35303=ORIENTED_EDGE ( 'NONE', *, *, #14638, .T. ) ;
#35307=CARTESIAN_POINT ( 'NONE',  ( -30.15642192025596202, 71.36377005712995469, -1.524000000000007571 ) ) ;
#35311=CARTESIAN_POINT ( 'NONE',  ( -29.20122892408340221, 63.96733531827668173, 1.269999999999945617 ) ) ;
#35316=VECTOR ( 'NONE', #41444, 1000.000000000000000 ) ;
#35319=DIRECTION ( 'NONE',  ( 0.8572391118119481179, 0.5149185422762151410, 0.000000000000000000 ) ) ;
#35328=LINE ( 'NONE', #38734, #34994 ) ;
#35333=DIRECTION ( 'NONE',  ( -0.01731298258488003436, 0.9998501190848634312, 0.000000000000000000 ) ) ;
#35334=DIRECTION ( 'NONE',  ( -0.3582377630123966261, 0.9336303900108832154, 0.000000000000000000 ) ) ;
#35340=DIRECTION ( 'NONE',  ( -0.8745520943968347893, 0.4849315768086356893, -6.829619984160681712E-16 ) ) ;
#35341=CARTESIAN_POINT ( 'NONE',  ( -46.86252819529217106, 25.53111598637714152, 1.612082337883730787 ) ) ;
#35342=CARTESIAN_POINT ( 'NONE',  ( -46.79514595010191158, 25.77136020477034606, 0.9526608576032333797 ) ) ;
#35344=EDGE_CURVE ( 'NONE', #18324, #32986, #9326, .T. ) ;
#35345=CARTESIAN_POINT ( 'NONE',  ( -44.13308345971568514, 24.21351174012166396, 1.567149544246648762 ) ) ;
#35349=DIRECTION ( 'NONE',  ( -0.8745520943968245753, 0.4849315768086539524, -5.691349986800526185E-16 ) ) ;
#35353=CARTESIAN_POINT ( 'NONE',  ( -11.17805678602830355, 77.92260723867444483, 1.269999999999999352 ) ) ;
#35356=DIRECTION ( 'NONE',  ( 0.9454731675810374991, -0.3256999990547734258, 7.420046207093947887E-15 ) ) ;
#35364=ORIENTED_EDGE ( 'NONE', *, *, #35977, .F. ) ;
#35373=CYLINDRICAL_SURFACE ( 'NONE', #28300, 0.6350000000000014522 ) ;
#35386=CARTESIAN_POINT ( 'NONE',  ( -24.32950799593924884, 77.42192949967211746, -1.524000000000005572 ) ) ;
#35387=( BOUNDED_SURFACE ( )  B_SPLINE_SURFACE ( 3, 2, ( 
 ( #12516, #8694, #25082 ),
 ( #2103, #41502, #15067 ),
 ( #2739, #18894, #24875 ),
 ( #34474, #5511, #5308 ),
 ( #6139, #41710, #25507 ),
 ( #5727, #37665, #18682 ),
 ( #11886, #12308, #41078 ),
 ( #21870, #31690, #28701 ),
 ( #12094, #38507, #2532 ),
 ( #18469, #25296, #32112 ),
 ( #9323, #28067, #34896 ),
 ( #15494, #22286, #35311 ),
 ( #2942, #19103, #15906 ),
 ( #31474, #38299, #41921 ),
 ( #24656, #2318, #15279 ),
 ( #28283, #9119, #41290 ) ),
 .UNSPECIFIED., .F., .F., .T. ) 
 B_SPLINE_SURFACE_WITH_KNOTS ( ( 4, 2, 2, 2, 2, 2, 2, 4 ),
 ( 3, 3 ),
 ( 1.734723475976807094E-18, 0.005291144675846519603, 0.007936717013769778103, 0.01058228935169303747, 0.01322786168961629684, 0.01455064785857792739, 0.01587343402753955621, 0.02116457870338607494 ),
 ( 0.000000000000000000, 1.000000000000000000 ),
 .UNSPECIFIED. ) 
 GEOMETRIC_REPRESENTATION_ITEM ( )  RATIONAL_B_SPLINE_SURFACE ( (
 ( 1.000000000000000000, 0.7071067811865519026, 1.000000000000000000),
 ( 1.000000000000000000, 0.7071067811865519026, 1.000000000000000000),
 ( 1.000000000000000000, 0.7071067811865469066, 1.000000000000000000),
 ( 1.000000000000000000, 0.7071067811865469066, 1.000000000000000000),
 ( 1.000000000000000000, 0.7071067811865472397, 1.000000000000000000),
 ( 1.000000000000000000, 0.7071067811865472397, 1.000000000000000000),
 ( 1.000000000000000000, 0.7071067811865491270, 1.000000000000000000),
 ( 1.000000000000000000, 0.7071067811865491270, 1.000000000000000000),
 ( 1.000000000000000000, 0.7071067811865464625, 1.000000000000000000),
 ( 1.000000000000000000, 0.7071067811865464625, 1.000000000000000000),
 ( 1.000000000000000000, 0.7071067811865472397, 1.000000000000000000),
 ( 1.000000000000000000, 0.7071067811865472397, 1.000000000000000000),
 ( 1.000000000000000000, 0.7071067811865472397, 1.000000000000000000),
 ( 1.000000000000000000, 0.7071067811865472397, 1.000000000000000000),
 ( 1.000000000000000000, 0.7071067811865423547, 1.000000000000000000),
 ( 1.000000000000000000, 0.7071067811865423547, 1.000000000000000000) ) ) 
 REPRESENTATION_ITEM ( '' )  SURFACE ( )  );
#35388=DIRECTION ( 'NONE',  ( -0.9575201071113178530, 0.2883665106726683858, -8.537024980200786319E-16 ) ) ;
#35392=CARTESIAN_POINT ( 'NONE',  ( -17.14500000000466784, 71.11999999999886768, -1.270000000000000684 ) ) ;
#35395=AXIS2_PLACEMENT_3D ( 'NONE', #4086, #23854, #13646 ) ;
#35396=CARTESIAN_POINT ( 'NONE',  ( -8.761523658392190939, 74.56051954986229191, -1.523999999999997135 ) ) ;
#35399=ADVANCED_FACE ( 'NONE', ( #1826 ), #31411, .F. ) ;
#35404=DIRECTION ( 'NONE',  ( -0.8745520943968235761, 0.4849315768086558398, -5.691349986800547879E-16 ) ) ;
#35405=DIRECTION ( 'NONE',  ( -0.7770581983690729722, 0.6294287539884164673, -8.537024980200685740E-16 ) ) ;
#35408=LINE ( 'NONE', #6439, #17776 ) ;
#35413=B_SPLINE_CURVE_WITH_KNOTS ( 'NONE', 3,
 ( #26580, #20802, #7216, #823, #35089, #5912 ),
 .UNSPECIFIED., .F., .F.,
 ( 4, 2, 4 ),
 ( -6.000000000029375625E-08, 0.0006551176351295480036, 0.001310295270259096301 ),
 .UNSPECIFIED. ) ;
#35416=VERTEX_POINT ( 'NONE', #8203 ) ;
#35420=CIRCLE ( 'NONE', #17043, 0.7620000000000000107 ) ;
#35423=CARTESIAN_POINT ( 'NONE',  ( -58.28145228256266108, 0.4519758043100738365, -1.031447170180650463 ) ) ;
#35424=ORIENTED_EDGE ( 'NONE', *, *, #19029, .T. ) ;
#35425=CARTESIAN_POINT ( 'NONE',  ( -56.57399730107058389, 3.557946380840157463, -2.108622681941325183 ) ) ;
#35432=CIRCLE ( 'NONE', #1414, 0.2540000000000062208 ) ;
#35434=CARTESIAN_POINT ( 'NONE',  ( -57.64973313486724038, 1.352533784701764885, -1.499908592384923134 ) ) ;
#35435=EDGE_LOOP ( 'NONE', ( #7592, #23667, #1345, #29127 ) ) ;
#35442=CARTESIAN_POINT ( 'NONE',  ( -53.01551111795199489, 8.729259440421063942, -9.365303671399559428E-15 ) ) ;
#35447=VECTOR ( 'NONE', #18427, 1000.000000000000227 ) ;
#35451=CARTESIAN_POINT ( 'NONE',  ( -52.30895062419047292, 13.66434875625866674, -4.401212925246500873 ) ) ;
#35452=CARTESIAN_POINT ( 'NONE',  ( -47.83226487260633775, 16.75079348177631999, -1.615774049669077117 ) ) ;
#35453=ORIENTED_EDGE ( 'NONE', *, *, #38191, .T. ) ;
#35456=CARTESIAN_POINT ( 'NONE',  ( -46.67889021447872011, 26.03274747417083645, -1.323595506759009499 ) ) ;
#35457=CARTESIAN_POINT ( 'NONE',  ( -52.53650722201378898, 11.97175513791591328, 4.250412846625016172 ) ) ;
#35459=DIRECTION ( 'NONE',  ( -0.8745520943968243532, 0.4849315768086547296, -6.829619984160642269E-16 ) ) ;
#35460=CARTESIAN_POINT ( 'NONE',  ( -54.99893072520226411, 10.64604335972153137, 1.135982259999769983 ) ) ;
#35463=VERTEX_POINT ( 'NONE', #12866 ) ;
#35464=CARTESIAN_POINT ( 'NONE',  ( -52.14602366315243387, 18.74265329119796064, -0.7451446608535732263 ) ) ;
#35483=CYLINDRICAL_SURFACE ( 'NONE', #26589, 0.2540000000000045000 ) ;
#35489=AXIS2_PLACEMENT_3D ( 'NONE', #16025, #9645, #22612 ) ;
#35490=CYLINDRICAL_SURFACE ( 'NONE', #15215, 0.2540000000000000036 ) ;
#35491=ADVANCED_FACE ( 'NONE', ( #31836 ), #42070, .F. ) ;
#35496=AXIS2_PLACEMENT_3D ( 'NONE', #25901, #41688, #38488 ) ;
#35497=DIRECTION ( 'NONE',  ( -5.188838149069472160E-16, 1.699382548006136559E-16, 1.000000000000000000 ) ) ;
#35498=EDGE_CURVE ( 'NONE', #27023, #30178, #35184, .T. ) ;
#35499=CARTESIAN_POINT ( 'NONE',  ( -42.72397600927682504, 22.83316142988638831, -1.683267422954632275 ) ) ;
#35500=VERTEX_POINT ( 'NONE', #12660 ) ;
#35503=TOROIDAL_SURFACE ( 'NONE', #28679, 8.794749999999996959, 0.2540000000000000036 ) ;
#35510=DIRECTION ( 'NONE',  ( -0.7770581983690878491, 0.6294287539883980376, -5.101669463485847584E-16 ) ) ;
#35513=VERTEX_POINT ( 'NONE', #19250 ) ;
#35520=ORIENTED_EDGE ( 'NONE', *, *, #1445, .T. ) ;
#35526=CARTESIAN_POINT ( 'NONE',  ( -15.42835734045148577, 79.74558783746839197, -1.270000000000001350 ) ) ;
#35543=ADVANCED_FACE ( 'NONE', ( #19665 ), #64, .T. ) ;
#35549=LINE ( 'NONE', #39375, #20477 ) ;
#35556=CARTESIAN_POINT ( 'NONE',  ( -47.24381373535820217, 25.63803778330989047, 0.2531820549803469045 ) ) ;
#35559=CARTESIAN_POINT ( 'NONE',  ( -43.87210973174860129, 22.05421410453335795, 2.454571855453426377 ) ) ;
#35563=ORIENTED_EDGE ( 'NONE', *, *, #37098, .F. ) ;
#35578=DIRECTION ( 'NONE',  ( -0.8745520943968243532, 0.4849315768086547296, -5.361993529360573944E-16 ) ) ;
#35579=ORIENTED_EDGE ( 'NONE', *, *, #19339, .F. ) ;
#35583=CARTESIAN_POINT ( 'NONE',  ( -30.01829664378881546, 60.43850663962886216, 1.523999999999993804 ) ) ;
#35591=CARTESIAN_POINT ( 'NONE',  ( -47.64484625134591766, 19.26749830283604936, 4.730721332201270890 ) ) ;
#35597=DIRECTION ( 'NONE',  ( -0.8745520943968240202, 0.4849315768086553402, -6.829619984160650158E-16 ) ) ;
#35598=EDGE_CURVE ( 'NONE', #28714, #4082, #39923, .T. ) ;
#35602=ORIENTED_EDGE ( 'NONE', *, *, #24903, .F. ) ;
#35606=CARTESIAN_POINT ( 'NONE',  ( -58.64342337384959336, -0.3142157529041483821, 0.3359497956446368394 ) ) ;
#35612=VECTOR ( 'NONE', #34826, 1000.000000000000000 ) ;
#35614=DIRECTION ( 'NONE',  ( 0.8745520943968235761, -0.4849315768086558398, 0.000000000000000000 ) ) ;
#35630=ORIENTED_EDGE ( 'NONE', *, *, #40520, .F. ) ;
#35632=VERTEX_POINT ( 'NONE', #33740 ) ;
#35633=DIRECTION ( 'NONE',  ( -5.188838149069472160E-16, 1.699382548006136559E-16, 1.000000000000000000 ) ) ;
#35639=CARTESIAN_POINT ( 'NONE',  ( -57.44144277618438110, 2.261329945018465182, -1.861782675839624313 ) ) ;
#35641=CARTESIAN_POINT ( 'NONE',  ( -49.23283723365199904, 17.42967204962654648, -5.014312523173099834 ) ) ;
#35649=CARTESIAN_POINT ( 'NONE',  ( -58.87911280034276018, -0.2081424763510641984, -0.2451831517279998984 ) ) ;
#35654=VERTEX_POINT ( 'NONE', #36931 ) ;
#35657=AXIS2_PLACEMENT_3D ( 'NONE', #10231, #30289, #20902 ) ;
#35658=CIRCLE ( 'NONE', #22692, 0.6350000000000014522 ) ;
#35667=LINE ( 'NONE', #41643, #17403 ) ;
#35668=CARTESIAN_POINT ( 'NONE',  ( -45.11192300388034937, 21.16850173503701527, -3.873855239238740200 ) ) ;
#35670=CARTESIAN_POINT ( 'NONE',  ( -15.37877921309976870, 79.99470228764801050, -1.524000000000001576 ) ) ;
#35672=CARTESIAN_POINT ( 'NONE',  ( -51.25515452438769159, 14.22119815747982052, 4.625262746768662225 ) ) ;
#35675=CARTESIAN_POINT ( 'NONE',  ( -17.22465686008793995, 48.97870818484556565, 1.524000000000002242 ) ) ;
#35676=CARTESIAN_POINT ( 'NONE',  ( -56.90590057130552282, 4.418898835881354792, 2.427662546266514454 ) ) ;
#35677=CARTESIAN_POINT ( 'NONE',  ( -58.37934292759150168, 0.9822739792931106662, 1.208960021102198246 ) ) ;
#35679=VERTEX_POINT ( 'NONE', #4564 ) ;
#35680=CARTESIAN_POINT ( 'NONE',  ( -55.52324119379100864, 8.418761648454426094, -1.955819887484162356 ) ) ;
#35694=CARTESIAN_POINT ( 'NONE',  ( -23.62918761621517660, 82.45577215708875940, 1.269999999999993134 ) ) ;
#35695=ORIENTED_EDGE ( 'NONE', *, *, #10763, .F. ) ;
#35705=ADVANCED_FACE ( 'NONE', ( #29688 ), #14321, .F. ) ;
#35709=EDGE_LOOP ( 'NONE', ( #25834, #12085, #2292, #12630 ) ) ;
#35714=CARTESIAN_POINT ( 'NONE',  ( -46.42538233320968288, 20.85422009098716956, -4.815137874471035140 ) ) ;
#35718=DIRECTION ( 'NONE',  ( -0.01731298258488073519, 0.9998501190848635423, -1.788962107505278613E-16 ) ) ;
#35725=EDGE_CURVE ( 'NONE', #4992, #31070, #4571, .T. ) ;
#35747=EDGE_CURVE ( 'NONE', #26127, #4116, #7301, .T. ) ;
#35748=VERTEX_POINT ( 'NONE', #31150 ) ;
#35753=CIRCLE ( 'NONE', #17373, 0.2540000000000006142 ) ;
#35754=ORIENTED_EDGE ( 'NONE', *, *, #1518, .F. ) ;
#35756=CARTESIAN_POINT ( 'NONE',  ( -10.73808814597608396, 77.14487411131504757, -1.269999999999998241 ) ) ;
#35760=ADVANCED_FACE ( 'NONE', ( #30943 ), #37214, .T. ) ;
#35762=CARTESIAN_POINT ( 'NONE',  ( -50.94786445731823221, 14.55500684364030661, 4.556750753989597058 ) ) ;
#35763=CARTESIAN_POINT ( 'NONE',  ( -47.06635113313992491, 25.00568333085942996, 1.230463370088882069 ) ) ;
#35765=CARTESIAN_POINT ( 'NONE',  ( -41.88683177698051452, 22.33947639032530219, 1.656270940288490312 ) ) ;
#35768=CARTESIAN_POINT ( 'NONE',  ( -58.18636467486479091, 0.07352994790495170907, -0.3924542439260719773 ) ) ;
#35771=ORIENTED_EDGE ( 'NONE', *, *, #6839, .F. ) ;
#35773=EDGE_CURVE ( 'NONE', #16976, #5685, #5193, .T. ) ;
#35780=EDGE_CURVE ( 'NONE', #332, #19961, #37545, .T. ) ;
#35782=CARTESIAN_POINT ( 'NONE',  ( -19.04204117267709506, 56.84332656279845963, 1.524000000000000243 ) ) ;
#35792=VERTEX_POINT ( 'NONE', #40756 ) ;
#35800=ORIENTED_EDGE ( 'NONE', *, *, #32307, .F. ) ;
#35801=CARTESIAN_POINT ( 'NONE',  ( -41.41491986784952672, 22.70581808553410497, 0.08466666666666171348 ) ) ;
#35808=CARTESIAN_POINT ( 'NONE',  ( -47.90792207059400454, 19.42479681086476617, -5.305186633237529037 ) ) ;
#35814=FACE_OUTER_BOUND ( 'NONE', #22914, .T. ) ;
#35815=VECTOR ( 'NONE', #24659, 1000.000000000000114 ) ;
#35817=CARTESIAN_POINT ( 'NONE',  ( -58.41257333834132481, 0.1697474083129230094, 0.8453419536833289838 ) ) ;
#35818=ADVANCED_FACE ( 'NONE', ( #37756 ), #31769, .T. ) ;
#35819=AXIS2_PLACEMENT_3D ( 'NONE', #3781, #35510, #3568 ) ;
#35820=CARTESIAN_POINT ( 'NONE',  ( -8.473844426907703564, 67.77203500197072117, 1.270000000000003570 ) ) ;
#35824=DIRECTION ( 'NONE',  ( -0.8745520943968241312, 0.4849315768086548406, -5.691349986800536046E-16 ) ) ;
#35836=ADVANCED_FACE ( 'NONE', ( #34573 ), #41998, .T. ) ;
#35837=CARTESIAN_POINT ( 'NONE',  ( -17.14500000000466784, 71.11999999999886768, -1.524000000000000909 ) ) ;
#35842=EDGE_CURVE ( 'NONE', #36653, #28149, #18825, .T. ) ;
#35846=ORIENTED_EDGE ( 'NONE', *, *, #36996, .F. ) ;
#35854=LINE ( 'NONE', #33287, #34059 ) ;
#35855=VECTOR ( 'NONE', #38706, 1000.000000000000227 ) ;
#35859=CARTESIAN_POINT ( 'NONE',  ( -11.32337086946255056, 78.46996359545325106, 1.270000000000000018 ) ) ;
#35862=CARTESIAN_POINT ( 'NONE',  ( -58.43690671596436914, -0.4125963578781866037, -0.2423173958219211055 ) ) ;
#35872=CARTESIAN_POINT ( 'NONE',  ( -23.43300365160792964, 82.12916405548841681, -1.524000000000006017 ) ) ;
#35876=AXIS2_PLACEMENT_3D ( 'NONE', #30153, #16732, #29942 ) ;
#35880=AXIS2_PLACEMENT_3D ( 'NONE', #6855, #30474, #29851 ) ;
#35881=CARTESIAN_POINT ( 'NONE',  ( -47.61549956331939626, 19.66157307908737195, -5.197827534590571119 ) ) ;
#35884=CARTESIAN_POINT ( 'NONE',  ( -46.98348089488082735, 24.79145570443871449, 2.118842393845961070 ) ) ;
#35885=CARTESIAN_POINT ( 'NONE',  ( -28.09515292912719175, 77.51021392068167870, 1.269999999999991580 ) ) ;
#35890=CARTESIAN_POINT ( 'NONE',  ( -57.34105142390578891, 4.241571993195719870, -1.063007725424832192E-14 ) ) ;
#35891=CARTESIAN_POINT ( 'NONE',  ( -57.93941708942283952, 2.052042089854988483, 1.628789306319508245 ) ) ;
#35894=CARTESIAN_POINT ( 'NONE',  ( -53.84631020981186822, 15.55534180636754193, -1.120024938224189362E-14 ) ) ;
#35903=CIRCLE ( 'NONE', #19538, 0.6350000000000014522 ) ;
#35909=DIRECTION ( 'NONE',  ( 0.5149185422762211362, -0.8572391118119444542, 0.000000000000000000 ) ) ;
#35910=VERTEX_POINT ( 'NONE', #41174 ) ;
#35913=CARTESIAN_POINT ( 'NONE',  ( -15.02280320640473121, 73.03244360434628391, -1.269999999999999796 ) ) ;
#35926=LINE ( 'NONE', #22889, #14256 ) ;
#35927=CARTESIAN_POINT ( 'NONE',  ( -48.56815661899837977, 19.24492339269602681, -5.224590812749990931 ) ) ;
#35937=DIRECTION ( 'NONE',  ( -5.188838149069471174E-16, 1.699382548006136313E-16, 1.000000000000000000 ) ) ;
#35939=ORIENTED_EDGE ( 'NONE', *, *, #22903, .T. ) ;
#35946=ORIENTED_EDGE ( 'NONE', *, *, #24320, .F. ) ;
#35954=CARTESIAN_POINT ( 'NONE',  ( -48.44802435120097783, 18.63281525352669021, -5.198089189982387559 ) ) ;
#35955=DIRECTION ( 'NONE',  ( -0.8745520943968235761, 0.4849315768086558398, -4.268512490100410909E-16 ) ) ;
#35959=ORIENTED_EDGE ( 'NONE', *, *, #20866, .T. ) ;
#35961=VECTOR ( 'NONE', #35718, 999.9999999999998863 ) ;
#35964=ORIENTED_EDGE ( 'NONE', *, *, #15232, .F. ) ;
#35968=AXIS2_PLACEMENT_3D ( 'NONE', #16001, #32416, #3246 ) ;
#35973=CARTESIAN_POINT ( 'NONE',  ( -47.68734114412297487, 23.26096984540084023, 2.152999274035547472 ) ) ;
#35975=CARTESIAN_POINT ( 'NONE',  ( -56.26318288983030413, 4.268071985104968213, 2.480832006587838645 ) ) ;
#35976=CARTESIAN_POINT ( 'NONE',  ( -58.74214995731320244, -0.3112433815685096139, 0.2392860922412864966 ) ) ;
#35977=EDGE_CURVE ( 'NONE', #39412, #35748, #20924, .T. ) ;
#35979=DIRECTION ( 'NONE',  ( -0.8745520943968663197, 0.4849315768085789013, -5.691349986800499561E-16 ) ) ;
#35980=EDGE_LOOP ( 'NONE', ( #21435, #16101, #40202, #9014 ) ) ;
#35981=VERTEX_POINT ( 'NONE', #1579 ) ;
#35983=VECTOR ( 'NONE', #3681, 1000.000000000000227 ) ;
#35987=AXIS2_PLACEMENT_3D ( 'NONE', #9072, #5048, #41239 ) ;
#35988=CARTESIAN_POINT ( 'NONE',  ( -47.22545206610593027, 24.52529105818055655, -1.461865184087826286 ) ) ;
#35994=EDGE_CURVE ( 'NONE', #23884, #19740, #2535, .T. ) ;
#35995=CARTESIAN_POINT ( 'NONE',  ( -9.909999474182708212, 76.95545850745379823, 1.270000000000001350 ) ) ;
#36001=VERTEX_POINT ( 'NONE', #15794 ) ;
#36008=ORIENTED_EDGE ( 'NONE', *, *, #39378, .F. ) ;
#36009=CARTESIAN_POINT ( 'NONE',  ( -45.11192300388035648, 21.16850173503701527, 3.873855239238726433 ) ) ;
#36018=EDGE_CURVE ( 'NONE', #14494, #8692, #1860, .T. ) ;
#36020=ORIENTED_EDGE ( 'NONE', *, *, #8709, .T. ) ;
#36021=FACE_OUTER_BOUND ( 'NONE', #5909, .T. ) ;
#36022=DIRECTION ( 'NONE',  ( -5.188838149069472160E-16, 1.699382548006136559E-16, 1.000000000000000000 ) ) ;
#36039=DIRECTION ( 'NONE',  ( 5.188838149069471174E-16, -1.699382548006136313E-16, -1.000000000000000000 ) ) ;
#36044=CARTESIAN_POINT ( 'NONE',  ( -23.16987411132078734, 77.52691185402750307, 1.269999999999994245 ) ) ;
#36050=ORIENTED_EDGE ( 'NONE', *, *, #3924, .F. ) ;
#36053=ORIENTED_EDGE ( 'NONE', *, *, #36079, .T. ) ;
#36059=CARTESIAN_POINT ( 'NONE',  ( -58.66492368201303975, -0.3142542598142069044, -0.3213541728213932802 ) ) ;
#36060=EDGE_CURVE ( 'NONE', #26454, #500, #23596, .T. ) ;
#36062=DIRECTION ( 'NONE',  ( 0.6825627711659039143, 0.7308269722843582228, 2.299753143848015941E-16 ) ) ;
#36066=CARTESIAN_POINT ( 'NONE',  ( -18.27007371177421291, 83.88799758123168715, 1.269999999999994689 ) ) ;
#36067=ADVANCED_FACE ( 'NONE', ( #25599 ), #41323, .T. ) ;
#36070=CARTESIAN_POINT ( 'NONE',  ( -57.81953393267934160, 1.609514594907199392, -1.636666387507151432 ) ) ;
#36074=EDGE_LOOP ( 'NONE', ( #39465, #35946, #9583, #6707 ) ) ;
#36077=EDGE_CURVE ( 'NONE', #33817, #16319, #10688, .T. ) ;
#36079=EDGE_CURVE ( 'NONE', #2275, #35679, #24272, .T. ) ;
#36080=CARTESIAN_POINT ( 'NONE',  ( -43.13073682054402269, 20.84535665847938546, -6.630667737810475277E-15 ) ) ;
#36081=CIRCLE ( 'NONE', #38779, 0.7620000000000000107 ) ;
#36089=CARTESIAN_POINT ( 'NONE',  ( -56.36488200494262202, 4.056002992322685685, -2.423683632884288564 ) ) ;
#36092=CARTESIAN_POINT ( 'NONE',  ( -46.81779053729648865, 25.68675045694219250, -1.510149268906148867 ) ) ;
#36093=DIRECTION ( 'NONE',  ( -0.8745520943968243532, 0.4849315768086547296, -6.829619984160642269E-16 ) ) ;
#36095=CIRCLE ( 'NONE', #21857, 0.6350000000000008971 ) ;
#36096=CARTESIAN_POINT ( 'NONE',  ( -25.97603047661466036, 74.27059221564131519, 1.269999999999992912 ) ) ;
#36099=CARTESIAN_POINT ( 'NONE',  ( -54.68578128246380743, 13.03233524003756472, 0.2705950194912850604 ) ) ;
#36100=CARTESIAN_POINT ( 'NONE',  ( -56.21344593158320180, 5.939860726778031896, 2.828251681716853927 ) ) ;
#36102=EDGE_LOOP ( 'NONE', ( #20271, #8401, #27677, #6630, #24723 ) ) ;
#36103=CARTESIAN_POINT ( 'NONE',  ( -51.68408071790322822, 18.36713515631302585, -1.546689197337258737 ) ) ;
#36105=EDGE_LOOP ( 'NONE', ( #21585, #40499, #5571, #24804 ) ) ;
#36106=FACE_OUTER_BOUND ( 'NONE', #1997, .T. ) ;
#36107=CIRCLE ( 'NONE', #27247, 0.6349999999999971223 ) ;
#36119=ORIENTED_EDGE ( 'NONE', *, *, #27666, .F. ) ;
#36121=ORIENTED_EDGE ( 'NONE', *, *, #40493, .T. ) ;
#36132=ORIENTED_EDGE ( 'NONE', *, *, #16999, .T. ) ;
#36135=FACE_OUTER_BOUND ( 'NONE', #30077, .T. ) ;
#36137=EDGE_CURVE ( 'NONE', #20165, #11776, #22919, .T. ) ;
#36138=CARTESIAN_POINT ( 'NONE',  ( -44.40534991575952972, 23.82367036525651116, -1.730788704199199834 ) ) ;
#36149=CARTESIAN_POINT ( 'NONE',  ( -25.83700401581416983, 71.09321415394998667, -1.270000000000005347 ) ) ;
#36151=ORIENTED_EDGE ( 'NONE', *, *, #7690, .T. ) ;
#36157=CARTESIAN_POINT ( 'NONE',  ( -10.93398011767285283, 82.89560043784887000, -1.269999999999999352 ) ) ;
#36160=ORIENTED_EDGE ( 'NONE', *, *, #8614, .F. ) ;
#36164=DIRECTION ( 'NONE',  ( -5.188838149069472160E-16, 1.699382548006136559E-16, 1.000000000000000000 ) ) ;
#36171=TOROIDAL_SURFACE ( 'NONE', #27308, 8.794749999999996959, 0.2540000000000000036 ) ;
#36178=CARTESIAN_POINT ( 'NONE',  ( -46.76714659696573051, 20.35889133747190272, 4.890039387020951089 ) ) ;
#36185=EDGE_CURVE ( 'NONE', #6464, #11324, #28592, .T. ) ;
#36190=CARTESIAN_POINT ( 'NONE',  ( -50.89935680924180161, 14.64024222003797426, 4.571006890225723929 ) ) ;
#36191=CARTESIAN_POINT ( 'NONE',  ( -49.70354155341430413, 23.42381788805148091, -9.364162196477891358E-15 ) ) ;
#36193=CARTESIAN_POINT ( 'NONE',  ( -50.78166962549567387, 16.07998339508975860, 4.893817234114164805 ) ) ;
#36194=DIRECTION ( 'NONE',  ( -0.6850534820564617711, 0.7284927773988681965, -8.537024980200850414E-16 ) ) ;
#36198=CARTESIAN_POINT ( 'NONE',  ( -46.31144060707497090, 24.05480373873685451, 2.308638262703916588 ) ) ;
#36204=DIRECTION ( 'NONE',  ( 5.188838149069472160E-16, -1.699382548006136559E-16, -1.000000000000000000 ) ) ;
#36207=CARTESIAN_POINT ( 'NONE',  ( -24.32950799593924884, 77.42192949967211746, 1.269999999999993578 ) ) ;
#36219=CIRCLE ( 'NONE', #37571, 0.2540000000000015579 ) ;
#36221=ORIENTED_EDGE ( 'NONE', *, *, #10010, .T. ) ;
#36222=CARTESIAN_POINT ( 'NONE',  ( -46.36222913602040308, 19.75614878210438263, 3.583538483381419670 ) ) ;
#36233=CIRCLE ( 'NONE', #33519, 0.7620000000000015650 ) ;
#36240=EDGE_CURVE ( 'NONE', #4992, #30709, #23650, .T. ) ;
#36243=AXIS2_PLACEMENT_3D ( 'NONE', #20559, #35356, #33588 ) ;
#36251=DIRECTION ( 'NONE',  ( 5.188838149069472160E-16, -1.699382548006136559E-16, -1.000000000000000000 ) ) ;
#36254=CIRCLE ( 'NONE', #2931, 0.2539999999999998925 ) ;
#36256=CARTESIAN_POINT ( 'NONE',  ( -47.02779878473986486, 24.11651466984139702, -2.637840241488492943 ) ) ;
#36259=EDGE_CURVE ( 'NONE', #13978, #2010, #3227, .T. ) ;
#36262=CIRCLE ( 'NONE', #23308, 0.3810000000000015041 ) ;
#36265=DIRECTION ( 'NONE',  ( -0.01731298258488772612, 0.9998501190848633202, -1.788962107505314604E-16 ) ) ;
#36273=CARTESIAN_POINT ( 'NONE',  ( -58.63359593288674887, -0.2965917858236741256, -0.3663021125533588163 ) ) ;
#36274=VERTEX_POINT ( 'NONE', #16851 ) ;
#36275=DIRECTION ( 'NONE',  ( -5.188838149069472160E-16, 1.699382548006136559E-16, 1.000000000000000000 ) ) ;
#36291=AXIS2_PLACEMENT_3D ( 'NONE', #23378, #33214, #17001 ) ;
#36292=CARTESIAN_POINT ( 'NONE',  ( -58.34514637059943709, -0.2398883667947132592, 0.1955437934783506304 ) ) ;
#36293=EDGE_CURVE ( 'NONE', #16976, #5996, #14093, .T. ) ;
#36299=DIRECTION ( 'NONE',  ( -5.188838149069472160E-16, 1.699382548006136559E-16, 1.000000000000000000 ) ) ;
#36300=ADVANCED_FACE ( 'NONE', ( #19825 ), #33269, .T. ) ;
#36301=CARTESIAN_POINT ( 'NONE',  ( -54.22787649382022579, 6.886497292746652121, -0.2709450413641087407 ) ) ;
#36307=CARTESIAN_POINT ( 'NONE',  ( -33.42971872652992005, 49.93539301574497102, -1.270000000000005569 ) ) ;
#36308=FACE_OUTER_BOUND ( 'NONE', #19675, .T. ) ;
#36309=DIRECTION ( 'NONE',  ( 5.188838149069472160E-16, -1.699382548006136559E-16, -1.000000000000000000 ) ) ;
#36311=CARTESIAN_POINT ( 'NONE',  ( -57.90853684698416259, 2.514838786807804816, -1.057700776740060064E-14 ) ) ;
#36312=CARTESIAN_POINT ( 'NONE',  ( -57.85534701229748578, 0.8496279762696679061, 1.203237356453206619 ) ) ;
#36314=AXIS2_PLACEMENT_3D ( 'NONE', #5069, #2072, #18022 ) ;
#36316=CARTESIAN_POINT ( 'NONE',  ( -56.03617394834085985, 6.499552843647532718, -2.676235688315271588 ) ) ;
#36319=ORIENTED_EDGE ( 'NONE', *, *, #40180, .T. ) ;
#36325=AXIS2_PLACEMENT_3D ( 'NONE', #15726, #35137, #40899 ) ;
#36327=EDGE_CURVE ( 'NONE', #22227, #25505, #33180, .T. ) ;
#36329=DIRECTION ( 'NONE',  ( -0.8745520943968354555, 0.4849315768086345235, -6.829619984160664949E-16 ) ) ;
#36333=FACE_OUTER_BOUND ( 'NONE', #34164, .T. ) ;
#36337=CARTESIAN_POINT ( 'NONE',  ( -57.93467410668397122, 0.6461773018132880297, -0.9430256072699126912 ) ) ;
#36340=AXIS2_PLACEMENT_3D ( 'NONE', #17085, #23893, #10695 ) ;
#36351=AXIS2_PLACEMENT_3D ( 'NONE', #38801, #12804, #35824 ) ;
#36352=CARTESIAN_POINT ( 'NONE',  ( -58.83227707057486811, -0.08366279997995551554, -1.529465441686574059E-14 ) ) ;
#36354=CARTESIAN_POINT ( 'NONE',  ( -55.03109054507046238, 6.816801101491506643, -3.135084751894932076 ) ) ;
#36355=DIRECTION ( 'NONE',  ( 0.9816537812491076265, 0.1906721105965138718, 4.769617732184456426E-16 ) ) ;
#36364=AXIS2_PLACEMENT_3D ( 'NONE', #36394, #29777, #4023 ) ;
#36370=CARTESIAN_POINT ( 'NONE',  ( -14.64596739026573857, 69.73430801926814127, -1.269999999999999130 ) ) ;
#36371=CIRCLE ( 'NONE', #10503, 0.7620000000000036744 ) ;
#36386=CARTESIAN_POINT ( 'NONE',  ( -56.80696390459748102, 3.604343092604253673, -2.316781442554163739 ) ) ;
#36394=CARTESIAN_POINT ( 'NONE',  ( -17.64290547347870941, 83.78857423953914463, -1.524000000000003130 ) ) ;
#36398=DIRECTION ( 'NONE',  ( -5.188838149069472160E-16, 1.699382548006136559E-16, 1.000000000000000000 ) ) ;
#36399=CARTESIAN_POINT ( 'NONE',  ( -29.27763062208790856, 65.70811510315778037, -1.270000000000006013 ) ) ;
#36405=CARTESIAN_POINT ( 'NONE',  ( -52.44164295988605318, 11.83295133839460611, 4.069468471668873377 ) ) ;
#36406=CARTESIAN_POINT ( 'NONE',  ( -47.08352113710599696, 24.38425570713750190, 2.219725161937576630 ) ) ;
#36408=CARTESIAN_POINT ( 'NONE',  ( -55.60486134785667645, 7.243031971518515633, 3.140198620020484110 ) ) ;
#36409=CARTESIAN_POINT ( 'NONE',  ( -58.18695740882700562, 0.6575158937857172869, 1.151667878608726214 ) ) ;
#36411=CARTESIAN_POINT ( 'NONE',  ( -58.12768216001780530, 0.1527613808938732554, -0.09815255304910418255 ) ) ;
#36413=CARTESIAN_POINT ( 'NONE',  ( -44.40534991575952972, 23.82367036525651116, 1.730788704199185624 ) ) ;
#36428=CARTESIAN_POINT ( 'NONE',  ( -26.29578028364076658, 73.87584665086983193, -1.524000000000006017 ) ) ;
#36434=ORIENTED_EDGE ( 'NONE', *, *, #11385, .T. ) ;
#36435=CARTESIAN_POINT ( 'NONE',  ( -45.43219756685621036, 19.09711438432238495, 1.200471166368901166 ) ) ;
#36444=CYLINDRICAL_SURFACE ( 'NONE', #5485, 0.6350000000000014522 ) ;
#36456=AXIS2_PLACEMENT_3D ( 'NONE', #8273, #21871, #17847 ) ;
#36465=DIRECTION ( 'NONE',  ( 5.188838149069472160E-16, -1.699382548006136559E-16, -1.000000000000000000 ) ) ;
#36471=DIRECTION ( 'NONE',  ( 0.000000000000000000, 0.000000000000000000, 1.000000000000000000 ) ) ;
#36473=DIRECTION ( 'NONE',  ( 0.9816537812491089587, 0.1906721105965065444, 4.769617732184475162E-16 ) ) ;
#36478=CARTESIAN_POINT ( 'NONE',  ( -58.59553834934886396, -0.2237177117754586830, -0.4722778291337721424 ) ) ;
#36480=CARTESIAN_POINT ( 'NONE',  ( -19.33375693323417366, 80.42273151551299293, 1.269999999999995577 ) ) ;
#36482=SURFACE_STYLE_USAGE ( .BOTH. , #30699 ) ;
#36487=DIRECTION ( 'NONE',  ( 0.7548010569845216011, 0.6559537821943317581, 2.801824109679581255E-16 ) ) ;
#36492=ORIENTED_EDGE ( 'NONE', *, *, #1985, .F. ) ;
#36502=( BOUNDED_SURFACE ( )  B_SPLINE_SURFACE ( 3, 2, ( 
 ( #14130, #8379, #24768 ),
 ( #27132, #40145, #2002 ),
 ( #33751, #10937, #27555 ),
 ( #7763, #37352, #27966 ),
 ( #21344, #4577, #37766 ),
 ( #17535, #30953, #40975 ),
 ( #1588, #8170, #34370 ),
 ( #17952, #30536, #40562 ),
 ( #31161, #5203, #14332 ),
 ( #7967, #27343, #21137 ),
 ( #20511, #37145, #40355 ),
 ( #11150, #33539, #24137 ),
 ( #1793, #33960, #4789 ),
 ( #40767, #17739, #34167 ),
 ( #11360, #4993, #11565 ),
 ( #14756, #27756, #29012 ),
 ( #28813, #3056, #5834 ),
 ( #31801, #18366, #38415 ),
 ( #9018, #18582, #21981 ),
 ( #41400, #32223, #24983 ),
 ( #15806, #12827, #18788 ),
 ( #6041, #19214, #9424 ),
 ( #8807, #34791, #31591 ),
 ( #2428, #35014, #6244 ) ),
 .UNSPECIFIED., .F., .F., .F. ) 
 B_SPLINE_SURFACE_WITH_KNOTS ( ( 4, 2, 2, 2, 2, 2, 2, 2, 2, 2, 2, 4 ),
 ( 3, 3 ),
 ( 0.000000000000000000, 0.0005614604826172228322, 0.001122920965234445664, 0.001684381447851668497, 0.002245841930468891329, 0.003368762895703336993, 0.004491683860937782657, 0.005614604826172228322, 0.006737525791406673986, 0.007298986274023896818, 0.007860446756641119651, 0.008983367721875565315 ),
 ( 0.000000000000000000, 1.000000000000000000 ),
 .UNSPECIFIED. ) 
 GEOMETRIC_REPRESENTATION_ITEM ( )  RATIONAL_B_SPLINE_SURFACE ( (
 ( 1.000000000000000000, 0.9987193938133342996, 1.000000000000000000),
 ( 1.000000000000000000, 0.9982000373971027241, 1.000000000000000000),
 ( 1.000000000000000000, 0.9975619604953736008, 1.000000000000000000),
 ( 1.000000000000000000, 0.9916939477464365993, 1.000000000000000000),
 ( 1.000000000000000000, 0.9861209039935189269, 1.000000000000000000),
 ( 1.000000000000000000, 0.9617740169780845116, 1.000000000000000000),
 ( 1.000000000000000000, 0.9448443023889108172, 1.000000000000000000),
 ( 1.000000000000000000, 0.9146158020808421441, 1.000000000000000000),
 ( 1.000000000000000000, 0.9004045293487663582, 1.000000000000000000),
 ( 1.000000000000000000, 0.8619933248317470653, 1.000000000000000000),
 ( 1.000000000000000000, 0.8427343359422859725, 1.000000000000000000),
 ( 1.000000000000000000, 0.8121850874637416284, 1.000000000000000000),
 ( 1.000000000000000000, 0.8005416906217645012, 1.000000000000000000),
 ( 1.000000000000000000, 0.7821458849528583057, 1.000000000000000000),
 ( 1.000000000000000000, 0.7751654015759510408, 1.000000000000000000),
 ( 1.000000000000000000, 0.7626205617104924173, 1.000000000000000000),
 ( 1.000000000000000000, 0.7574054414911801647, 1.000000000000000000),
 ( 1.000000000000000000, 0.7453179101192215494, 1.000000000000000000),
 ( 1.000000000000000000, 0.7405197175285387345, 1.000000000000000000),
 ( 1.000000000000000000, 0.7299770405551697650, 1.000000000000000000),
 ( 1.000000000000000000, 0.7243132446522438928, 1.000000000000000000),
 ( 1.000000000000000000, 0.7087302219173966522, 1.000000000000000000),
 ( 1.000000000000000000, 0.7007553748469402821, 1.000000000000000000),
 ( 1.000000000000000000, 0.7072256012393058899, 1.000000000000000000) ) ) 
 REPRESENTATION_ITEM ( '' )  SURFACE ( )  );
#36503=CARTESIAN_POINT ( 'NONE',  ( -52.76126113563441322, 10.11686208896574257, -1.835409310531190163 ) ) ;
#36506=CARTESIAN_POINT ( 'NONE',  ( -11.32337086946255056, 78.46996359545325106, -1.523999999999999133 ) ) ;
#36508=CARTESIAN_POINT ( 'NONE',  ( -29.30569680556072498, 61.36914094226862204, -1.524000000003056243 ) ) ;
#36509=DIRECTION ( 'NONE',  ( -5.188838149069471174E-16, 1.699382548006136313E-16, 1.000000000000000000 ) ) ;
#36512=CARTESIAN_POINT ( 'NONE',  ( -57.97744691355249813, 2.174673694799844625, 0.6577596567055979948 ) ) ;
#36514=CARTESIAN_POINT ( 'NONE',  ( -58.75009580408200094, 0.1057190229620807997, 0.6617493214610802310 ) ) ;
#36516=AXIS2_PLACEMENT_3D ( 'NONE', #19092, #32098, #28896 ) ;
#36517=ORIENTED_EDGE ( 'NONE', *, *, #14611, .T. ) ;
#36518=CARTESIAN_POINT ( 'NONE',  ( -57.35225397299146977, 4.112755766825001658, -0.3099640861128369895 ) ) ;
#36536=CARTESIAN_POINT ( 'NONE',  ( -57.85882094617455351, 0.8103094007012910938, -1.033824511878239871 ) ) ;
#36541=AXIS2_PLACEMENT_3D ( 'NONE', #4335, #7308, #24105 ) ;
#36543=CARTESIAN_POINT ( 'NONE',  ( -46.82679756180435504, 21.08486709759267086, -4.907624977305287572 ) ) ;
#36547=ORIENTED_EDGE ( 'NONE', *, *, #33964, .F. ) ;
#36552=CARTESIAN_POINT ( 'NONE',  ( -49.56090548067184898, 17.87959676410238430, -5.165259844110624776 ) ) ;
#36553=AXIS2_PLACEMENT_3D ( 'NONE', #23271, #27746, #14536 ) ;
#36554=CARTESIAN_POINT ( 'NONE',  ( -24.10666987309389597, 82.16896248603319464, -1.270000000000006235 ) ) ;
#36556=CYLINDRICAL_SURFACE ( 'NONE', #29437, 0.5080000000000000071 ) ;
#36563=FACE_OUTER_BOUND ( 'NONE', #35435, .T. ) ;
#36565=AXIS2_PLACEMENT_3D ( 'NONE', #15653, #9285, #32065 ) ;
#36567=ORIENTED_EDGE ( 'NONE', *, *, #13594, .F. ) ;
#36570=ORIENTED_EDGE ( 'NONE', *, *, #6820, .T. ) ;
#36581=DIRECTION ( 'NONE',  ( 0.8745520943968240202, -0.4849315768086553402, 6.829619984160650158E-16 ) ) ;
#36582=AXIS2_PLACEMENT_3D ( 'NONE', #20048, #33066, #10258 ) ;
#36586=CARTESIAN_POINT ( 'NONE',  ( -58.64207371057509022, -0.3086014758122701540, -0.3447476069571805413 ) ) ;
#36591=ORIENTED_EDGE ( 'NONE', *, *, #27215, .F. ) ;
#36592=ORIENTED_EDGE ( 'NONE', *, *, #28804, .F. ) ;
#36593=EDGE_CURVE ( 'NONE', #35792, #4212, #8683, .T. ) ;
#36596=CARTESIAN_POINT ( 'NONE',  ( -41.35619903644415984, 22.77303286471932964, 1.271070091490069665 ) ) ;
#36597=CIRCLE ( 'NONE', #33865, 0.2540000000000012248 ) ;
#36611=CARTESIAN_POINT ( 'NONE',  ( -56.16217148015365268, 4.421972936757549100, 2.364476696496186303 ) ) ;
#36612=CARTESIAN_POINT ( 'NONE',  ( -50.25741847910705928, 21.95975045971864503, 0.7628348698132231265 ) ) ;
#36614=CARTESIAN_POINT ( 'NONE',  ( -52.76912830878634253, 12.08540908813377612, 4.334427935445234858 ) ) ;
#36615=CARTESIAN_POINT ( 'NONE',  ( -58.58875816907507783, -0.2095754749432666153, 0.4896725462942392304 ) ) ;
#36619=CARTESIAN_POINT ( 'NONE',  ( -41.45218294293373162, 22.69057396248467384, 1.547390787314418592 ) ) ;
#36629=CARTESIAN_POINT ( 'NONE',  ( -46.92937102808930661, 20.25120335581494047, 4.971330492147314928 ) ) ;
#36632=CARTESIAN_POINT ( 'NONE',  ( -5.591535794131393899, 65.03215273817657760, -1.269999999999993801 ) ) ;
#36641=CARTESIAN_POINT ( 'NONE',  ( -48.35712625370394591, 16.55775765112550602, 2.292466156223448071 ) ) ;
#36648=VECTOR ( 'NONE', #21543, 1000.000000000000114 ) ;
#36651=LINE ( 'NONE', #33671, #22438 ) ;
#36653=VERTEX_POINT ( 'NONE', #4728 ) ;
#36656=EDGE_CURVE ( 'NONE', #28056, #41432, #8315, .T. ) ;
#36658=EDGE_CURVE ( 'NONE', #6380, #15145, #16832, .T. ) ;
#36659=CARTESIAN_POINT ( 'NONE',  ( -10.53334313995851801, 65.32054992887103140, 1.524000000000002908 ) ) ;
#36661=AXIS2_PLACEMENT_3D ( 'NONE', #38700, #3344, #22268 ) ;
#36662=CARTESIAN_POINT ( 'NONE',  ( -30.44847906516384128, 70.61110078258337808, -1.524000000000007571 ) ) ;
#36672=CARTESIAN_POINT ( 'NONE',  ( -16.02764313970816090, 80.34763903973272647, -1.270000000000001794 ) ) ;
#36675=DIRECTION ( 'NONE',  ( 0.8745520943968280170, -0.4849315768086480682, 5.361993529360581832E-16 ) ) ;
#36681=DIRECTION ( 'NONE',  ( 5.188838149069472160E-16, -1.699382548006136559E-16, -1.000000000000000000 ) ) ;
#36690=CARTESIAN_POINT ( 'NONE',  ( -47.61268983602954563, 19.67534098009182841, 5.209569014970943712 ) ) ;
#36691=VECTOR ( 'NONE', #39985, 1000.000000000000114 ) ;
#36693=AXIS2_PLACEMENT_3D ( 'NONE', #39876, #27079, #40087 ) ;
#36699=VERTEX_POINT ( 'NONE', #35353 ) ;
#36702=CARTESIAN_POINT ( 'NONE',  ( -55.35389262108063235, 6.100188123704747056, 2.822635004243398971 ) ) ;
#36703=EDGE_CURVE ( 'NONE', #4510, #5052, #38552, .T. ) ;
#36709=CARTESIAN_POINT ( 'NONE',  ( -24.26619908708081041, 81.70586579672512073, -1.524000000000006239 ) ) ;
#36711=CARTESIAN_POINT ( 'NONE',  ( -55.14069116334859189, 5.401725095812784261, -9.794129604158680367E-15 ) ) ;
#36714=ORIENTED_EDGE ( 'NONE', *, *, #41474, .T. ) ;
#36715=CARTESIAN_POINT ( 'NONE',  ( -15.77830307927088604, 80.39606975582424297, 1.269999999999997575 ) ) ;
#36716=CARTESIAN_POINT ( 'NONE',  ( -14.60888863026623952, 79.54114996201613508, -1.270000000000000906 ) ) ;
#36717=CARTESIAN_POINT ( 'NONE',  ( -29.57263912055365296, 58.75010695897971402, -1.524000000000004906 ) ) ;
#36721=CARTESIAN_POINT ( 'NONE',  ( -58.46425016648313999, 0.8496528882456222398, 0.7404953295986751449 ) ) ;
#36724=ORIENTED_EDGE ( 'NONE', *, *, #36240, .F. ) ;
#36725=CARTESIAN_POINT ( 'NONE',  ( -57.66243511465493299, 3.255537196535568611, -1.068383054469936886E-14 ) ) ;
#36727=ORIENTED_EDGE ( 'NONE', *, *, #18928, .T. ) ;
#36735=CARTESIAN_POINT ( 'NONE',  ( -29.82668814030757787, 58.78177181444144139, 1.269999999999993578 ) ) ;
#36743=CARTESIAN_POINT ( 'NONE',  ( -58.10440571236197371, 0.2782998738747570200, -0.7125144706669881423 ) ) ;
#36749=CARTESIAN_POINT ( 'NONE',  ( -43.24646561529713296, 21.63922848039483071, -2.381786957946274264 ) ) ;
#36752=VECTOR ( 'NONE', #21684, 1000.000000000000000 ) ;
#36755=EDGE_LOOP ( 'NONE', ( #31097, #25271, #9921, #17651, #35100, #12306, #17602, #14973, #13053, #24483, #33659, #39136, #21270, #16019, #8711, #5830, #38129, #3332, #33873, #19211, #23770, #17076, #8006, #820, #35162, #12421, #37468, #21696, #13557, #28601, #31280, #31715, #38369, #20904, #20931, #38919, #33378, #24098, #33721, #19642, #2427, #42147, #12246, #27552, #26170, #36570, #16341, #31160, #14103, #11202, #30090, #9383, #17374, #21673, #37687, #24187, #30696, #27472, #26550, #11476, #2557, #20698, #28309, #15533, #3813, #13184, #17886, #11415, #3495, #26571, #4218, #400, #21196, #27605, #2635, #41116 ) ) ;
#36758=DIRECTION ( 'NONE',  ( -0.8745520943968240202, 0.4849315768086551737, -5.361993529360572958E-16 ) ) ;
#36761=CARTESIAN_POINT ( 'NONE',  ( -55.60508136934060275, 7.116827924314645060, -3.170888472016298198 ) ) ;
#36771=AXIS2_PLACEMENT_3D ( 'NONE', #31086, #5541, #31291 ) ;
#36773=CARTESIAN_POINT ( 'NONE',  ( -58.28497307353763546, -0.1385909279409125450, 0.01567725181048698277 ) ) ;
#36777=CARTESIAN_POINT ( 'NONE',  ( -47.36536141536632982, 24.59964078100214380, -1.062456689557177203 ) ) ;
#36779=CARTESIAN_POINT ( 'NONE',  ( -47.06702646257116385, 25.34112732371119137, -1.513569369951335286 ) ) ;
#36781=DIRECTION ( 'NONE',  ( 0.9816537812491076265, 0.1906721105965138718, 4.769617732184456426E-16 ) ) ;
#36785=CARTESIAN_POINT ( 'NONE',  ( -25.77058783747419213, 72.83664265955201245, -1.270000000000005569 ) ) ;
#36787=CIRCLE ( 'NONE', #18388, 0.3809999999999984510 ) ;
#36788=ORIENTED_EDGE ( 'NONE', *, *, #4277, .F. ) ;
#36790=ADVANCED_FACE ( 'NONE', ( #25133 ), #23527, .T. ) ;
#36797=CARTESIAN_POINT ( 'NONE',  ( -58.07568876781230216, 0.3868594689444180834, -1.028118745741293028 ) ) ;
#36798=CARTESIAN_POINT ( 'NONE',  ( -28.36525985791271154, 77.02308833105713859, -1.270000000000007345 ) ) ;
#36803=ADVANCED_FACE ( 'NONE', ( #30951 ), #10711, .T. ) ;
#36804=EDGE_LOOP ( 'NONE', ( #26090, #27300, #22079, #2864 ) ) ;
#36808=CARTESIAN_POINT ( 'NONE',  ( -43.06611735332018043, 21.60822042109154850, 2.043235477782671783 ) ) ;
#36810=ORIENTED_EDGE ( 'NONE', *, *, #25126, .F. ) ;
#36813=CARTESIAN_POINT ( 'NONE',  ( -29.37460785692852028, 66.57574643235753342, -1.270000000000006457 ) ) ;
#36817=DIRECTION ( 'NONE',  ( 0.2290273297124504059, -0.9734199927291325993, 0.000000000000000000 ) ) ;
#36820=CARTESIAN_POINT ( 'NONE',  ( -52.55726398868221594, 11.61499462435256547, 4.027787250912923334 ) ) ;
#36821=CARTESIAN_POINT ( 'NONE',  ( -48.36699572807423664, 24.50126085711046997, 0.4363764532069195901 ) ) ;
#36822=VECTOR ( 'NONE', #28355, 999.9999999999998863 ) ;
#36823=CARTESIAN_POINT ( 'NONE',  ( -49.56090548067184898, 17.87959676410238430, 5.165259844110607013 ) ) ;
#36824=CARTESIAN_POINT ( 'NONE',  ( -58.62245367815513220, -0.2772137513683323173, 0.3975356116906103021 ) ) ;
#36829=CARTESIAN_POINT ( 'NONE',  ( -44.66298991629287940, 23.47648082339880915, 1.964675176939932655 ) ) ;
#36840=CARTESIAN_POINT ( 'NONE',  ( -46.34235131104849614, 20.67093754025273356, 4.736928721792746266 ) ) ;
#36843=ADVANCED_FACE ( 'NONE', ( #40559 ), #8167, .T. ) ;
#36846=CARTESIAN_POINT ( 'NONE',  ( -8.258874273888745066, 69.93630909653145977, 1.270000000000003126 ) ) ;
#36849=AXIS2_PLACEMENT_3D ( 'NONE', #13245, #484, #16005 ) ;
#36854=ORIENTED_EDGE ( 'NONE', *, *, #28512, .T. ) ;
#36855=CARTESIAN_POINT ( 'NONE',  ( -50.84949806483948720, 11.71728973011883923, -8.098653904493606571E-15 ) ) ;
#36862=VECTOR ( 'NONE', #37484, 1000.000000000000114 ) ;
#36869=VERTEX_POINT ( 'NONE', #27754 ) ;
#36874=CARTESIAN_POINT ( 'NONE',  ( -17.64290547347870941, 83.78857423953914463, 1.269999999999996021 ) ) ;
#36876=DIRECTION ( 'NONE',  ( 5.188838149069472160E-16, -1.699382548006136559E-16, -1.000000000000000000 ) ) ;
#36881=ORIENTED_EDGE ( 'NONE', *, *, #21414, .T. ) ;
#36888=CIRCLE ( 'NONE', #28719, 0.5080000000000000071 ) ;
#36890=DIRECTION ( 'NONE',  ( -5.188838149069472160E-16, 1.699382548006136559E-16, 1.000000000000000000 ) ) ;
#36896=CARTESIAN_POINT ( 'NONE',  ( -24.57769139521899149, 76.70147894597536720, -1.270000000000005569 ) ) ;
#36897=ORIENTED_EDGE ( 'NONE', *, *, #14987, .T. ) ;
#36907=CIRCLE ( 'NONE', #843, 0.2539999999999978386 ) ;
#36917=CARTESIAN_POINT ( 'NONE',  ( -47.84356795211456870, 19.38525671449504983, 5.197506975155130604 ) ) ;
#36926=CARTESIAN_POINT ( 'NONE',  ( -55.14069116334857767, 5.401725095812811794, -0.2259897844578017678 ) ) ;
#36928=DIRECTION ( 'NONE',  ( -0.8745520943968235761, 0.4849315768086558953, -5.361993529360570985E-16 ) ) ;
#36931=CARTESIAN_POINT ( 'NONE',  ( -18.27007371177420936, 83.88799758123168715, -1.270000000000003570 ) ) ;
#36935=CARTESIAN_POINT ( 'NONE',  ( -57.80399136194962040, 2.779771081967835400, 0.2452555687351543334 ) ) ;
#36936=CARTESIAN_POINT ( 'NONE',  ( -58.87911280034276018, -0.2081424763510641984, 0.2451831517279786654 ) ) ;
#36939=CARTESIAN_POINT ( 'NONE',  ( -57.83255607995954506, 2.614142775670388996, -0.5104628509321665897 ) ) ;
#36946=TOROIDAL_SURFACE ( 'NONE', #10414, 8.794749999999996959, 0.2540000000000000036 ) ;
#36949=CARTESIAN_POINT ( 'NONE',  ( -17.14500000000466784, 71.11999999999886768, 1.269999999999998241 ) ) ;
#36952=CARTESIAN_POINT ( 'NONE',  ( -49.00328780856283828, 17.83307836943493641, -5.117960591156088590 ) ) ;
#36956=CARTESIAN_POINT ( 'NONE',  ( -57.92782709497848970, 0.6610469618635247402, -0.9517285047954554544 ) ) ;
#36960=EDGE_CURVE ( 'NONE', #5222, #32069, #19838, .T. ) ;
#36961=CARTESIAN_POINT ( 'NONE',  ( -43.49527490626578441, 22.26612824116996237, -2.150709692269579865 ) ) ;
#36971=CARTESIAN_POINT ( 'NONE',  ( -49.19743978460682143, 17.65503563884207594, -5.190924102448302158 ) ) ;
#36972=CARTESIAN_POINT ( 'NONE',  ( -17.08598887363762131, 83.79821757228496892, 1.523999999999996469 ) ) ;
#36984=CARTESIAN_POINT ( 'NONE',  ( -57.53554607470949378, 1.398951746849091959, 0.8928682508385403782 ) ) ;
#36986=ORIENTED_EDGE ( 'NONE', *, *, #3012, .T. ) ;
#36987=CARTESIAN_POINT ( 'NONE',  ( -46.68395179480138779, 26.03198510454123848, -1.524000000000008015 ) ) ;
#36996=EDGE_CURVE ( 'NONE', #32811, #6738, #23022, .T. ) ;
#36997=CARTESIAN_POINT ( 'NONE',  ( -22.98045850745951668, 78.35500052582088415, -1.270000000000005125 ) ) ;
#36999=EDGE_CURVE ( 'NONE', #7108, #32222, #31124, .T. ) ;
#37002=CARTESIAN_POINT ( 'NONE',  ( -23.75997692595333177, 82.67351089148900201, 1.269999999999992024 ) ) ;
#37007=CARTESIAN_POINT ( 'NONE',  ( -58.67410397513807396, -0.3138866149756391888, -0.3147537707001585860 ) ) ;
#37009=AXIS2_PLACEMENT_3D ( 'NONE', #27243, #14444, #11459 ) ;
#37014=VECTOR ( 'NONE', #19248, 1000.000000000000000 ) ;
#37017=DIRECTION ( 'NONE',  ( -0.8745520943968245753, 0.4849315768086539524, -5.691349986800526185E-16 ) ) ;
#37018=AXIS2_PLACEMENT_3D ( 'NONE', #17276, #23868, #30265 ) ;
#37020=VERTEX_POINT ( 'NONE', #32004 ) ;
#37022=DIRECTION ( 'NONE',  ( -0.9876665170007969952, 0.1565721916417935344, -5.390917751951444915E-16 ) ) ;
#37023=AXIS2_PLACEMENT_3D ( 'NONE', #28778, #12997, #32819 ) ;
#37031=DIRECTION ( 'NONE',  ( -5.188838149069472160E-16, 1.699382548006136559E-16, 1.000000000000000000 ) ) ;
#37032=CARTESIAN_POINT ( 'NONE',  ( -57.54159257952407103, 1.494932415318306340, 1.359492011164181946 ) ) ;
#37033=CARTESIAN_POINT ( 'NONE',  ( -57.57967628038989005, 1.451576601202181349, 1.494865757154131725 ) ) ;
#37034=CARTESIAN_POINT ( 'NONE',  ( -57.61954905543894512, 1.880482199989210956, 1.716091637445736007 ) ) ;
#37037=ORIENTED_EDGE ( 'NONE', *, *, #13059, .T. ) ;
#37038=CARTESIAN_POINT ( 'NONE',  ( -41.88683177698051452, 22.33947639032530219, 1.656270940288490312 ) ) ;
#37043=SURFACE_SIDE_STYLE ('',( #11043 ) ) ;
#37045=EDGE_CURVE ( 'NONE', #32933, #11474, #16011, .T. ) ;
#37046=ORIENTED_EDGE ( 'NONE', *, *, #32458, .T. ) ;
#37050=CARTESIAN_POINT ( 'NONE',  ( -45.09675090431021260, 21.02858785303205380, 3.680331723257769028 ) ) ;
#37062=EDGE_CURVE ( 'NONE', #29590, #16766, #34547, .T. ) ;
#37063=CARTESIAN_POINT ( 'NONE',  ( -50.34589867275522579, 15.36027825638806910, 4.364407372394862428 ) ) ;
#37064=PRODUCT_CONTEXT ( 'NONE', #25165, 'mechanical' ) ;
#37073=ORIENTED_EDGE ( 'NONE', *, *, #6562, .F. ) ;
#37077=DIRECTION ( 'NONE',  ( 0.3213437296502729135, -0.9469626219732499850, 2.623573200068682142E-15 ) ) ;
#37080=LINE ( 'NONE', #21276, #6388 ) ;
#37081=EDGE_CURVE ( 'NONE', #10127, #41143, #13251, .T. ) ;
#37086=ORIENTED_EDGE ( 'NONE', *, *, #41075, .T. ) ;
#37094=DIRECTION ( 'NONE',  ( 0.4849315768086534528, 0.8745520943968249084, 1.030032898892974818E-16 ) ) ;
#37098=EDGE_CURVE ( 'NONE', #2129, #22153, #11381, .T. ) ;
#37106=EDGE_LOOP ( 'NONE', ( #6935, #2903, #23230, #28967 ) ) ;
#37107=EDGE_LOOP ( 'NONE', ( #28022, #2261, #24954, #1034 ) ) ;
#37120=CARTESIAN_POINT ( 'NONE',  ( -57.97024931889899335, 0.5691613924951877124, 0.8993266954188116058 ) ) ;
#37125=EDGE_CURVE ( 'NONE', #26682, #13736, #20224, .T. ) ;
#37129=EDGE_CURVE ( 'NONE', #37552, #35632, #4607, .T. ) ;
#37130=CARTESIAN_POINT ( 'NONE',  ( -57.85534701229749999, 0.8496279762696401505, -1.203237356453227491 ) ) ;
#37133=CARTESIAN_POINT ( 'NONE',  ( -46.89253820722738908, 25.40240703814324164, -1.700804414715234580 ) ) ;
#37135=CARTESIAN_POINT ( 'NONE',  ( -31.58045816364236202, 52.93464387108262059, -1.524000000000004906 ) ) ;
#37137=CARTESIAN_POINT ( 'NONE',  ( -8.594951744493888768, 74.76616009375631222, -1.523999999999996913 ) ) ;
#37139=CARTESIAN_POINT ( 'NONE',  ( -57.92935616279446265, 2.416188466839983118, 0.2259612492381935789 ) ) ;
#37143=CARTESIAN_POINT ( 'NONE',  ( -57.42300747107054093, 3.318281940618617032, -1.876676483338179491 ) ) ;
#37145=CARTESIAN_POINT ( 'NONE',  ( -45.60639265695031952, 20.98815520443264404, -4.238054969593709309 ) ) ;
#37152=CARTESIAN_POINT ( 'NONE',  ( -49.56431242325176356, 16.98212490189121127, -5.014837167102403015 ) ) ;
#37154=CIRCLE ( 'NONE', #3844, 0.2540000000000000591 ) ;
#37157=CARTESIAN_POINT ( 'NONE',  ( -58.19031870555688357, 0.09256663605368072034, -0.5720079524431537221 ) ) ;
#37161=CARTESIAN_POINT ( 'NONE',  ( -47.16890147375937659, 22.20336809214646578, -4.187060126831891438 ) ) ;
#37165=ORIENTED_EDGE ( 'NONE', *, *, #37062, .T. ) ;
#37170=CARTESIAN_POINT ( 'NONE',  ( -52.42133349025997546, 11.92692459785933679, -4.172736198742198255 ) ) ;
#37175=ADVANCED_FACE ( 'NONE', ( #20252 ), #1115, .F. ) ;
#37180=CARTESIAN_POINT ( 'NONE',  ( -45.90302585792993284, 20.78970012321159899, -4.334318749026735418 ) ) ;
#37181=DIRECTION ( 'NONE',  ( -0.8745520943968235761, 0.4849315768086558953, -5.361993529360570985E-16 ) ) ;
#37182=CARTESIAN_POINT ( 'NONE',  ( -57.37715403173692152, 1.618736692213004869, 0.5106765013061003167 ) ) ;
#37184=ORIENTED_EDGE ( 'NONE', *, *, #32083, .F. ) ;
#37185=CARTESIAN_POINT ( 'NONE',  ( -47.31580374228550312, 25.16323110364244897, -0.6294670755810810592 ) ) ;
#37188=VERTEX_POINT ( 'NONE', #33278 ) ;
#37193=AXIS2_PLACEMENT_3D ( 'NONE', #9598, #16183, #6415 ) ;
#37200=CARTESIAN_POINT ( 'NONE',  ( -41.41133299024001246, 23.09032428891222111, -1.527002492031612979 ) ) ;
#37207=CARTESIAN_POINT ( 'NONE',  ( -58.82991071597902533, -0.2577532384650527142, -9.114074148744775817E-15 ) ) ;
#37213=ORIENTED_EDGE ( 'NONE', *, *, #27356, .F. ) ;
#37214=TOROIDAL_SURFACE ( 'NONE', #28364, 0.3809999999999990616, 0.2540000000000000036 ) ;
#37217=CARTESIAN_POINT ( 'NONE',  ( -18.88649316419433788, 79.99958772249931371, 1.269999999999996021 ) ) ;
#37219=VERTEX_POINT ( 'NONE', #701 ) ;
#37230=CARTESIAN_POINT ( 'NONE',  ( -52.99508395989393250, 10.78319250833652809, 3.865765426181710041 ) ) ;
#37231=DIRECTION ( 'NONE',  ( 0.8745520943968235761, -0.4849315768086558398, 4.268512490100410909E-16 ) ) ;
#37232=CARTESIAN_POINT ( 'NONE',  ( -58.60752282809816904, -0.1920500713008393978, 0.6598870774482750168 ) ) ;
#37233=CARTESIAN_POINT ( 'NONE',  ( -58.61247718564857223, -0.2580816525627335767, 0.4259738903449781788 ) ) ;
#37237=ORIENTED_EDGE ( 'NONE', *, *, #33876, .F. ) ;
#37238=CARTESIAN_POINT ( 'NONE',  ( -53.65759266121656879, 11.01975743955735432, 4.003319250743206936 ) ) ;
#37244=DIRECTION ( 'NONE',  ( 0.7770581983690878491, -0.6294287539883980376, 5.101669463485847584E-16 ) ) ;
#37245=ORIENTED_EDGE ( 'NONE', *, *, #39652, .T. ) ;
#37249=CARTESIAN_POINT ( 'NONE',  ( -46.82131867383161961, 20.47688106639223449, 5.000304862135632966 ) ) ;
#37252=CARTESIAN_POINT ( 'NONE',  ( -8.519412162535125788, 69.40335734044577976, 1.524000000000003352 ) ) ;
#37261=ORIENTED_EDGE ( 'NONE', *, *, #21654, .T. ) ;
#37262=CARTESIAN_POINT ( 'NONE',  ( -52.57757236033170045, 11.11936768914174145, 3.180765541460421897 ) ) ;
#37266=EDGE_LOOP ( 'NONE', ( #40354, #34079, #34537, #20842 ) ) ;
#37269=DIRECTION ( 'NONE',  ( 0.8745520943968253524, -0.4849315768086530087, 8.537024980200771528E-16 ) ) ;
#37271=ORIENTED_EDGE ( 'NONE', *, *, #34710, .T. ) ;
#37278=CARTESIAN_POINT ( 'NONE',  ( -10.00099186598785650, 77.19260062651656540, 1.524000000000000465 ) ) ;
#37281=CARTESIAN_POINT ( 'NONE',  ( -14.21338345945963688, 79.68069512491149453, 1.269999999999998241 ) ) ;
#37282=EDGE_CURVE ( 'NONE', #10652, #25646, #26663, .T. ) ;
#37299=EDGE_CURVE ( 'NONE', #38754, #37322, #16137, .T. ) ;
#37301=VERTEX_POINT ( 'NONE', #23443 ) ;
#37306=ADVANCED_FACE ( 'NONE', ( #29653 ), #20462, .T. ) ;
#37307=VERTEX_POINT ( 'NONE', #30274 ) ;
#37309=LINE ( 'NONE', #34124, #1135 ) ;
#37313=EDGE_CURVE ( 'NONE', #915, #12580, #14284, .T. ) ;
#37318=EDGE_CURVE ( 'NONE', #40156, #22433, #908, .T. ) ;
#37322=VERTEX_POINT ( 'NONE', #11101 ) ;
#37324=AXIS2_PLACEMENT_3D ( 'NONE', #27542, #18145, #40131 ) ;
#37327=CARTESIAN_POINT ( 'NONE',  ( -52.95179419874582294, 11.24610246599371699, 4.133922171299013293 ) ) ;
#37335=CARTESIAN_POINT ( 'NONE',  ( -57.23135758994266098, 1.814875683430833275, -0.2588789259697646394 ) ) ;
#37338=DIRECTION ( 'NONE',  ( 5.188838149069472160E-16, -1.699382548006136559E-16, -1.000000000000000000 ) ) ;
#37339=DIRECTION ( 'NONE',  ( 5.188838149069472160E-16, -1.699382548006136559E-16, -1.000000000000000000 ) ) ;
#37342=DIRECTION ( 'NONE',  ( 5.188838149069472160E-16, -1.699382548006136559E-16, -1.000000000000000000 ) ) ;
#37343=DIRECTION ( 'NONE',  ( -0.8745520943968241312, 0.4849315768086547851, -5.271987356194193006E-16 ) ) ;
#37346=EDGE_CURVE ( 'NONE', #37301, #16441, #37940, .T. ) ;
#37348=CARTESIAN_POINT ( 'NONE',  ( -58.83227707057486811, -0.08366279997996939333, -5.839471642284167958E-15 ) ) ;
#37349=AXIS2_PLACEMENT_3D ( 'NONE', #5244, #31418, #30782 ) ;
#37350=EDGE_CURVE ( 'NONE', #1503, #915, #7994, .T. ) ;
#37352=CARTESIAN_POINT ( 'NONE',  ( -47.34495446287286313, 19.93462121980824620, -5.151308439895126767 ) ) ;
#37359=CARTESIAN_POINT ( 'NONE',  ( -49.47195631129834226, 17.12452434303404303, -5.032791565054547611 ) ) ;
#37360=FACE_OUTER_BOUND ( 'NONE', #35070, .T. ) ;
#37362=CARTESIAN_POINT ( 'NONE',  ( -50.95832625531466675, 14.53658918554379298, -4.553647182183382824 ) ) ;
#37363=EDGE_CURVE ( 'NONE', #29093, #25607, #23661, .T. ) ;
#37366=CARTESIAN_POINT ( 'NONE',  ( -46.81005371095109524, 25.73327194510133253, -1.583310528698488984 ) ) ;
#37372=EDGE_CURVE ( 'NONE', #31966, #2670, #22851, .T. ) ;
#37374=CARTESIAN_POINT ( 'NONE',  ( -57.93941708942283952, 2.052042089854988483, -1.628789306319529118 ) ) ;
#37378=AXIS2_PLACEMENT_3D ( 'NONE', #23983, #14601, #7397 ) ;
#37379=VECTOR ( 'NONE', #35154, 1000.000000000000000 ) ;
#37384=CARTESIAN_POINT ( 'NONE',  ( -41.38112080847943020, 22.74200708568027807, -0.4658591655019068689 ) ) ;
#37387=CARTESIAN_POINT ( 'NONE',  ( -57.47393550255003447, 1.325481720219581661, -1.009526220810559183E-14 ) ) ;
#37389=VERTEX_POINT ( 'NONE', #30483 ) ;
#37390=CARTESIAN_POINT ( 'NONE',  ( -47.23483502501005660, 23.02499599010462816, -3.263444997004429915 ) ) ;
#37403=DIRECTION ( 'NONE',  ( -5.188838149069471174E-16, 1.699382548006136313E-16, 1.000000000000000000 ) ) ;
#37406=DIRECTION ( 'NONE',  ( -0.7548010569845216011, -0.6559537821943317581, -2.801824109679581255E-16 ) ) ;
#37407=EDGE_LOOP ( 'NONE', ( #5141, #19428, #11907, #27313 ) ) ;
#37409=CARTESIAN_POINT ( 'NONE',  ( -17.76856900107737403, 61.81127730225986738, 1.523999999999999133 ) ) ;
#37411=CARTESIAN_POINT ( 'NONE',  ( -58.45128286774109938, -0.4309378487381305689, -0.3205346425646805053 ) ) ;
#37416=EDGE_CURVE ( 'NONE', #36699, #35463, #24234, .T. ) ;
#37431=CARTESIAN_POINT ( 'NONE',  ( -58.36702958454534951, -0.2857891562030455135, 0.06428893395075664652 ) ) ;
#37433=CARTESIAN_POINT ( 'NONE',  ( -51.04345146481078643, 14.57989528305921745, 4.679979037057004909 ) ) ;
#37438=CARTESIAN_POINT ( 'NONE',  ( -53.17586183559576085, 10.67386474145934372, 4.017225210190868978 ) ) ;
#37444=AXIS2_PLACEMENT_3D ( 'NONE', #31063, #27867, #37672 ) ;
#37449=CARTESIAN_POINT ( 'NONE',  ( -5.591489108514605455, 77.73497692594764885, -1.269999999999996021 ) ) ;
#37450=CARTESIAN_POINT ( 'NONE',  ( -43.40712238249599864, 21.47926646521387184, 2.288489392298276748 ) ) ;
#37451=CARTESIAN_POINT ( 'NONE',  ( -41.05193670661653726, 23.09446788613699653, 1.270000000071882518 ) ) ;
#37463=ORIENTED_EDGE ( 'NONE', *, *, #23687, .T. ) ;
#37464=CARTESIAN_POINT ( 'NONE',  ( -51.42025106686629243, 13.11195823927271320, 3.453838694686329536 ) ) ;
#37468=ORIENTED_EDGE ( 'NONE', *, *, #2742, .T. ) ;
#37475=FACE_OUTER_BOUND ( 'NONE', #7213, .T. ) ;
#37478=CARTESIAN_POINT ( 'NONE',  ( -28.09515292912719175, 77.51021392068167870, 1.523999999999992028 ) ) ;
#37480=DIRECTION ( 'NONE',  ( -0.4849315768086481238, -0.8745520943968281280, 8.647447314816545091E-15 ) ) ;
#37484=DIRECTION ( 'NONE',  ( 0.6294287539884059202, 0.7770581983690814099, 1.945484789722797322E-16 ) ) ;
#37486=ORIENTED_EDGE ( 'NONE', *, *, #1206, .F. ) ;
#37496=CARTESIAN_POINT ( 'NONE',  ( -57.43227285409300009, 3.226759729073131133, 2.064049688025078488 ) ) ;
#37503=EDGE_LOOP ( 'NONE', ( #22307, #23162, #29506, #347, #1471, #23186 ) ) ;
#37504=DIRECTION ( 'NONE',  ( -0.7308269722843343530, 0.6825627711659295604, -8.537024980200805055E-16 ) ) ;
#37511=VERTEX_POINT ( 'NONE', #31317 ) ;
#37513=FACE_OUTER_BOUND ( 'NONE', #34187, .T. ) ;
#37521=DIRECTION ( 'NONE',  ( 5.188838149069472160E-16, -1.699382548006136559E-16, -1.000000000000000000 ) ) ;
#37524=EDGE_LOOP ( 'NONE', ( #36854, #8329, #28858, #27790 ) ) ;
#37528=CARTESIAN_POINT ( 'NONE',  ( -57.70126415073575998, 1.705439686548140710, 1.647193596431507645 ) ) ;
#37534=AXIS2_PLACEMENT_3D ( 'NONE', #27635, #2305, #16050 ) ;
#37540=CARTESIAN_POINT ( 'NONE',  ( -57.28860081656939229, 2.041040056096066202, -1.590330371070468152 ) ) ;
#37543=CARTESIAN_POINT ( 'NONE',  ( -8.313969523394650452, 67.96940778435646280, -1.269999999999995577 ) ) ;
#37544=DIRECTION ( 'NONE',  ( 0.2883665106726583938, 0.9575201071113210727, 0.000000000000000000 ) ) ;
#37545=LINE ( 'NONE', #40551, #18154 ) ;
#37552=VERTEX_POINT ( 'NONE', #6395 ) ;
#37553=CARTESIAN_POINT ( 'NONE',  ( -58.66661043166477896, 0.3408866871785626307, -0.5032371457779314383 ) ) ;
#37555=CYLINDRICAL_SURFACE ( 'NONE', #40330, 0.2539999999999996150 ) ;
#37562=CARTESIAN_POINT ( 'NONE',  ( -52.44660108373793150, 12.13357835523497563, -4.279154699026443964 ) ) ;
#37563=ORIENTED_EDGE ( 'NONE', *, *, #26671, .T. ) ;
#37567=CARTESIAN_POINT ( 'NONE',  ( -19.97113776634630256, 79.44829951959813741, -1.270000000000003570 ) ) ;
#37570=CARTESIAN_POINT ( 'NONE',  ( -54.39768377094780760, 8.094885465611476150, -3.421923752996840928 ) ) ;
#37571=AXIS2_PLACEMENT_3D ( 'NONE', #36044, #29647, #58 ) ;
#37578=CARTESIAN_POINT ( 'NONE',  ( -58.09657527255103560, 0.9821181129459344294, -1.359330230256445393 ) ) ;
#37579=CIRCLE ( 'NONE', #18537, 3.111499999999999932 ) ;
#37582=ADVANCED_FACE ( 'NONE', ( #15548 ), #12366, .T. ) ;
#37583=DIRECTION ( 'NONE',  ( -5.188838149069472160E-16, 1.699382548006136559E-16, 1.000000000000000000 ) ) ;
#37586=CARTESIAN_POINT ( 'NONE',  ( -54.34142964503966056, 9.837102586603037935, -3.694930414371515148 ) ) ;
#37588=CARTESIAN_POINT ( 'NONE',  ( -44.16391282238571847, 20.57229585060895616, -1.749602973179261944 ) ) ;
#37594=CARTESIAN_POINT ( 'NONE',  ( -57.63883995378735392, 1.113466886629776997, 0.4249547484444501921 ) ) ;
#37595=CARTESIAN_POINT ( 'NONE',  ( -51.38196307734524737, 20.99359796827592817, 0.3730309213897141096 ) ) ;
#37598=CARTESIAN_POINT ( 'NONE',  ( -48.33886291794431145, 23.55519408767752054, -1.110521498696447118 ) ) ;
#37607=CIRCLE ( 'NONE', #24004, 0.3810000000000030584 ) ;
#37613=CARTESIAN_POINT ( 'NONE',  ( -46.85406971281315691, 20.44882436048083818, -5.016006885995599518 ) ) ;
#37615=CARTESIAN_POINT ( 'NONE',  ( -38.65395868481546415, 29.38327706004843876, 1.523999999999994470 ) ) ;
#37616=ADVANCED_FACE ( 'NONE', ( #32371 ), #33111, .T. ) ;
#37622=CARTESIAN_POINT ( 'NONE',  ( -58.49146960918327665, -0.5079027975582817156, -0.2843517202595862714 ) ) ;
#37628=ORIENTED_EDGE ( 'NONE', *, *, #2742, .F. ) ;
#37633=DIRECTION ( 'NONE',  ( 0.1565721916418034432, 0.9876665170007953298, -8.659954811667511346E-17 ) ) ;
#37637=ORIENTED_EDGE ( 'NONE', *, *, #20329, .F. ) ;
#37639=CARTESIAN_POINT ( 'NONE',  ( -28.60507221318228943, 76.72702915747851193, -1.270000000000007567 ) ) ;
#37649=CARTESIAN_POINT ( 'NONE',  ( -58.18051401232126807, 0.1137601867684435997, 0.5894366672358869463 ) ) ;
#37655=VERTEX_POINT ( 'NONE', #17016 ) ;
#37656=CARTESIAN_POINT ( 'NONE',  ( -48.82738941085167284, 18.57305038084609095, 5.399437279161905856 ) ) ;
#37661=CARTESIAN_POINT ( 'NONE',  ( -23.14542444889682216, 82.37908244650444090, -1.270000000000005791 ) ) ;
#37665=CARTESIAN_POINT ( 'NONE',  ( -30.03238267980982457, 57.98137616137810824, 1.524000000000849564 ) ) ;
#37668=DIRECTION ( 'NONE',  ( -0.7770581983690836303, 0.6294287539884032556, -5.101669463485833779E-16 ) ) ;
#37672=DIRECTION ( 'NONE',  ( -0.8745520943968243532, 0.4849315768086547296, -5.361993529360573944E-16 ) ) ;
#37678=AXIS2_PLACEMENT_3D ( 'NONE', #17879, #14681, #11490 ) ;
#37680=ORIENTED_EDGE ( 'NONE', *, *, #13898, .F. ) ;
#37681=CARTESIAN_POINT ( 'NONE',  ( -56.36488200494262202, 4.056002992322685685, 2.423683632884268579 ) ) ;
#37687=ORIENTED_EDGE ( 'NONE', *, *, #18824, .T. ) ;
#37691=VERTEX_POINT ( 'NONE', #10837 ) ;
#37694=VECTOR ( 'NONE', #34520, 1000.000000000000000 ) ;
#37695=LINE ( 'NONE', #31290, #34766 ) ;
#37701=CARTESIAN_POINT ( 'NONE',  ( -36.79765817521327165, 27.64956762128695900, 1.269999999999994689 ) ) ;
#37712=CARTESIAN_POINT ( 'NONE',  ( -58.33777482027512207, 1.113448835244237767, 1.208045587469420701 ) ) ;
#37713=FACE_OUTER_BOUND ( 'NONE', #10230, .T. ) ;
#37716=CARTESIAN_POINT ( 'NONE',  ( -24.46582648842863961, 82.15028593570633575, -1.270000000000006679 ) ) ;
#37721=VERTEX_POINT ( 'NONE', #7031 ) ;
#37733=CARTESIAN_POINT ( 'NONE',  ( -43.26072228752227744, 21.85338980287131605, 2.263362209153686244 ) ) ;
#37744=CARTESIAN_POINT ( 'NONE',  ( -58.62884620442479644, -0.7615560826029293962, 0.07633319197526360067 ) ) ;
#37752=CARTESIAN_POINT ( 'NONE',  ( -57.38720131040756200, 1.641502911523470942, -0.7119259365333358014 ) ) ;
#37756=FACE_OUTER_BOUND ( 'NONE', #2598, .T. ) ;
#37759=CARTESIAN_POINT ( 'NONE',  ( -19.33375693323417366, 80.42273151551299293, 1.269999999999995577 ) ) ;
#37760=CARTESIAN_POINT ( 'NONE',  ( -58.83227707057486811, -0.08366279997996939333, -1.539018077965326743E-14 ) ) ;
#37764=CARTESIAN_POINT ( 'NONE',  ( -58.64217253742437208, 0.4108157498741576985, -0.3978973257256673279 ) ) ;
#37766=CARTESIAN_POINT ( 'NONE',  ( -47.20408514806585742, 20.03888983422004344, -5.082056583519131365 ) ) ;
#37773=CARTESIAN_POINT ( 'NONE',  ( -50.06326276805182118, 16.19468026859921039, -4.911295769374709685 ) ) ;
#37774=EDGE_LOOP ( 'NONE', ( #33998, #12134, #41568, #26662 ) ) ;
#37776=FACE_OUTER_BOUND ( 'NONE', #37106, .T. ) ;
#37779=CARTESIAN_POINT ( 'NONE',  ( -53.97752642499204967, 8.868598658150437686, -3.466679480857036477 ) ) ;
#37782=CARTESIAN_POINT ( 'NONE',  ( -52.97391985390434144, 12.30611266682019789, -4.247241762254921227 ) ) ;
#37787=DIRECTION ( 'NONE',  ( -5.188838149069471174E-16, 1.699382548006136313E-16, 1.000000000000000000 ) ) ;
#37788=CARTESIAN_POINT ( 'NONE',  ( -58.03414100541874632, 0.4564111095344686175, -0.9708715263941700702 ) ) ;
#37792=EDGE_CURVE ( 'NONE', #22227, #41583, #11325, .T. ) ;
#37795=DIRECTION ( 'NONE',  ( -0.7770581983690878491, 0.6294287539883980376, -5.101669463485847584E-16 ) ) ;
#37796=CARTESIAN_POINT ( 'NONE',  ( -44.09535491252989203, 20.89266065238331294, -2.220044762595793753 ) ) ;
#37799=FACE_OUTER_BOUND ( 'NONE', #33215, .T. ) ;
#37800=LINE ( 'NONE', #34618, #13339 ) ;
#37801=CARTESIAN_POINT ( 'NONE',  ( -50.73416975447392474, 21.22185706673585059, 0.7846160747444976824 ) ) ;
#37806=CARTESIAN_POINT ( 'NONE',  ( -50.57586884603683330, 21.47051451305503988, -0.7809936997224710131 ) ) ;
#37817=DIRECTION ( 'NONE',  ( -0.4849315768086534528, -0.8745520943968250194, -1.030032898892974942E-16 ) ) ;
#37820=CARTESIAN_POINT ( 'NONE',  ( -41.08171237912073792, 23.06270199366203855, -1.270028482463944064 ) ) ;
#37821=DIRECTION ( 'NONE',  ( -0.8745520943968225769, 0.4849315768086576717, -5.691349986800551823E-16 ) ) ;
#37823=ORIENTED_EDGE ( 'NONE', *, *, #6349, .T. ) ;
#37827=CARTESIAN_POINT ( 'NONE',  ( -57.83370854706699760, 0.8645507274500918715, -1.063039573801316307 ) ) ;
#37834=EDGE_LOOP ( 'NONE', ( #27445, #39843, #29519, #6010 ) ) ;
#37837=EDGE_CURVE ( 'NONE', #5531, #10519, #14859, .T. ) ;
#37840=EDGE_CURVE ( 'NONE', #11774, #5717, #17849, .T. ) ;
#37841=AXIS2_PLACEMENT_3D ( 'NONE', #34957, #38769, #22549 ) ;
#37842=LINE ( 'NONE', #21627, #32201 ) ;
#37848=DIRECTION ( 'NONE',  ( -0.8745520943968235761, 0.4849315768086558398, -4.268512490100410909E-16 ) ) ;
#37856=CARTESIAN_POINT ( 'NONE',  ( -58.17408770762806114, 0.1276510453498960473, 0.6006340682012513144 ) ) ;
#37857=CARTESIAN_POINT ( 'NONE',  ( -32.35164496306255444, 51.35586489404142441, -1.524000000000005794 ) ) ;
#37858=DIRECTION ( 'NONE',  ( -0.6294287539884133587, -0.7770581983690755257, 0.000000000000000000 ) ) ;
#37862=CARTESIAN_POINT ( 'NONE',  ( -51.02479983779974049, 14.46739584830851477, 4.600955224801048793 ) ) ;
#37868=ORIENTED_EDGE ( 'NONE', *, *, #564, .T. ) ;
#37871=DIRECTION ( 'NONE',  ( -0.8745520943968240202, 0.4849315768086553402, -5.361993529360572958E-16 ) ) ;
#37872=CARTESIAN_POINT ( 'NONE',  ( -42.18235783619532953, 22.15054559413689006, 1.778153187293267434 ) ) ;
#37875=CARTESIAN_POINT ( 'NONE',  ( -48.24242213954391900, 19.61027420771482355, 5.299259492517840009 ) ) ;
#37887=CARTESIAN_POINT ( 'NONE',  ( -56.89722832398061314, 2.603431824206650536, 0.9028745487782365853 ) ) ;
#37892=CIRCLE ( 'NONE', #41981, 0.5080000000000000071 ) ;
#37894=AXIS2_PLACEMENT_3D ( 'NONE', #5683, #9484, #31646 ) ;
#37895=ADVANCED_FACE ( 'NONE', ( #31264 ), #6559, .T. ) ;
#37898=ORIENTED_EDGE ( 'NONE', *, *, #36293, .F. ) ;
#37901=CIRCLE ( 'NONE', #35876, 0.7620000000000000107 ) ;
#37908=DIRECTION ( 'NONE',  ( -0.8745520943968251304, 0.4849315768086535638, 5.226292508699495262E-15 ) ) ;
#37913=CARTESIAN_POINT ( 'NONE',  ( -23.69188486464780752, 78.08202335040543574, -1.524000000000005350 ) ) ;
#37919=AXIS2_PLACEMENT_3D ( 'NONE', #16762, #39793, #23565 ) ;
#37920=CARTESIAN_POINT ( 'NONE',  ( -17.14500000000466784, 71.11999999999886768, -1.524000000000000909 ) ) ;
#37938=EDGE_LOOP ( 'NONE', ( #88, #3359, #40922, #2680 ) ) ;
#37940=CIRCLE ( 'NONE', #26347, 0.7620000000000015650 ) ;
#37944=DIRECTION ( 'NONE',  ( 5.188838149069472160E-16, -1.699382548006136559E-16, -1.000000000000000000 ) ) ;
#37945=EDGE_CURVE ( 'NONE', #1503, #5200, #11889, .T. ) ;
#37949=FACE_OUTER_BOUND ( 'NONE', #636, .T. ) ;
#37950=EDGE_CURVE ( 'NONE', #12622, #38820, #33416, .T. ) ;
#37959=CARTESIAN_POINT ( 'NONE',  ( -58.44555280191302415, -0.4200408777295304152, 0.3231375529342178643 ) ) ;
#37967=CARTESIAN_POINT ( 'NONE',  ( -57.43023524350843445, 1.739013888464230329, -1.477089945056109910 ) ) ;
#37970=DIRECTION ( 'NONE',  ( -0.8745520943968250194, 0.4849315768086534528, -5.361993529360573944E-16 ) ) ;
#37979=EDGE_LOOP ( 'NONE', ( #4290, #37637, #19720, #5971 ) ) ;
#37980=CARTESIAN_POINT ( 'NONE',  ( -58.03428750496626520, 2.144022121626010247, -1.074202927763570110E-14 ) ) ;
#37982=DIRECTION ( 'NONE',  ( 5.188838149069472160E-16, -1.699382548006136559E-16, -1.000000000000000000 ) ) ;
#37986=PRODUCT_DEFINITION_FORMATION_WITH_SPECIFIED_SOURCE ( 'ANY', '', #29310, .NOT_KNOWN. ) ;
#37990=CARTESIAN_POINT ( 'NONE',  ( -57.26545915665239050, 2.636046494217942016, -1.996990251079107770 ) ) ;
#37995=CARTESIAN_POINT ( 'NONE',  ( -50.47963954645450713, 15.37956391664342171, -4.696064106192690879 ) ) ;
#37998=CARTESIAN_POINT ( 'NONE',  ( -54.32300027520380326, 9.724537220608771904, -3.743864951777645445 ) ) ;
#38000=EDGE_CURVE ( 'NONE', #3009, #4929, #11672, .T. ) ;
#38007=CARTESIAN_POINT ( 'NONE',  ( -57.71946847630993460, 1.146847591362354368, -1.351507486235954403 ) ) ;
#38010=CARTESIAN_POINT ( 'NONE',  ( -11.67683074431529988, 78.22376516830392745, 1.270000000000000018 ) ) ;
#38013=CARTESIAN_POINT ( 'NONE',  ( -57.80205714066466527, 2.371715784325115095, -1.753227392946310470 ) ) ;
#38014=CIRCLE ( 'NONE', #15535, 0.2540000000000000036 ) ;
#38015=CARTESIAN_POINT ( 'NONE',  ( -41.05189575270515689, 23.09451173561988924, -0.6632222222222277086 ) ) ;
#38016=ORIENTED_EDGE ( 'NONE', *, *, #37945, .T. ) ;
#38017=CARTESIAN_POINT ( 'NONE',  ( -17.64290547347870941, 83.78857423953914463, 1.523999999999996247 ) ) ;
#38018=DIRECTION ( 'NONE',  ( 0.6825627711659461028, 0.7308269722843185878, 2.299753143848302396E-16 ) ) ;
#38021=CARTESIAN_POINT ( 'NONE',  ( -50.95401363114979176, 21.69085172357045010, -9.625367201313238999E-15 ) ) ;
#38024=CARTESIAN_POINT ( 'NONE',  ( -49.85168879002940656, 22.56840098298264152, -0.7122439767497329433 ) ) ;
#38033=CARTESIAN_POINT ( 'NONE',  ( -3.841520934845505941, 71.62889921741444255, -1.523999999999994026 ) ) ;
#38039=CARTESIAN_POINT ( 'NONE',  ( -44.39753738666030358, 21.50835220694079197, -3.136200265191924075 ) ) ;
#38040=EDGE_CURVE ( 'NONE', #20172, #11776, #27824, .T. ) ;
#38041=DIRECTION ( 'NONE',  ( -0.8745520943968243532, 0.4849315768086547296, -5.361993529360573944E-16 ) ) ;
#38044=CARTESIAN_POINT ( 'NONE',  ( -17.31000046771894318, 62.32679794340116786, 1.269999999999999574 ) ) ;
#38050=EDGE_CURVE ( 'NONE', #25107, #17471, #22190, .T. ) ;
#38054=CIRCLE ( 'NONE', #15573, 2.539999999999996483 ) ;
#38056=VECTOR ( 'NONE', #4518, 1000.000000000000000 ) ;
#38058=CARTESIAN_POINT ( 'NONE',  ( -43.82859865241511699, 24.63416949198730421, -1.524000000000007127 ) ) ;
#38071=CARTESIAN_POINT ( 'NONE',  ( -58.21877897856138873, 0.03104753578543094361, 0.5212065818953967034 ) ) ;
#38075=VECTOR ( 'NONE', #6316, 1000.000000000000114 ) ;
#38079=CARTESIAN_POINT ( 'NONE',  ( -47.71508057896579658, 20.49549959222711593, 5.111566084959459744 ) ) ;
#38080=AXIS2_PLACEMENT_3D ( 'NONE', #39997, #30797, #23560 ) ;
#38085=DIRECTION ( 'NONE',  ( -0.8572391118119511155, -0.5149185422762101449, -3.573031421855331076E-16 ) ) ;
#38086=EDGE_CURVE ( 'NONE', #25039, #6518, #5104, .T. ) ;
#38092=DIRECTION ( 'NONE',  ( -5.188838149069472160E-16, 1.699382548006136559E-16, 1.000000000000000000 ) ) ;
#38096=CARTESIAN_POINT ( 'NONE',  ( -23.91048590848665611, 81.84235438443283783, -1.270000000000006235 ) ) ;
#38103=ORIENTED_EDGE ( 'NONE', *, *, #5598, .F. ) ;
#38104=CARTESIAN_POINT ( 'NONE',  ( -57.40070531792823516, 1.672101763895803117, 0.9705777051857996662 ) ) ;
#38110=ORIENTED_EDGE ( 'NONE', *, *, #12017, .F. ) ;
#38120=DIRECTION ( 'NONE',  ( 0.9998501190848634312, 0.01731298258488012456, 8.537024980200823790E-16 ) ) ;
#38122=FACE_OUTER_BOUND ( 'NONE', #19081, .T. ) ;
#38123=VECTOR ( 'NONE', #7721, 1000.000000000000000 ) ;
#38125=CARTESIAN_POINT ( 'NONE',  ( -46.25688858429102623, 20.73875112231587892, 4.700046123029338219 ) ) ;
#38128=ORIENTED_EDGE ( 'NONE', *, *, #8199, .F. ) ;
#38129=ORIENTED_EDGE ( 'NONE', *, *, #37837, .T. ) ;
#38131=EDGE_CURVE ( 'NONE', #15145, #24767, #8596, .T. ) ;
#38134=CIRCLE ( 'NONE', #21780, 0.7620000000000000107 ) ;
#38136=CARTESIAN_POINT ( 'NONE',  ( -46.60530155212502734, 26.17382724835478314, -1.397000000000007791 ) ) ;
#38139=EDGE_CURVE ( 'NONE', #6464, #40376, #16053, .T. ) ;
#38140=CARTESIAN_POINT ( 'NONE',  ( -54.50298212578950796, 9.515077312548310573, 3.630897911711898018 ) ) ;
#38141=DIRECTION ( 'NONE',  ( 5.188838149069472160E-16, -1.699382548006136559E-16, -1.000000000000000000 ) ) ;
#38146=CARTESIAN_POINT ( 'NONE',  ( -17.14500000000466784, 71.11999999999886768, 1.269999999999998241 ) ) ;
#38158=CARTESIAN_POINT ( 'NONE',  ( -41.05189575270519242, 23.09451173561983239, -4.677211348804838536E-15 ) ) ;
#38166=CARTESIAN_POINT ( 'NONE',  ( -5.639506490940112471, 64.42185452804264401, 1.270000000000004681 ) ) ;
#38171=VERTEX_POINT ( 'NONE', #9327 ) ;
#38173=DIRECTION ( 'NONE',  ( 5.188838149069472160E-16, -1.699382548006136559E-16, -1.000000000000000000 ) ) ;
#38176=CARTESIAN_POINT ( 'NONE',  ( -47.85244527695893879, 19.39403540832956807, 5.219971639306655753 ) ) ;
#38187=FACE_OUTER_BOUND ( 'NONE', #10847, .T. ) ;
#38191=EDGE_CURVE ( 'NONE', #915, #3540, #32322, .T. ) ;
#38194=CARTESIAN_POINT ( 'NONE',  ( -17.14500000000466784, 71.11999999999886768, -1.270000000000000684 ) ) ;
#38198=CARTESIAN_POINT ( 'NONE',  ( -58.80872392184672037, -0.02106340533553074934, -0.1867271868312316840 ) ) ;
#38200=DIRECTION ( 'NONE',  ( 0.8745520943968235761, -0.4849315768086558398, 0.000000000000000000 ) ) ;
#38201=CIRCLE ( 'NONE', #19808, 0.2539999999999956737 ) ;
#38208=CARTESIAN_POINT ( 'NONE',  ( -57.72754330036800496, 1.649358777147267752, -1.624819368011742204 ) ) ;
#38215=AXIS2_PLACEMENT_3D ( 'NONE', #10091, #26275, #13075 ) ;
#38217=CARTESIAN_POINT ( 'NONE',  ( -55.03109054507046238, 6.816801101491506643, -3.135084751894932076 ) ) ;
#38225=CARTESIAN_POINT ( 'NONE',  ( -58.50860430493789721, 0.7049166599848305514, -0.9756837515128595761 ) ) ;
#38229=CARTESIAN_POINT ( 'NONE',  ( -47.06702646257116385, 25.34112732371118781, 1.513569369951779597 ) ) ;
#38232=CARTESIAN_POINT ( 'NONE',  ( -48.28978369826177186, 19.63653578263564015, -5.206999999995405304 ) ) ;
#38233=CARTESIAN_POINT ( 'NONE',  ( -41.05189575270517111, 23.09451173561986081, -1.397000000000004238 ) ) ;
#38236=CARTESIAN_POINT ( 'NONE',  ( -57.71946847630993460, 1.146847591362354368, 1.351507486235933975 ) ) ;
#38237=CARTESIAN_POINT ( 'NONE',  ( -53.84463291498614268, 9.545084226694347862, 3.785192793386291665 ) ) ;
#38240=CARTESIAN_POINT ( 'NONE',  ( -51.90232906080404263, 16.51944673254565643, 2.845700375512744795 ) ) ;
#38243=CARTESIAN_POINT ( 'NONE',  ( -48.35471193741586404, 22.70554656608007704, -1.835820227619855416 ) ) ;
#38251=CARTESIAN_POINT ( 'NONE',  ( -26.07365872405947727, 72.73903180058835005, -1.270000000000005791 ) ) ;
#38252=VECTOR ( 'NONE', #34576, 1000.000000000000114 ) ;
#38258=DIRECTION ( 'NONE',  ( -0.8745520943968235761, 0.4849315768086558398, 0.000000000000000000 ) ) ;
#38259=DIRECTION ( 'NONE',  ( -0.6559537821943243197, 0.7548010569845282625, -8.537024980200743918E-16 ) ) ;
#38262=CARTESIAN_POINT ( 'NONE',  ( -23.75665686005077859, 76.91945007112674659, 1.269999999999994245 ) ) ;
#38279=AXIS2_PLACEMENT_3D ( 'NONE', #16157, #38556, #29379 ) ;
#38285=CARTESIAN_POINT ( 'NONE',  ( -58.35332038481796957, -0.2570561626924458554, 0.1612409511329637168 ) ) ;
#38291=ORIENTED_EDGE ( 'NONE', *, *, #20565, .T. ) ;
#38295=CARTESIAN_POINT ( 'NONE',  ( -28.96638701358144985, 63.08302880246334610, 1.523999999999992916 ) ) ;
#38297=EDGE_LOOP ( 'NONE', ( #33423, #32562, #31214, #13628 ) ) ;
#38299=CARTESIAN_POINT ( 'NONE',  ( -29.30242189345354831, 66.59148765006932535, 1.524000000000569344 ) ) ;
#38301=CARTESIAN_POINT ( 'NONE',  ( -17.14500000000466784, 71.11999999999886768, -1.524000000000000909 ) ) ;
#38302=CARTESIAN_POINT ( 'NONE',  ( -36.65473259702432784, 28.27472347546385123, -1.270000000000003570 ) ) ;
#38313=AXIS2_PLACEMENT_3D ( 'NONE', #38773, #29171, #229 ) ;
#38314=B_SPLINE_CURVE_WITH_KNOTS ( 'NONE', 3,
 ( #30772, #2458, #21583, #17984, #27582, #34611, #24168, #40590, #38013, #30981, #1821, #8835, #14785, #40797, #34825, #11597, #37586, #32672, #9258, #35451, #16044, #2875, #22631, #28630, #9870, #31830, #38232 ),
 .UNSPECIFIED., .F., .F.,
 ( 4, 1, 1, 1, 1, 1, 1, 1, 1, 1, 1, 1, 1, 1, 1, 1, 1, 1, 1, 1, 1, 1, 1, 1, 4 ),
 ( 0.000000000000000000, 0.02298233349012935092, 0.04596466698025847980, 0.05745583372532304944, 0.06894700047038783419, 0.08043816721545261894, 0.09192933396051740369, 0.1034205007055817582, 0.1149116674506463209, 0.1264028341957113277, 0.1378940009407758904, 0.1838586679210341412, 0.2298233349012926419, 0.2757880018815508927, 0.3217526688618093655, 0.3677173358420680049, 0.4136820028223265333, 0.4596466698025850617, 0.5056113367828434235, 0.5515760037631017854, 0.5975406707433603692, 0.6435053377236188421, 0.6664876712137480785, 0.6894700047038772039, 0.7354344192538664338 ),
 .UNSPECIFIED. ) ;
#38316=ORIENTED_EDGE ( 'NONE', *, *, #38000, .F. ) ;
#38317=CARTESIAN_POINT ( 'NONE',  ( -54.95604735203036029, 6.474113128985478305, 1.942216106931671904 ) ) ;
#38321=DIRECTION ( 'NONE',  ( 0.4849315768086535638, 0.8745520943968251304, 2.742148322653192551E-14 ) ) ;
#38326=VERTEX_POINT ( 'NONE', #5937 ) ;
#38330=CARTESIAN_POINT ( 'NONE',  ( -9.712308604790296229, 65.53852105402241079, -1.523999999999996025 ) ) ;
#38333=CIRCLE ( 'NONE', #14509, 0.2539999999999937863 ) ;
#38334=CARTESIAN_POINT ( 'NONE',  ( -46.85748110696954427, 25.55033861525921779, 1.599144941528299224 ) ) ;
#38335=CARTESIAN_POINT ( 'NONE',  ( -47.31580374228550312, 25.16323110364244897, 0.6294670755810632956 ) ) ;
#38337=CARTESIAN_POINT ( 'NONE',  ( -47.87216941255763203, 19.82042534259524658, 5.426529464407925829 ) ) ;
#38339=ADVANCED_FACE ( 'NONE', ( #18897 ), #31906, .F. ) ;
#38349=TOROIDAL_SURFACE ( 'NONE', #19967, 0.7620000000000000107, 0.2540000000000000036 ) ;
#38363=AXIS2_PLACEMENT_3D ( 'NONE', #19806, #3653, #16620 ) ;
#38369=ORIENTED_EDGE ( 'NONE', *, *, #27356, .T. ) ;
#38377=CIRCLE ( 'NONE', #34975, 0.2539999999999973390 ) ;
#38379=CARTESIAN_POINT ( 'NONE',  ( -41.05189575270516400, 23.09451173561988213, -0.7620000000000052287 ) ) ;
#38384=ORIENTED_EDGE ( 'NONE', *, *, #5633, .F. ) ;
#38388=EDGE_CURVE ( 'NONE', #120, #30637, #28240, .T. ) ;
#38395=AXIS2_PLACEMENT_3D ( 'NONE', #32187, #26417, #19799 ) ;
#38397=PLANE ( 'NONE',  #23037 ) ;
#38403=TOROIDAL_SURFACE ( 'NONE', #310, 0.3809999999999995057, 0.2540000000000000036 ) ;
#38414=ORIENTED_EDGE ( 'NONE', *, *, #10530, .T. ) ;
#38415=CARTESIAN_POINT ( 'NONE',  ( -42.66890350025449408, 21.80565315997039733, -1.797223148892109545 ) ) ;
#38420=CARTESIAN_POINT ( 'NONE',  ( -54.46595390896940359, 8.352818827531990564, -3.537195888581306402 ) ) ;
#38421=EDGE_CURVE ( 'NONE', #22644, #32069, #15303, .T. ) ;
#38429=CARTESIAN_POINT ( 'NONE',  ( -51.09990735641632398, 14.52648110433587370, -4.713018929684125169 ) ) ;
#38435=ADVANCED_FACE ( 'NONE', ( #2087 ), #41061, .F. ) ;
#38440=CARTESIAN_POINT ( 'NONE',  ( -46.81030548986588968, 25.80411194895121341, 1.573461678943545161 ) ) ;
#38443=CARTESIAN_POINT ( 'NONE',  ( -6.096037513970406607, 78.08166987308820239, 1.270000000000003126 ) ) ;
#38444=CARTESIAN_POINT ( 'NONE',  ( -48.50421218116022004, 14.67712143704007133, -0.4105607596418053284 ) ) ;
#38446=CARTESIAN_POINT ( 'NONE',  ( -57.80205714066466527, 2.371715784325115095, 1.753227392946289598 ) ) ;
#38447=CARTESIAN_POINT ( 'NONE',  ( -52.49023018389913631, 12.05517075480290679, 4.265271142760512113 ) ) ;
#38450=CARTESIAN_POINT ( 'NONE',  ( -57.66243511465493299, 3.255537196535568611, -1.046671340306231880E-14 ) ) ;
#38452=ORIENTED_EDGE ( 'NONE', *, *, #36077, .F. ) ;
#38453=CARTESIAN_POINT ( 'NONE',  ( -50.95401362087786623, 21.69085173448186055, -0.3723302588259480572 ) ) ;
#38461=DIRECTION ( 'NONE',  ( -5.188838149069471174E-16, 1.699382548006136313E-16, 1.000000000000000000 ) ) ;
#38468=ORIENTED_EDGE ( 'NONE', *, *, #5800, .F. ) ;
#38471=CARTESIAN_POINT ( 'NONE',  ( -4.377002418771855474, 72.24507371176854065, 1.270000000000004015 ) ) ;
#38480=EDGE_CURVE ( 'NONE', #35121, #40763, #3478, .T. ) ;
#38484=CARTESIAN_POINT ( 'NONE',  ( -43.83556092231052048, 21.45200552150719631, -2.811646013901254015 ) ) ;
#38488=DIRECTION ( 'NONE',  ( 0.9575201071113178530, -0.2883665106726683858, 8.537024980200786319E-16 ) ) ;
#38492=TOROIDAL_SURFACE ( 'NONE', #35093, 0.3809999999999990616, 0.2540000000000000036 ) ;
#38494=CARTESIAN_POINT ( 'NONE',  ( -23.91048590848665611, 81.84235438443283783, -1.524000000000006239 ) ) ;
#38501=DIRECTION ( 'NONE',  ( -5.188838149069471174E-16, 1.699382548006136313E-16, 1.000000000000000000 ) ) ;
#38503=FACE_OUTER_BOUND ( 'NONE', #9270, .T. ) ;
#38507=CARTESIAN_POINT ( 'NONE',  ( -29.35321562997442513, 61.36487289457124206, 1.523999999999994470 ) ) ;
#38510=DIRECTION ( 'NONE',  ( 0.000000000000000000, 0.000000000000000000, -1.000000000000000000 ) ) ;
#38514=DIRECTION ( 'NONE',  ( -5.188838149069472160E-16, 1.699382548006136559E-16, 1.000000000000000000 ) ) ;
#38524=DIRECTION ( 'NONE',  ( -0.8745520943968235761, 0.4849315768086558398, -5.691349986800547879E-16 ) ) ;
#38529=EDGE_LOOP ( 'NONE', ( #27102, #38110, #15300, #13770 ) ) ;
#38538=CARTESIAN_POINT ( 'NONE',  ( -46.85405389106658447, 25.56320314331479437, 1.590520987398670982 ) ) ;
#38539=CARTESIAN_POINT ( 'NONE',  ( -46.60530155212502734, 26.17382724835478314, 1.396999999999990472 ) ) ;
#38541=CARTESIAN_POINT ( 'NONE',  ( -47.65206802627297833, 20.46304711373551299, 5.210715034831059356 ) ) ;
#38548=DIRECTION ( 'NONE',  ( -5.188838149069472160E-16, 1.699382548006136559E-16, 1.000000000000000000 ) ) ;
#38552=LINE ( 'NONE', #6386, #9350 ) ;
#38556=DIRECTION ( 'NONE',  ( -0.6825627711659234542, -0.7308269722843399041, -2.299753143848148568E-16 ) ) ;
#38564=ORIENTED_EDGE ( 'NONE', *, *, #26871, .F. ) ;
#38569=CIRCLE ( 'NONE', #22207, 9.048749999999998295 ) ;
#38572=EDGE_CURVE ( 'NONE', #26682, #11267, #7849, .T. ) ;
#38573=EDGE_LOOP ( 'NONE', ( #4576, #25001, #40399, #40579, #41619, #3258, #1452, #5997, #147, #25287, #16619, #21629, #23416, #21419, #29713, #28470, #4524, #24838, #29699, #27514, #2386, #10152, #9886, #9445, #22855, #9564, #28872, #20630, #20891, #31893, #5579, #11884, #33850, #34740, #17285, #14290, #22028, #9774, #30002, #21799, #29774, #5211, #34810, #36517, #7759, #1959, #18408, #17922, #7410, #13376, #9184, #36020, #22360, #21774, #22203, #38884, #37463, #21443, #13295, #1287, #24295, #42081, #41332, #18425, #39239, #2637, #378, #22485, #39770, #5475, #18720, #8527, #11147, #17450, #7549, #19312 ) ) ;
#38574=FACE_OUTER_BOUND ( 'NONE', #1952, .T. ) ;
#38577=DIRECTION ( 'NONE',  ( 0.01731298258488003436, -0.9998501190848634312, 0.000000000000000000 ) ) ;
#38582=LINE ( 'NONE', #2812, #12534 ) ;
#38587=AXIS2_PLACEMENT_3D ( 'NONE', #28384, #2418, #18356 ) ;
#38588=EDGE_LOOP ( 'NONE', ( #34912, #2797, #35453, #15123 ) ) ;
#38589=CYLINDRICAL_SURFACE ( 'NONE', #21063, 0.5080000000000000071 ) ;
#38590=DIRECTION ( 'NONE',  ( 0.000000000000000000, 0.000000000000000000, -1.000000000000000000 ) ) ;
#38591=DIRECTION ( 'NONE',  ( 0.8745520943968235761, -0.4849315768086558398, 4.268512490100410909E-16 ) ) ;
#38602=EDGE_CURVE ( 'NONE', #4128, #29982, #25527, .T. ) ;
#38607=DIRECTION ( 'NONE',  ( -0.8745520943968241312, 0.4849315768086548406, -5.691349986800536046E-16 ) ) ;
#38611=DIRECTION ( 'NONE',  ( -0.6559537821943239866, 0.7548010569845283735, -4.686333752532408853E-16 ) ) ;
#38616=AXIS2_PLACEMENT_3D ( 'NONE', #19000, #22391, #16217 ) ;
#38617=VERTEX_POINT ( 'NONE', #5714 ) ;
#38621=DIRECTION ( 'NONE',  ( -0.8745520943968235761, 0.4849315768086558398, -5.691349986800547879E-16 ) ) ;
#38625=EDGE_CURVE ( 'NONE', #37552, #29590, #18033, .T. ) ;
#38627=CARTESIAN_POINT ( 'NONE',  ( -56.27576540577094732, 4.709657678713138118, -2.637635859394501292 ) ) ;
#38629=CARTESIAN_POINT ( 'NONE',  ( -58.34386316732116740, -0.2371896724559646730, -0.2005938501612954394 ) ) ;
#38636=CARTESIAN_POINT ( 'NONE',  ( -58.24807683554808335, 1.288543178753334573, -1.357556113208963744 ) ) ;
#38638=EDGE_LOOP ( 'NONE', ( #9729, #18785, #40614, #21136 ) ) ;
#38640=ORIENTED_EDGE ( 'NONE', *, *, #16727, .F. ) ;
#38652=CARTESIAN_POINT ( 'NONE',  ( -45.43219756685621036, 19.09711438432238495, -1.200471166368914933 ) ) ;
#38654=DIRECTION ( 'NONE',  ( -0.8745520943968250194, 0.4849315768086535083, -5.424246918827963022E-16 ) ) ;
#38655=CARTESIAN_POINT ( 'NONE',  ( -47.16890147375944764, 22.20336809214633433, 4.187060126831872786 ) ) ;
#38656=CARTESIAN_POINT ( 'NONE',  ( -53.84782375693468737, 9.539003880032991489, 3.783945623633715893 ) ) ;
#38660=CARTESIAN_POINT ( 'NONE',  ( -54.56940519185135230, 9.666406039105165604, 3.302709833357596381 ) ) ;
#38663=CARTESIAN_POINT ( 'NONE',  ( -52.46220839783629941, 13.84563717269405458, -4.010158452165651255 ) ) ;
#38665=EDGE_CURVE ( 'NONE', #7253, #2316, #34387, .T. ) ;
#38666=ORIENTED_EDGE ( 'NONE', *, *, #25378, .T. ) ;
#38678=LINE ( 'NONE', #6095, #518 ) ;
#38679=CARTESIAN_POINT ( 'NONE',  ( -17.14500000000466784, 71.11999999999886768, 1.523999999999998689 ) ) ;
#38683=CARTESIAN_POINT ( 'NONE',  ( -58.37116772670351850, -0.2940390518722524327, -2.603646672650065119E-13 ) ) ;
#38693=DIRECTION ( 'NONE',  ( 5.188838149069472160E-16, -1.699382548006136559E-16, -1.000000000000000000 ) ) ;
#38694=CARTESIAN_POINT ( 'NONE',  ( -47.00787117332040310, 24.49876931072293829, -2.333946431867834015 ) ) ;
#38695=ORIENTED_EDGE ( 'NONE', *, *, #19649, .T. ) ;
#38698=CIRCLE ( 'NONE', #24376, 0.2539999999999998925 ) ;
#38699=AXIS2_PLACEMENT_3D ( 'NONE', #6298, #3106, #16067 ) ;
#38700=CARTESIAN_POINT ( 'NONE',  ( -29.81357423954495189, 70.62209452652477637, -1.270000000000007123 ) ) ;
#38705=CARTESIAN_POINT ( 'NONE',  ( -17.14500000000466784, 71.11999999999886768, -1.524000000000000909 ) ) ;
#38706=DIRECTION ( 'NONE',  ( 0.8745520943968250194, -0.4849315768086534528, 5.361993529360573944E-16 ) ) ;
#38708=ORIENTED_EDGE ( 'NONE', *, *, #9148, .T. ) ;
#38712=DIRECTION ( 'NONE',  ( -5.188838149069471174E-16, 1.699382548006136313E-16, 1.000000000000000000 ) ) ;
#38722=AXIS2_PLACEMENT_3D ( 'NONE', #2889, #12669, #29859 ) ;
#38728=CLOSED_SHELL ( 'NONE', ( #10522, #29273, #33205, #39316, #40508, #3197, #28770, #30290, #35300, #155, #1111, #3711, #13923, #7743, #24211, #21571, #22765, #37582, #1384, #16236, #6164, #29529, #22980, #35491, #5600, #34915, #12882, #10048, #17226, #35705, #31052, #35399, #3818, #3979, #33520, #29759, #22415, #1515, #14696, #23441, #16298, #19331, #3500, #29829, #9244, #1971, #13409, #18393, #21609, #30919, #6063, #33165, #4018, #37175, #36300, #13397, #39476, #20568, #6020, #21756, #24711, #10232, #19120, #33192, #39435, #698, #11588, #11762, #25951, #14617, #27453, #19597, #14831, #16199, #42028, #32955, #12742, #15418, #36790, #41025, #33582, #24542, #21212, #9240, #31883, #28668, #11872, #25152, #38435, #35302, #22813, #29988, #3995, #17763, #38339, #7866, #16538, #11289, #17748, #20933, #3232, #7852, #35011, #39486, #17252, #111, #34978, #23784, #1622, #13359, #1602, #27370, #13985, #1705, #33402, #36067, #30923, #15173, #6356, #23798, #32405, #20948, #34019, #101, #36803, #15981, #8988, #30510, #29484, #3773, #20959, #41707, #41167, #3181, #1672, #35760, #9758, #23051, #25623, #37895, #19703, #13470, #26929, #29433, #4697, #22484, #39720, #23591, #12791, #15734, #24263, #18288, #9698, #41515, #28273, #30026, #32886, #31024, #2030, #32394, #11229, #17456, #23817, #35543, #32714, #21595, #40430, #11805, #4005, #12799, #1612, #16932, #22230, #14461, #30756, #7447, #22005, #7363, #26584, #37616, #23525, #5497, #8935, #8468, #618, #6945, #32651, #3334, #23450, #29187, #24270, #2121, #26391, #6122, #23463, #16828, #27739, #35836, #9048, #35247, #25325, #8646, #2664, #9044, #1407, #2028, #11510, #2171, #20275, #41805, #22463, #18601, #36843, #24353, #23249, #35818, #31382, #29330, #13135, #3730, #31152, #41734, #32228, #28577, #40713, #5809, #13354, #6628, #9658, #28938, #21894, #16758, #8143, #31742, #37306, #6947, #33699, #7106, #40188, #31244, #32656, #16521, #22240, #25391, #31695, #40553 ) ) ;
#38734=CARTESIAN_POINT ( 'NONE',  ( -29.94429436251954613, 71.80236127745905605, -1.524000000000007571 ) ) ;
#38737=VERTEX_POINT ( 'NONE', #37716 ) ;
#38739=DIRECTION ( 'NONE',  ( -0.6850534820564764260, 0.7284927773988544297, 1.146843430008119832E-15 ) ) ;
#38740=DIRECTION ( 'NONE',  ( -0.9876665170007968841, 0.1565721916417945614, -2.874959381037663881E-15 ) ) ;
#38746=CARTESIAN_POINT ( 'NONE',  ( -11.05715273818225164, 82.67346420587206524, -1.523999999999999577 ) ) ;
#38747=CARTESIAN_POINT ( 'NONE',  ( -48.09020259270877062, 19.08749025517105480, 5.202481609175432453 ) ) ;
#38750=CARTESIAN_POINT ( 'NONE',  ( -45.91718695868514288, 25.22619731686664224, 1.578102078770057037 ) ) ;
#38751=CARTESIAN_POINT ( 'NONE',  ( -58.81095673130623425, -0.2799022426899211990, 0.1165709727617455505 ) ) ;
#38753=CARTESIAN_POINT ( 'NONE',  ( -58.28497307353767809, -0.1385909279409680561, -1.048413496073990905E-14 ) ) ;
#38754=VERTEX_POINT ( 'NONE', #5358 ) ;
#38769=DIRECTION ( 'NONE',  ( -5.188838149069471174E-16, 1.699382548006136313E-16, 1.000000000000000000 ) ) ;
#38773=CARTESIAN_POINT ( 'NONE',  ( -24.32950799593924884, 77.42192949967211746, 1.523999999999993804 ) ) ;
#38778=ORIENTED_EDGE ( 'NONE', *, *, #25566, .F. ) ;
#38779=AXIS2_PLACEMENT_3D ( 'NONE', #17041, #674, #26635 ) ;
#38780=ORIENTED_EDGE ( 'NONE', *, *, #17244, .T. ) ;
#38792=ORIENTED_EDGE ( 'NONE', *, *, #26678, .F. ) ;
#38797=FACE_OUTER_BOUND ( 'NONE', #11075, .T. ) ;
#38801=CARTESIAN_POINT ( 'NONE',  ( -4.466782427718574588, 71.06098887363195615, -1.523999999999994248 ) ) ;
#38813=PLANE ( 'NONE',  #32129 ) ;
#38815=AXIS2_PLACEMENT_3D ( 'NONE', #7492, #33896, #20452 ) ;
#38816=EDGE_CURVE ( 'NONE', #1088, #11005, #19381, .T. ) ;
#38820=VERTEX_POINT ( 'NONE', #41347 ) ;
#38822=ORIENTED_EDGE ( 'NONE', *, *, #5838, .T. ) ;
#38826=CIRCLE ( 'NONE', #69, 0.2540000000000000591 ) ;
#38829=CARTESIAN_POINT ( 'NONE',  ( -58.17934017679519343, 0.6739543484516548055, -1.160953350562855091 ) ) ;
#38831=CARTESIAN_POINT ( 'NONE',  ( -58.26714162322899426, -0.07371858623886340389, -0.4245910480433032763 ) ) ;
#38835=DIRECTION ( 'NONE',  ( -0.8745520943968251304, 0.4849315768086532863, -5.424246918827961050E-16 ) ) ;
#38837=AXIS2_PLACEMENT_3D ( 'NONE', #252, #19392, #10025 ) ;
#38839=CARTESIAN_POINT ( 'NONE',  ( -58.20820809768403592, 1.420579653404085985, -1.355822160094614759 ) ) ;
#38850=CARTESIAN_POINT ( 'NONE',  ( -46.84426172109978381, 25.74287342672570844, 1.326046531035948828 ) ) ;
#38854=CARTESIAN_POINT ( 'NONE',  ( -30.20416046766209917, 71.17241488000101413, 1.269999999999991580 ) ) ;
#38855=CARTESIAN_POINT ( 'NONE',  ( -45.58494389689082738, 18.10922195552005221, -0.2974575429725926368 ) ) ;
#38859=CARTESIAN_POINT ( 'NONE',  ( -47.07934102874912696, 22.98505637820354153, 3.579966862081923828 ) ) ;
#38860=CARTESIAN_POINT ( 'NONE',  ( -52.68752125517421092, 11.69862226064154065, 4.201349328611278189 ) ) ;
#38863=LINE ( 'NONE', #9674, #12375 ) ;
#38864=CARTESIAN_POINT ( 'NONE',  ( -54.06930887699937216, 11.98206827348202808, 2.380698788532457311 ) ) ;
#38865=CARTESIAN_POINT ( 'NONE',  ( -56.78650302187183740, 3.241477563879227475, 2.205756828360251109 ) ) ;
#38868=CARTESIAN_POINT ( 'NONE',  ( -52.43464216547582879, 18.97776253636583732, -1.102323479587938957E-14 ) ) ;
#38870=ORIENTED_EDGE ( 'NONE', *, *, #37098, .T. ) ;
#38884=ORIENTED_EDGE ( 'NONE', *, *, #34679, .T. ) ;
#38887=CARTESIAN_POINT ( 'NONE',  ( -58.36310612058592540, -0.2775539044676491041, -0.1022538777131802717 ) ) ;
#38893=VECTOR ( 'NONE', #4363, 1000.000000000000000 ) ;
#38894=DIRECTION ( 'NONE',  ( 0.9876665170007968841, -0.1565721916417935344, 5.390917751951443929E-16 ) ) ;
#38897=VERTEX_POINT ( 'NONE', #39184 ) ;
#38902=CARTESIAN_POINT ( 'NONE',  ( -46.91604881613255174, 25.30076613767161220, -1.786867259277528985 ) ) ;
#38906=DIRECTION ( 'NONE',  ( 0.6594218222380214822, 0.7517731442105972661, 4.341145124518715900E-16 ) ) ;
#38908=EDGE_CURVE ( 'NONE', #5996, #18705, #3111, .T. ) ;
#38913=CARTESIAN_POINT ( 'NONE',  ( -58.36919919733277595, -0.2903088519664511757, 0.02951549999211592473 ) ) ;
#38914=AXIS2_PLACEMENT_3D ( 'NONE', #41177, #11981, #34784 ) ;
#38915=B_SPLINE_CURVE_WITH_KNOTS ( 'NONE', 3,
 ( #29761, #13779, #37200, #5051, #34015, #4634, #4843, #18211, #31431, #21608, #27400, #20992, #17798, #1645, #38039, #5257, #18007, #14598, #27604, #31212, #11412, #37613, #41030, #34636, #24608, #30593, #30794, #21195 ),
 .UNSPECIFIED., .F., .F.,
 ( 4, 2, 2, 2, 2, 2, 2, 2, 2, 2, 2, 2, 2, 4 ),
 ( -6.000000002036711361E-08, 0.0002743568420867710956, 0.0005487736841735625431, 0.001097607368347123212, 0.001646441052520683773, 0.002195274736694244333, 0.003292942105041382368, 0.004390609473388520402, 0.005488276841735658003, 0.006585944210082795604, 0.007134777894256365272, 0.007683611578429934072, 0.008232445262603502872, 0.008781278946777071673 ),
 .UNSPECIFIED. ) ;
#38919=ORIENTED_EDGE ( 'NONE', *, *, #7643, .T. ) ;
#38921=LINE ( 'NONE', #13138, #18975 ) ;
#38924=DIRECTION ( 'NONE',  ( -5.188838149069471174E-16, 1.699382548006136313E-16, 1.000000000000000000 ) ) ;
#38930=DIRECTION ( 'NONE',  ( -0.8745520943968236871, 0.4849315768086559508, -6.829619984160659032E-16 ) ) ;
#38944=FACE_OUTER_BOUND ( 'NONE', #37107, .T. ) ;
#38945=VECTOR ( 'NONE', #41829, 1000.000000000000000 ) ;
#38946=ORIENTED_EDGE ( 'NONE', *, *, #39889, .F. ) ;
#38949=CYLINDRICAL_SURFACE ( 'NONE', #13004, 0.6350000000000006750 ) ;
#38957=CARTESIAN_POINT ( 'NONE',  ( -46.91604881613258016, 25.30076613767155180, 1.786867259277509001 ) ) ;
#38959=CARTESIAN_POINT ( 'NONE',  ( -47.19936399096372526, 20.24790404726484283, 5.251082349106850344 ) ) ;
#38962=CARTESIAN_POINT ( 'NONE',  ( -58.37241122568488549, -0.2962816677227891882, -1.031899547879545818E-14 ) ) ;
#38973=CARTESIAN_POINT ( 'NONE',  ( -8.095114962461808616, 74.19100168833409725, 1.524000000000002686 ) ) ;
#38983=EDGE_LOOP ( 'NONE', ( #18255, #12068, #1444, #3126 ) ) ;
#38984=DIRECTION ( 'NONE',  ( 0.8745520943968235761, -0.4849315768086558398, 4.268512490100410909E-16 ) ) ;
#38989=TOROIDAL_SURFACE ( 'NONE', #20590, 0.7620000000000000107, 0.2540000000000000036 ) ;
#38992=ORIENTED_EDGE ( 'NONE', *, *, #23345, .F. ) ;
#38993=CARTESIAN_POINT ( 'NONE',  ( -41.38112080847943020, 22.74200708568027807, 0.4658591655018960442 ) ) ;
#39000=CARTESIAN_POINT ( 'NONE',  ( -6.650126595083637682, 78.47834120613788400, -1.269999999999996687 ) ) ;
#39004=EDGE_LOOP ( 'NONE', ( #19304, #22218, #13511, #40294 ) ) ;
#39005=DIRECTION ( 'NONE',  ( -5.188838149069471174E-16, 1.699382548006136313E-16, 1.000000000000000000 ) ) ;
#39007=CARTESIAN_POINT ( 'NONE',  ( -23.21760062652228029, 78.26400813401573942, -1.270000000000004903 ) ) ;
#39008=CARTESIAN_POINT ( 'NONE',  ( -58.78565887484231212, -0.2971860671465154091, 0.1726678976671059684 ) ) ;
#39009=AXIS2_PLACEMENT_3D ( 'NONE', #2289, #40837, #1450 ) ;
#39031=ORIENTED_EDGE ( 'NONE', *, *, #6916, .T. ) ;
#39035=CIRCLE ( 'NONE', #6370, 0.7620000000000000107 ) ;
#39040=CARTESIAN_POINT ( 'NONE',  ( -58.67480324322914953, -0.3139011383600042726, -0.3141419669791276625 ) ) ;
#39042=CARTESIAN_POINT ( 'NONE',  ( -4.394136353581303389, 70.68697878297604120, -1.523999999999994026 ) ) ;
#39044=CIRCLE ( 'NONE', #13183, 0.2539999999999978386 ) ;
#39049=CARTESIAN_POINT ( 'NONE',  ( -57.53497731650991653, 2.247686704661286505, -1.882970859819768306 ) ) ;
#39050=CIRCLE ( 'NONE', #2990, 0.7620000000000000107 ) ;
#39058=TOROIDAL_SURFACE ( 'NONE', #37023, 0.7620000000000000107, 0.2540000000000000036 ) ;
#39061=CARTESIAN_POINT ( 'NONE',  ( -50.84949806483948720, 11.71728973011883923, -8.857595425233459675E-15 ) ) ;
#39064=CARTESIAN_POINT ( 'NONE',  ( -8.584304875092012566, 68.18838345945393087, -1.523999999999995802 ) ) ;
#39068=LINE ( 'NONE', #19032, #7269 ) ;
#39069=CARTESIAN_POINT ( 'NONE',  ( -50.02669608763528686, 12.78473261814649931, -8.449425852006687485E-15 ) ) ;
#39072=CARTESIAN_POINT ( 'NONE',  ( -46.74873316577708238, 25.87611666761727847, -1.399911675830463054 ) ) ;
#39073=DIRECTION ( 'NONE',  ( -0.8745520943968243532, 0.4849315768086547296, -5.361993529360573944E-16 ) ) ;
#39074=DIRECTION ( 'NONE',  ( 0.9876665170007972172, -0.1565721916417913695, -6.288420277261245215E-16 ) ) ;
#39077=LINE ( 'NONE', #39286, #19827 ) ;
#39078=CARTESIAN_POINT ( 'NONE',  ( -57.36672490206960617, 3.909939030509804070, 0.6468086288197671951 ) ) ;
#39079=CARTESIAN_POINT ( 'NONE',  ( -58.11258158571958177, 1.603013069906233934, 1.501710181103012465 ) ) ;
#39081=ORIENTED_EDGE ( 'NONE', *, *, #15398, .T. ) ;
#39082=CARTESIAN_POINT ( 'NONE',  ( -49.81807968324856972, 18.07223176367294570, -4.612844822355063990 ) ) ;
#39084=ORIENTED_EDGE ( 'NONE', *, *, #14633, .F. ) ;
#39092=DIRECTION ( 'NONE',  ( -0.6878275643654763183, -0.7258741224889179167, -2.335488090154185488E-16 ) ) ;
#39095=CARTESIAN_POINT ( 'NONE',  ( -47.85244527695891037, 19.39403540832952544, -5.219971639306605127 ) ) ;
#39100=CARTESIAN_POINT ( 'NONE',  ( -58.34256328868874419, -0.2344693364347718856, -0.2069899249132446384 ) ) ;
#39110=ORIENTED_EDGE ( 'NONE', *, *, #26623, .F. ) ;
#39115=CARTESIAN_POINT ( 'NONE',  ( -46.30033180095409051, 21.65562830348028456, -4.292083522273610008 ) ) ;
#39125=CARTESIAN_POINT ( 'NONE',  ( -47.32981077577592544, 19.92739019301280834, -5.119713631627043959 ) ) ;
#39126=FACE_OUTER_BOUND ( 'NONE', #32979, .T. ) ;
#39129=ORIENTED_EDGE ( 'NONE', *, *, #14633, .T. ) ;
#39136=ORIENTED_EDGE ( 'NONE', *, *, #458, .T. ) ;
#39143=EDGE_CURVE ( 'NONE', #29332, #7253, #4454, .T. ) ;
#39155=CARTESIAN_POINT ( 'NONE',  ( -23.94760723868026631, 77.08694321397520355, 1.269999999999992912 ) ) ;
#39158=ORIENTED_EDGE ( 'NONE', *, *, #31687, .F. ) ;
#39164=CARTESIAN_POINT ( 'NONE',  ( -29.82321757229076908, 71.17901112636586447, -1.270000000000007123 ) ) ;
#39165=CARTESIAN_POINT ( 'NONE',  ( -49.98771841168287722, 16.20356568994197843, 4.825110013074525916 ) ) ;
#39166=CARTESIAN_POINT ( 'NONE',  ( -47.04217617083259029, 23.73857702128102076, 2.948847133965281309 ) ) ;
#39168=CARTESIAN_POINT ( 'NONE',  ( -54.39768377094780760, 8.094885465611476150, 3.421923752996821833 ) ) ;
#39169=CARTESIAN_POINT ( 'NONE',  ( -4.416771755448873904, 71.99420641645033925, -1.523999999999994248 ) ) ;
#39171=CARTESIAN_POINT ( 'NONE',  ( -5.809227842914839179, 77.60418761620948658, -1.269999999999996021 ) ) ;
#39179=CARTESIAN_POINT ( 'NONE',  ( -46.97515415817102280, 24.89137758704634962, -2.045406795549905787 ) ) ;
#39184=CARTESIAN_POINT ( 'NONE',  ( -24.23745918283205469, 82.38670122043342303, 1.269999999999992690 ) ) ;
#39191=EDGE_LOOP ( 'NONE', ( #29773, #5410, #20573, #31514 ) ) ;
#39197=EDGE_CURVE ( 'NONE', #7000, #26382, #853, .T. ) ;
#39199=ORIENTED_EDGE ( 'NONE', *, *, #34248, .T. ) ;
#39201=CARTESIAN_POINT ( 'NONE',  ( -44.40685758373556524, 19.43703734468909516, -5.999789834925398652E-15 ) ) ;
#39213=ORIENTED_EDGE ( 'NONE', *, *, #15618, .F. ) ;
#39216=LINE ( 'NONE', #22783, #7551 ) ;
#39217=VECTOR ( 'NONE', #12311, 1000.000000000000000 ) ;
#39219=VECTOR ( 'NONE', #26903, 1000.000000000000000 ) ;
#39233=LINE ( 'NONE', #26656, #16411 ) ;
#39239=ORIENTED_EDGE ( 'NONE', *, *, #13127, .T. ) ;
#39242=CIRCLE ( 'NONE', #40621, 0.2540000000000002256 ) ;
#39243=VERTEX_POINT ( 'NONE', #17227 ) ;
#39249=EDGE_CURVE ( 'NONE', #39372, #13050, #30297, .T. ) ;
#39251=CARTESIAN_POINT ( 'NONE',  ( -58.51800049984071705, -0.05885670287285882374, -0.6510176481063610909 ) ) ;
#39254=AXIS2_PLACEMENT_3D ( 'NONE', #15843, #28637, #41863 ) ;
#39257=CARTESIAN_POINT ( 'NONE',  ( -44.11964021406032543, 21.57970624656428171, 2.906001918892821223 ) ) ;
#39258=EDGE_CURVE ( 'NONE', #31300, #19961, #7212, .T. ) ;
#39261=CARTESIAN_POINT ( 'NONE',  ( -57.43854689232674815, 1.757847328446624058, -1.624773336220253217 ) ) ;
#39262=ORIENTED_EDGE ( 'NONE', *, *, #9466, .F. ) ;
#39265=ORIENTED_EDGE ( 'NONE', *, *, #38191, .F. ) ;
#39269=VECTOR ( 'NONE', #23777, 1000.000000000000227 ) ;
#39278=CARTESIAN_POINT ( 'NONE',  ( -45.15528325240632057, 20.88806775524793125, -3.529375091719475943 ) ) ;
#39281=FACE_OUTER_BOUND ( 'NONE', #4759, .T. ) ;
#39286=CARTESIAN_POINT ( 'NONE',  ( -27.59695233663404679, 58.25262445104075226, 1.523999999999995358 ) ) ;
#39287=CARTESIAN_POINT ( 'NONE',  ( -55.34794038087419210, 7.786537553440359360, 3.264576684945853291 ) ) ;
#39288=CARTESIAN_POINT ( 'NONE',  ( -58.03414100541874632, 0.4564111095344686175, 0.9708715263941495310 ) ) ;
#39290=ORIENTED_EDGE ( 'NONE', *, *, #41569, .T. ) ;
#39291=CARTESIAN_POINT ( 'NONE',  ( -51.34394198884087501, 20.23131347170496142, -0.7795225783603546565 ) ) ;
#39293=EDGE_LOOP ( 'NONE', ( #42096, #13099, #10640, #23722 ) ) ;
#39306=DIRECTION ( 'NONE',  ( -5.188838149069472160E-16, 1.699382548006136559E-16, 1.000000000000000000 ) ) ;
#39311=CARTESIAN_POINT ( 'NONE',  ( -58.36826665097051148, -0.2883791471137164830, -0.04671551776550799534 ) ) ;
#39316=ADVANCED_FACE ( 'NONE', ( #21040 ), #38492, .T. ) ;
#39325=CARTESIAN_POINT ( 'NONE',  ( -44.66298991629287940, 23.47648082339880915, -1.964675176939946644 ) ) ;
#39334=EDGE_CURVE ( 'NONE', #2940, #8461, #35753, .T. ) ;
#39337=AXIS2_PLACEMENT_3D ( 'NONE', #25732, #12541, #25938 ) ;
#39351=DIRECTION ( 'NONE',  ( -5.188838149069472160E-16, 1.699382548006136559E-16, 1.000000000000000000 ) ) ;
#39363=EDGE_CURVE ( 'NONE', #18759, #34369, #21461, .T. ) ;
#39370=CARTESIAN_POINT ( 'NONE',  ( -29.82321757229076908, 71.17901112636586447, -1.524000000000007349 ) ) ;
#39372=VERTEX_POINT ( 'NONE', #30846 ) ;
#39374=CARTESIAN_POINT ( 'NONE',  ( -30.45812239790965492, 71.16801738242446618, -1.524000000000007793 ) ) ;
#39375=CARTESIAN_POINT ( 'NONE',  ( -10.15441061790785682, 81.86333342972157823, -1.269999999999998908 ) ) ;
#39378=EDGE_CURVE ( 'NONE', #37219, #16254, #16708, .T. ) ;
#39381=CARTESIAN_POINT ( 'NONE',  ( -48.95619900250866863, 17.85589990993532439, 5.076226165768623844 ) ) ;
#39382=CARTESIAN_POINT ( 'NONE',  ( -47.35944255389389923, 21.37623662739411401, 4.722871667523157235 ) ) ;
#39383=CARTESIAN_POINT ( 'NONE',  ( -41.28107547821694112, 23.22158991241130011, 1.523999999999988475 ) ) ;
#39384=EDGE_CURVE ( 'NONE', #37691, #8502, #41908, .T. ) ;
#39385=CARTESIAN_POINT ( 'NONE',  ( -50.11792632901008915, 17.09067799859288783, 5.048577231237564966 ) ) ;
#39386=CARTESIAN_POINT ( 'NONE',  ( -11.53797084252497562, 82.58007221317646440, 1.269999999999999130 ) ) ;
#39389=VERTEX_POINT ( 'NONE', #24239 ) ;
#39390=DIRECTION ( 'NONE',  ( -0.8572391118119510045, -0.5149185422762100339, -3.573031421855330583E-16 ) ) ;
#39391=CIRCLE ( 'NONE', #19657, 0.2539999999999997260 ) ;
#39400=DIRECTION ( 'NONE',  ( -5.188838149069472160E-16, 1.699382548006136559E-16, 1.000000000000000000 ) ) ;
#39401=DIRECTION ( 'NONE',  ( -0.8745520943968080330, 0.4849315768086841505, -5.271987356194194978E-16 ) ) ;
#39406=CYLINDRICAL_SURFACE ( 'NONE', #8384, 0.5080000000000000071 ) ;
#39412=VERTEX_POINT ( 'NONE', #37449 ) ;
#39413=EDGE_CURVE ( 'NONE', #26517, #14331, #22130, .T. ) ;
#39415=CARTESIAN_POINT ( 'NONE',  ( -47.11704014324648426, 20.18577099567724886, 5.127035723291425207 ) ) ;
#39425=EDGE_CURVE ( 'NONE', #11324, #5052, #28956, .T. ) ;
#39429=AXIS2_PLACEMENT_3D ( 'NONE', #21921, #40914, #14697 ) ;
#39431=DIRECTION ( 'NONE',  ( -5.188838149069472160E-16, 1.699382548006136559E-16, 1.000000000000000000 ) ) ;
#39435=ADVANCED_FACE ( 'NONE', ( #15068 ), #41079, .T. ) ;
#39453=CIRCLE ( 'NONE', #19025, 0.6350000000000030065 ) ;
#39457=AXIS2_PLACEMENT_3D ( 'NONE', #15021, #37406, #41458 ) ;
#39464=CARTESIAN_POINT ( 'NONE',  ( -58.82792982499385914, -0.2609477946144658778, -0.04398265886348604742 ) ) ;
#39465=ORIENTED_EDGE ( 'NONE', *, *, #11387, .T. ) ;
#39468=DIRECTION ( 'NONE',  ( 1.000000000000000000, 0.000000000000000000, 0.000000000000000000 ) ) ;
#39473=CARTESIAN_POINT ( 'NONE',  ( -57.92346726745822849, 0.7446056814934959300, -1.206286704679871535 ) ) ;
#39476=ADVANCED_FACE ( 'NONE', ( #11454 ), #24876, .T. ) ;
#39481=CARTESIAN_POINT ( 'NONE',  ( -29.81357423954495189, 70.62209452652477637, -1.270000000000007123 ) ) ;
#39482=CARTESIAN_POINT ( 'NONE',  ( -57.74058121727584592, 1.065718057877890201, 1.162857118034767545 ) ) ;
#39486=ADVANCED_FACE ( 'NONE', ( #34475 ), #4487, .T. ) ;
#39489=CARTESIAN_POINT ( 'NONE',  ( -5.924740142096584172, 65.21691166894066782, 1.524000000000005350 ) ) ;
#39490=( BOUNDED_SURFACE ( )  B_SPLINE_SURFACE ( 2, 3, ( 
 ( #604, #22923, #35954, #19734, #16550, #22714, #9331, #22294, #2949, #41928, #12729, #1439, #1651, #1236, #36386, #23348, #20999, #7615, #39792, #4013, #33603, #30802, #16970, #14193, #4849, #26781, #14399, #13785, #14606, #27198, #7202, #7826, #17805, #36586, #20577, #40211, #40417, #40003, #37007, #33185, #4436, #30601, #27407, #10586, #34024, #17183, #30182, #20788, #23564, #37207 ),
 ( #17394, #30385, #11009, #23988, #33812, #7404, #26992, #4640, #17597, #11213, #24197, #10794, #29969, #8028, #39573, #10379, #20160, #20366, #809, #33388, #4222, #1023, #13988, #23776, #36797, #32232, #5264, #40828, #22401, #6252, #3267, #18217, #41836, #32014, #28026, #22193, #11627, #28822, #37411, #24614, #22609, #8230, #37622, #41036, #25618, #32435, #12835, #9432, #1853, #11845 ),
 ( #8445, #31218, #24832, #3063, #35641, #24405, #21403, #19429, #18014, #9642, #34431, #42039, #2062, #21203, #35425, #2853, #19221, #29020, #15814, #34229, #15026, #37827, #14817, #5058, #19010, #25823, #16020, #27611, #38831, #27819, #9234, #31011, #6456, #40620, #12631, #38629, #35223, #6048, #11419, #7096, #32646, #17077, #13474, #33498, #20260, #20471, #20057, #13043, #75, #39891 ) ),
 .UNSPECIFIED., .F., .F., .T. ) 
 B_SPLINE_SURFACE_WITH_KNOTS ( ( 3, 3 ),
 ( 4, 2, 2, 2, 2, 2, 2, 2, 2, 2, 2, 2, 2, 2, 2, 2, 2, 2, 2, 2, 2, 2, 2, 2, 4 ),
 ( 0.000000000000000000, 1.000000000000000000 ),
 ( 0.000000000000000000, 0.001458241944942356878, 0.002916483889884713757, 0.005832967779769427513, 0.01166593555953885503, 0.01458241944942356878, 0.01749890333930828254, 0.01895714528425063855, 0.02041538722919299803, 0.02114450820166417777, 0.02150906868789976417, 0.02187362917413535404, 0.02223818966037094391, 0.02260275014660653031, 0.02296731063284212018, 0.02305845075440101505, 0.02310402081518046422, 0.02312680584557019053, 0.02313250210316761951, 0.02313819836076505196, 0.02314959087595991338, 0.02319516093673936255, 0.02324073099751881172, 0.02328630105829826089, 0.02333187111907771005 ),
 .UNSPECIFIED. ) 
 GEOMETRIC_REPRESENTATION_ITEM ( )  RATIONAL_B_SPLINE_SURFACE ( (
 ( 1.000000000000000000, 1.000000000000000000, 1.000000000000000000, 1.000000000000000000, 1.000000000000000000, 1.000000000000000000, 1.000000000000000000, 1.000000000000000000, 1.000000000000000000, 1.000000000000000000, 1.000000000000000000, 1.000000000000000000, 1.000000000000000000, 1.000000000000000000, 1.000000000000000000, 1.000000000000000000, 1.000000000000000000, 1.000000000000000000, 1.000000000000000000, 1.000000000000000000, 1.000000000000000000, 1.000000000000000000, 1.000000000000000000, 1.000000000000000000, 1.000000000000000000, 1.000000000000000000, 1.000000000000000000, 1.000000000000000000, 1.000000000000000000, 1.000000000000000000, 1.000000000000000000, 1.000000000000000000, 1.000000000000000000, 1.000000000000000000, 1.000000000000000000, 1.000000000000000000, 1.000000000000000000, 1.000000000000000000, 1.000000000000000000, 1.000000000000000000, 1.000000000000000000, 1.000000000000000000, 1.000000000000000000, 1.000000000000000000, 1.000000000000000000, 1.000000000000000000, 1.000000000000000000, 1.000000000000000000, 1.000000000000000000, 1.000000000000000000),
 ( 0.9987193938133603899, 0.9996013059082062835, 0.9991963860897459249, 0.9949866313572486298, 0.9909603791786357752, 0.9774858857060727546, 0.9654485462826584152, 0.9208787474394699579, 0.8807605768841590965, 0.8373543814140436137, 0.8249666374273941782, 0.8044008243570911487, 0.7962249832256278470, 0.7861950991343641393, 0.7832680976383418203, 0.7777782220923173950, 0.7752303374625654220, 0.7716286403948026118, 0.7703172242824322113, 0.7685261186013288004, 0.7673635575507736784, 0.7657163664511276169, 0.7656514573019265191, 0.7645255059884744631, 0.7630494482559035951, 0.7607147317261879760, 0.7600215756462245231, 0.7585094466923363310, 0.7575231611311871172, 0.7546848085732021927, 0.7541407386738737673, 0.7516848864309048084, 0.7509064819815688407, 0.7462986158550390936, 0.7479156148844432472, 0.7339777749606422041, 0.7233604987231169181, 0.7138238211886495099, 0.7102391262350743473, 0.6994720207877663798, 0.6929862625726375125, 0.6601362149651482936, 0.6323867238882598940, 0.5714353380975951691, 0.5388352690754523167, 0.4817946329372650993, 0.4578268140826607380, 0.4260966422721294555, 0.4180307774944384547, 0.4190531958288030157),
 ( 1.000000000000000000, 1.000000000000000000, 1.000000000000000000, 1.000000000000000000, 1.000000000000000000, 1.000000000000000000, 1.000000000000000000, 1.000000000000000000, 1.000000000000000000, 1.000000000000000000, 1.000000000000000000, 1.000000000000000000, 1.000000000000000000, 1.000000000000000000, 1.000000000000000000, 1.000000000000000000, 1.000000000000000000, 1.000000000000000000, 1.000000000000000000, 1.000000000000000000, 1.000000000000000000, 1.000000000000000000, 1.000000000000000000, 1.000000000000000000, 1.000000000000000000, 1.000000000000000000, 1.000000000000000000, 1.000000000000000000, 1.000000000000000000, 1.000000000000000000, 1.000000000000000000, 1.000000000000000000, 1.000000000000000000, 1.000000000000000000, 1.000000000000000000, 1.000000000000000000, 1.000000000000000000, 1.000000000000000000, 1.000000000000000000, 1.000000000000000000, 1.000000000000000000, 1.000000000000000000, 1.000000000000000000, 1.000000000000000000, 1.000000000000000000, 1.000000000000000000, 1.000000000000000000, 1.000000000000000000, 1.000000000000000000, 1.000000000000000000) ) ) 
 REPRESENTATION_ITEM ( '' )  SURFACE ( )  );
#39491=CARTESIAN_POINT ( 'NONE',  ( -54.16862281694330505, 7.200593192618495841, -0.5614961770967549226 ) ) ;
#39496=CARTESIAN_POINT ( 'NONE',  ( -29.27789202447384653, 65.71096991539397436, -1.523999999999142707 ) ) ;
#39497=VECTOR ( 'NONE', #36275, 1000.000000000000000 ) ;
#39500=DIRECTION ( 'NONE',  ( -0.9734199927291280474, -0.2290273297124694185, -8.537024980200812943E-16 ) ) ;
#39501=CARTESIAN_POINT ( 'NONE',  ( -58.55612285180487930, 0.6590214021355705887, 0.05016670522517701486 ) ) ;
#39502=CARTESIAN_POINT ( 'NONE',  ( -56.26318288983030413, 4.268071985104968213, 2.480832006587838645 ) ) ;
#39505=CARTESIAN_POINT ( 'NONE',  ( -57.89852354142710311, 2.261894840748110536, -1.235920526244146167 ) ) ;
#39509=CIRCLE ( 'NONE', #18380, 8.794749999999996959 ) ;
#39515=CARTESIAN_POINT ( 'NONE',  ( -17.31000046771894318, 62.32679794340116786, 1.524000000000000021 ) ) ;
#39522=ORIENTED_EDGE ( 'NONE', *, *, #19811, .T. ) ;
#39526=CARTESIAN_POINT ( 'NONE',  ( -57.60749290269577472, 1.353032280971704804, -1.296780305043655490 ) ) ;
#39540=AXIS2_PLACEMENT_3D ( 'NONE', #38262, #18215, #9079 ) ;
#39542=CARTESIAN_POINT ( 'NONE',  ( -56.82628769568140115, 4.502340570254503405, -2.499646007873257414 ) ) ;
#39543=CARTESIAN_POINT ( 'NONE',  ( -18.83202234259777086, 80.34319284215894186, 1.269999999999995799 ) ) ;
#39553=VERTEX_POINT ( 'NONE', #34897 ) ;
#39554=CARTESIAN_POINT ( 'NONE',  ( -5.591489108514605455, 77.73497692594764885, 1.270000000000003126 ) ) ;
#39558=DIRECTION ( 'NONE',  ( -5.188838149069471174E-16, 1.699382548006136313E-16, 1.000000000000000000 ) ) ;
#39562=CARTESIAN_POINT ( 'NONE',  ( -30.44847906516384128, 70.61110078258337808, 1.269999999999991580 ) ) ;
#39567=DIRECTION ( 'NONE',  ( -0.8745520943968245753, 0.4849315768086539524, -5.691349986800526185E-16 ) ) ;
#39569=CARTESIAN_POINT ( 'NONE',  ( -17.14500000000466784, 71.11999999999886768, -1.524000000000000909 ) ) ;
#39573=CARTESIAN_POINT ( 'NONE',  ( -56.62423581747610513, 3.520748359631705515, -2.300294558596477135 ) ) ;
#39574=DIRECTION ( 'NONE',  ( -0.8745520943968663197, 0.4849315768085789013, -5.691349986800499561E-16 ) ) ;
#39582=AXIS2_PLACEMENT_3D ( 'NONE', #23436, #901, #17061 ) ;
#39583=CARTESIAN_POINT ( 'NONE',  ( -43.35906100199910185, 21.49635880980142133, 2.252931129856620363 ) ) ;
#39590=AXIS2_PLACEMENT_3D ( 'NONE', #9879, #29482, #7130 ) ;
#39593=EDGE_CURVE ( 'NONE', #36869, #13695, #29247, .T. ) ;
#39596=DIRECTION ( 'NONE',  ( -5.188838149069472160E-16, 1.699382548006136559E-16, 1.000000000000000000 ) ) ;
#39597=CARTESIAN_POINT ( 'NONE',  ( -46.75240110268729410, 25.86707425373576541, 1.404788063146650501 ) ) ;
#39598=CARTESIAN_POINT ( 'NONE',  ( -48.35963184368405621, 21.82761434182101112, 2.838462189984248596 ) ) ;
#39600=CARTESIAN_POINT ( 'NONE',  ( -51.58367816905025194, 14.91232437457545146, 4.609044670965822377 ) ) ;
#39601=CARTESIAN_POINT ( 'NONE',  ( -58.59183231654615298, -0.2159720215225674478, 0.4817266061078952499 ) ) ;
#39605=CARTESIAN_POINT ( 'NONE',  ( -45.14658554404967106, 22.88857079803865346, 2.562886992506556272 ) ) ;
#39620=CARTESIAN_POINT ( 'NONE',  ( -23.62918761621517305, 82.45577215708875940, -1.524000000000006017 ) ) ;
#39629=CARTESIAN_POINT ( 'NONE',  ( -47.61549956331939626, 19.66157307908737195, 5.197827534590555132 ) ) ;
#39644=EDGE_CURVE ( 'NONE', #15945, #20056, #15334, .T. ) ;
#39645=CARTESIAN_POINT ( 'NONE',  ( -10.55305098051677426, 77.31887769575739355, 1.269999999999999796 ) ) ;
#39652=EDGE_CURVE ( 'NONE', #13978, #26949, #25712, .T. ) ;
#39659=CARTESIAN_POINT ( 'NONE',  ( -17.14500000000466784, 71.11999999999886768, -1.524000000000000909 ) ) ;
#39661=AXIS2_PLACEMENT_3D ( 'NONE', #17413, #1258, #27014 ) ;
#39664=FACE_OUTER_BOUND ( 'NONE', #20377, .T. ) ;
#39668=VECTOR ( 'NONE', #14419, 1000.000000000000114 ) ;
#39670=ORIENTED_EDGE ( 'NONE', *, *, #41253, .F. ) ;
#39671=CARTESIAN_POINT ( 'NONE',  ( -3.841520934845505941, 71.62889921741444255, -1.269999999999994023 ) ) ;
#39672=ORIENTED_EDGE ( 'NONE', *, *, #11339, .F. ) ;
#39679=CARTESIAN_POINT ( 'NONE',  ( -58.52263300247899735, -0.06897136332623234056, -0.6413478136646119099 ) ) ;
#39689=CARTESIAN_POINT ( 'NONE',  ( -29.50431010628811990, 60.44740661353770150, -1.524000000000005350 ) ) ;
#39692=ORIENTED_EDGE ( 'NONE', *, *, #20710, .T. ) ;
#39697=DIRECTION ( 'NONE',  ( 5.188838149069472160E-16, -1.699382548006136559E-16, -1.000000000000000000 ) ) ;
#39699=CARTESIAN_POINT ( 'NONE',  ( -48.15927431541864223, 19.02058896282273182, 5.220430799429900404 ) ) ;
#39706=CARTESIAN_POINT ( 'NONE',  ( -50.84949806483948720, 11.71728973011883923, -8.857595425233459675E-15 ) ) ;
#39708=DIRECTION ( 'NONE',  ( -0.8745520943968241312, 0.4849315768086548406, -5.691349986800536046E-16 ) ) ;
#39709=AXIS2_PLACEMENT_3D ( 'NONE', #3103, #16064, #9687 ) ;
#39710=CARTESIAN_POINT ( 'NONE',  ( -46.91299662966074635, 25.29696379526928496, -1.775053009676189397 ) ) ;
#39711=CARTESIAN_POINT ( 'NONE',  ( -48.41349243880052455, 18.68090591540773460, 5.201624795074226704 ) ) ;
#39712=CARTESIAN_POINT ( 'NONE',  ( -29.12312633939021822, 66.61190372955286421, -1.524000000000005350 ) ) ;
#39715=CARTESIAN_POINT ( 'NONE',  ( -21.91949108387693812, 59.24500507708427932, 1.523999999999998245 ) ) ;
#39716=CARTESIAN_POINT ( 'NONE',  ( -57.92473815682701144, 2.127617342915319565, 1.480748064241587114 ) ) ;
#39717=CARTESIAN_POINT ( 'NONE',  ( -58.09657527255103560, 0.9821181129459344294, 1.359330230256424521 ) ) ;
#39719=VECTOR ( 'NONE', #27831, 1000.000000000000114 ) ;
#39720=ADVANCED_FACE ( 'NONE', ( #9739 ), #22082, .T. ) ;
#39722=CARTESIAN_POINT ( 'NONE',  ( -57.36672490206960617, 3.909939030509804070, -0.6468086288197882894 ) ) ;
#39724=ORIENTED_EDGE ( 'NONE', *, *, #20565, .F. ) ;
#39725=FACE_OUTER_BOUND ( 'NONE', #11087, .T. ) ;
#39730=CIRCLE ( 'NONE', #22020, 0.2540000000000027236 ) ;
#39736=DIRECTION ( 'NONE',  ( 5.188838149069472160E-16, -1.699382548006136559E-16, -1.000000000000000000 ) ) ;
#39737=FACE_OUTER_BOUND ( 'NONE', #39191, .T. ) ;
#39738=ORIENTED_EDGE ( 'NONE', *, *, #8763, .F. ) ;
#39741=CARTESIAN_POINT ( 'NONE',  ( -58.21675469219344734, 0.03542984183141312249, -0.5229180514795568335 ) ) ;
#39748=CARTESIAN_POINT ( 'NONE',  ( -46.67659519887700981, 22.71018310752411651, -3.598098858967615055 ) ) ;
#39757=AXIS2_PLACEMENT_3D ( 'NONE', #6718, #6504, #553 ) ;
#39760=CARTESIAN_POINT ( 'NONE',  ( -52.76912830878634253, 12.08540908813377612, -4.334427935445254398 ) ) ;
#39765=CIRCLE ( 'NONE', #5070, 0.6349999999999977884 ) ;
#39770=ORIENTED_EDGE ( 'NONE', *, *, #12821, .T. ) ;
#39773=VERTEX_POINT ( 'NONE', #4430 ) ;
#39792=CARTESIAN_POINT ( 'NONE',  ( -57.79860935920169851, 1.496589803104450667, -1.561213607913327639 ) ) ;
#39793=DIRECTION ( 'NONE',  ( -5.188838149069472160E-16, 1.699382548006136559E-16, 1.000000000000000000 ) ) ;
#39802=DIRECTION ( 'NONE',  ( -0.4849315768086535083, -0.8745520943968250194, -1.030032898892974695E-16 ) ) ;
#39807=CARTESIAN_POINT ( 'NONE',  ( -30.84268108620762305, 55.46651512039750997, -1.270000000000005125 ) ) ;
#39811=DIRECTION ( 'NONE',  ( 5.188838149069472160E-16, -1.699382548006136559E-16, -1.000000000000000000 ) ) ;
#39813=DIRECTION ( 'NONE',  ( -0.8745520943968243532, 0.4849315768086547296, -6.829619984160642269E-16 ) ) ;
#39814=CARTESIAN_POINT ( 'NONE',  ( -57.34225532943530368, 1.923124478597425524, 1.535638195068367073 ) ) ;
#39815=CARTESIAN_POINT ( 'NONE',  ( -47.93352606754567091, 24.19884373620804396, 0.9125764105762101952 ) ) ;
#39817=CARTESIAN_POINT ( 'NONE',  ( -52.50198181065980663, 11.96455506022023307, 4.263607785004571937 ) ) ;
#39818=CARTESIAN_POINT ( 'NONE',  ( -58.51012109478204337, -0.04195086158869835297, 0.6673390170621641415 ) ) ;
#39822=CARTESIAN_POINT ( 'NONE',  ( -46.67659519887701691, 22.71018310752411651, 3.598098858967599512 ) ) ;
#39832=CARTESIAN_POINT ( 'NONE',  ( -43.11180532273385779, 21.58876176642518629, 2.074236749937639068 ) ) ;
#39835=DIRECTION ( 'NONE',  ( 0.4849315768086534528, 0.8745520943968250194, 1.030032898892974942E-16 ) ) ;
#39843=ORIENTED_EDGE ( 'NONE', *, *, #18498, .F. ) ;
#39845=CARTESIAN_POINT ( 'NONE',  ( -42.12253153191132782, 21.94389511927449732, 0.09363185731630196962 ) ) ;
#39876=CARTESIAN_POINT ( 'NONE',  ( -17.14500000000466784, 71.11999999999886768, 1.523999999999998689 ) ) ;
#39881=EDGE_CURVE ( 'NONE', #40718, #13050, #7882, .T. ) ;
#39883=DIRECTION ( 'NONE',  ( -0.4849315768086534528, -0.8745520943968249084, -1.030032898892974818E-16 ) ) ;
#39889=EDGE_CURVE ( 'NONE', #17866, #23676, #33050, .T. ) ;
#39891=CARTESIAN_POINT ( 'NONE',  ( -58.36992421181234647, -0.2917964073288620286, 4.861495987418534161E-13 ) ) ;
#39898=CARTESIAN_POINT ( 'NONE',  ( -24.10666987309389597, 82.16896248603319464, 1.523999999999993138 ) ) ;
#39899=ORIENTED_EDGE ( 'NONE', *, *, #34392, .T. ) ;
#39902=EDGE_CURVE ( 'NONE', #29093, #25690, #31673, .T. ) ;
#39904=VECTOR ( 'NONE', #35172, 999.9999999999998863 ) ;
#39909=CARTESIAN_POINT ( 'NONE',  ( -58.36582417652992660, -0.2832568706214733112, 0.07935633695520924458 ) ) ;
#39918=CARTESIAN_POINT ( 'NONE',  ( -52.48304539424793091, 11.63526101311008354, -3.802211793135442885 ) ) ;
#39921=FACE_OUTER_BOUND ( 'NONE', #26558, .T. ) ;
#39923=LINE ( 'NONE', #7127, #33153 ) ;
#39928=CARTESIAN_POINT ( 'NONE',  ( -58.43523997267251247, 0.9435442997105664142, 0.5849561510202019310 ) ) ;
#39931=AXIS2_PLACEMENT_3D ( 'NONE', #22901, #35937, #32954 ) ;
#39932=EDGE_LOOP ( 'NONE', ( #32005, #32149, #5789, #21306 ) ) ;
#39933=CARTESIAN_POINT ( 'NONE',  ( -56.91937565786325592, 5.591339438888994984, -0.1632292574589517820 ) ) ;
#39936=DIRECTION ( 'NONE',  ( 0.8745520943968249084, -0.4849315768086533418, 5.271987356194193006E-16 ) ) ;
#39950=CARTESIAN_POINT ( 'NONE',  ( -57.92987961479896342, 0.6565893080917146740, -0.9491229006729858808 ) ) ;
#39955=VECTOR ( 'NONE', #8345, 1000.000000000000000 ) ;
#39956=CARTESIAN_POINT ( 'NONE',  ( -41.45218294293373162, 22.69057396248467384, -1.547390787314429472 ) ) ;
#39965=DIRECTION ( 'NONE',  ( -0.8745520943968235761, 0.4849315768086558953, -5.361993529360570985E-16 ) ) ;
#39967=CARTESIAN_POINT ( 'NONE',  ( -50.15972161391664486, 17.13814111569220699, -4.955022299345085202 ) ) ;
#39968=EDGE_CURVE ( 'NONE', #12580, #8945, #8568, .T. ) ;
#39969=AXIS2_PLACEMENT_3D ( 'NONE', #16207, #9006, #35003 ) ;
#39983=CARTESIAN_POINT ( 'NONE',  ( -46.60530155212508419, 26.17382724835469432, -1.171222222222230824 ) ) ;
#39985=DIRECTION ( 'NONE',  ( -0.5149185422762221354, 0.8572391118119438991, -4.128606161907600514E-16 ) ) ;
#39993=ORIENTED_EDGE ( 'NONE', *, *, #20134, .T. ) ;
#39997=CARTESIAN_POINT ( 'NONE',  ( -24.10666987309389597, 82.16896248603319464, 1.269999999999993134 ) ) ;
#39998=AXIS2_PLACEMENT_3D ( 'NONE', #17284, #33491, #10474 ) ;
#40003=CARTESIAN_POINT ( 'NONE',  ( -58.67120857663339706, -0.3138064510428972831, -0.3172299661764663159 ) ) ;
#40012=CARTESIAN_POINT ( 'NONE',  ( -43.93237127071131454, 21.31409657049223227, 2.696834577194972216 ) ) ;
#40015=VERTEX_POINT ( 'NONE', #10581 ) ;
#40024=CARTESIAN_POINT ( 'NONE',  ( -57.62836615807631802, 1.308031921563323596, 1.276376674128435029 ) ) ;
#40025=CARTESIAN_POINT ( 'NONE',  ( -50.22242355904485578, 22.76272800790864181, 0.3424289802766369295 ) ) ;
#40026=EDGE_CURVE ( 'NONE', #9964, #33280, #38915, .T. ) ;
#40027=CARTESIAN_POINT ( 'NONE',  ( -51.02479983779974049, 14.46739584830851477, 4.600955224801048793 ) ) ;
#40028=CARTESIAN_POINT ( 'NONE',  ( -58.64020961342745153, -0.3060494297185549217, 0.3493912677027103397 ) ) ;
#40030=CARTESIAN_POINT ( 'NONE',  ( -30.15519950990045572, 69.97033940222175374, -1.270000000000007123 ) ) ;
#40031=ORIENTED_EDGE ( 'NONE', *, *, #7974, .T. ) ;
#40032=CARTESIAN_POINT ( 'NONE',  ( -44.96292901393739783, 21.56701576681934540, 3.486870777078499017 ) ) ;
#40043=CARTESIAN_POINT ( 'NONE',  ( -46.93088534759985464, 20.29541677029552460, 5.030633991647738945 ) ) ;
#40054=ORIENTED_EDGE ( 'NONE', *, *, #302, .T. ) ;
#40055=CARTESIAN_POINT ( 'NONE',  ( -48.74330358230356808, 18.21177412086844072, 5.147861347727184622 ) ) ;
#40062=CIRCLE ( 'NONE', #21640, 0.5080000000000000071 ) ;
#40067=ORIENTED_EDGE ( 'NONE', *, *, #2160, .F. ) ;
#40071=FACE_OUTER_BOUND ( 'NONE', #5766, .T. ) ;
#40079=ORIENTED_EDGE ( 'NONE', *, *, #28197, .F. ) ;
#40087=DIRECTION ( 'NONE',  ( -0.8745520943968250194, 0.4849315768086535083, -5.424246918827963022E-16 ) ) ;
#40093=DIRECTION ( 'NONE',  ( -5.188838149069472160E-16, 1.699382548006136559E-16, 1.000000000000000000 ) ) ;
#40094=ORIENTED_EDGE ( 'NONE', *, *, #1682, .F. ) ;
#40099=ORIENTED_EDGE ( 'NONE', *, *, #41610, .F. ) ;
#40100=DIRECTION ( 'NONE',  ( -0.9998501190848633202, -0.01731298258488772612, -5.158639060800499282E-16 ) ) ;
#40104=CARTESIAN_POINT ( 'NONE',  ( -46.95911617132934879, 24.98948415085533270, 1.986615011824473864 ) ) ;
#40107=AXIS2_PLACEMENT_3D ( 'NONE', #24084, #13875, #33272 ) ;
#40110=EDGE_LOOP ( 'NONE', ( #28966, #36810, #4889, #13971 ) ) ;
#40116=DIRECTION ( 'NONE',  ( -0.8745520943968235761, 0.4849315768086558398, -5.691349986800547879E-16 ) ) ;
#40117=CARTESIAN_POINT ( 'NONE',  ( -58.34765594471344485, -0.2451624547641084728, 0.1853313705894183983 ) ) ;
#40122=EDGE_CURVE ( 'NONE', #1088, #12215, #40613, .T. ) ;
#40128=AXIS2_PLACEMENT_3D ( 'NONE', #39569, #16113, #177 ) ;
#40129=CARTESIAN_POINT ( 'NONE',  ( -56.42052199906244425, 3.302738315264078128, -0.3606658556335856081 ) ) ;
#40131=DIRECTION ( 'NONE',  ( -0.8745520943968235761, 0.4849315768086558398, -4.268512490100410909E-16 ) ) ;
#40134=CARTESIAN_POINT ( 'NONE',  ( -30.84292043842125963, 55.46612528690534560, -1.270000000000195417 ) ) ;
#40136=CARTESIAN_POINT ( 'NONE',  ( -46.48884030892912023, 25.85920880503905650, 1.537089628573577338 ) ) ;
#40138=CARTESIAN_POINT ( 'NONE',  ( -57.78461401849437351, 2.885363594410703225, -1.046722867489131048E-14 ) ) ;
#40142=CARTESIAN_POINT ( 'NONE',  ( -58.20820809768405013, 1.420579653404072218, -1.355822160094615203 ) ) ;
#40145=CARTESIAN_POINT ( 'NONE',  ( -47.72737885966222393, 19.53144537861342656, -5.204668046373046586 ) ) ;
#40154=CARTESIAN_POINT ( 'NONE',  ( -49.90208883897420833, 16.45160819380948425, -4.945622778263405905 ) ) ;
#40155=CARTESIAN_POINT ( 'NONE',  ( -7.994219716368544226, 68.36415334912796027, -1.269999999999995577 ) ) ;
#40156=VERTEX_POINT ( 'NONE', #34221 ) ;
#40159=CARTESIAN_POINT ( 'NONE',  ( -58.29423361876341403, -0.1316707858636646522, -0.3525719584774348325 ) ) ;
#40163=CARTESIAN_POINT ( 'NONE',  ( -47.19936399096371105, 20.24790404726484283, -5.251082349106865443 ) ) ;
#40169=VERTEX_POINT ( 'NONE', #15020 ) ;
#40174=CARTESIAN_POINT ( 'NONE',  ( -50.58884987432006852, 15.93229845861179861, -5.010371253631922706 ) ) ;
#40175=CARTESIAN_POINT ( 'NONE',  ( -26.29578028364076658, 73.87584665086983193, -1.524000000000006017 ) ) ;
#40179=CIRCLE ( 'NONE', #30635, 0.3810000000000015041 ) ;
#40180=EDGE_CURVE ( 'NONE', #21262, #22469, #11938, .T. ) ;
#40187=CARTESIAN_POINT ( 'NONE',  ( -58.28497307353767809, -0.1385909279409680561, -1.015887430899425772E-14 ) ) ;
#40188=ADVANCED_FACE ( 'NONE', ( #11621 ), #27539, .T. ) ;
#40191=CARTESIAN_POINT ( 'NONE',  ( -47.93352606754567091, 24.19884373620804396, -0.9125764105762284029 ) ) ;
#40202=ORIENTED_EDGE ( 'NONE', *, *, #1402, .F. ) ;
#40207=ORIENTED_EDGE ( 'NONE', *, *, #30723, .T. ) ;
#40211=CARTESIAN_POINT ( 'NONE',  ( -58.65598178208009017, -0.3163282088987223739, -0.3245478190977730271 ) ) ;
#40215=CIRCLE ( 'NONE', #20439, 0.2540000000000018909 ) ;
#40217=ORIENTED_EDGE ( 'NONE', *, *, #610, .F. ) ;
#40223=EDGE_CURVE ( 'NONE', #20172, #23403, #33806, .T. ) ;
#40224=CARTESIAN_POINT ( 'NONE',  ( -8.438477507926629428, 69.62414081991882142, -1.523999999999995802 ) ) ;
#40225=ORIENTED_EDGE ( 'NONE', *, *, #30777, .F. ) ;
#40233=EDGE_CURVE ( 'NONE', #5054, #21592, #7983, .T. ) ;
#40235=CARTESIAN_POINT ( 'NONE',  ( -11.24191166894635074, 82.34025985790688651, -1.269999999999999574 ) ) ;
#40236=CARTESIAN_POINT ( 'NONE',  ( -56.16847044329335148, 4.408804334539881964, 2.360680022881862961 ) ) ;
#40238=CARTESIAN_POINT ( 'NONE',  ( -57.22363667057550884, 2.289652018204080264, 1.875138655370640173 ) ) ;
#40239=CARTESIAN_POINT ( 'NONE',  ( -58.57305159669930816, -0.1768144671344527297, 0.5299680571121552219 ) ) ;
#40244=CARTESIAN_POINT ( 'NONE',  ( -46.82679756180435504, 21.08486709759267086, 4.907624977305271585 ) ) ;
#40247=CIRCLE ( 'NONE', #1475, 0.5080000000000000071 ) ;
#40255=CARTESIAN_POINT ( 'NONE',  ( -45.96492958222027880, 21.02066589183244361, 4.445716362541716649 ) ) ;
#40257=CARTESIAN_POINT ( 'NONE',  ( -41.09670346151922615, 23.04688172092959775, 1.270085369932517194 ) ) ;
#40259=CARTESIAN_POINT ( 'NONE',  ( -17.99070523305416813, 61.93444992276926797, -1.269999999999999574 ) ) ;
#40264=CIRCLE ( 'NONE', #5557, 0.7620000000000015650 ) ;
#40268=ORIENTED_EDGE ( 'NONE', *, *, #25035, .F. ) ;
#40269=CARTESIAN_POINT ( 'NONE',  ( -48.77973395026506864, 17.81645205181620639, 4.684626272830461069 ) ) ;
#40280=VECTOR ( 'NONE', #17644, 1000.000000000000227 ) ;
#40283=ORIENTED_EDGE ( 'NONE', *, *, #31348, .T. ) ;
#40291=CARTESIAN_POINT ( 'NONE',  ( -28.09515292912719175, 77.51021392068167870, 1.269999999999992468 ) ) ;
#40294=ORIENTED_EDGE ( 'NONE', *, *, #6452, .T. ) ;
#40303=DIRECTION ( 'NONE',  ( 0.8745520943968240202, -0.4849315768086551182, 4.268512490100404500E-16 ) ) ;
#40314=ORIENTED_EDGE ( 'NONE', *, *, #311, .F. ) ;
#40315=CIRCLE ( 'NONE', #13110, 0.2540000000000012248 ) ;
#40316=ORIENTED_EDGE ( 'NONE', *, *, #30576, .T. ) ;
#40319=( LENGTH_UNIT ( ) NAMED_UNIT ( * ) SI_UNIT ( .MILLI., .METRE. ) );
#40330=AXIS2_PLACEMENT_3D ( 'NONE', #14964, #30322, #1375 ) ;
#40331=CARTESIAN_POINT ( 'NONE',  ( -58.34429324193580868, -0.2380942604818248043, 0.1989150628791497843 ) ) ;
#40340=CARTESIAN_POINT ( 'NONE',  ( -52.82621711067185544, 9.762356329794503296, -1.302233150175829302 ) ) ;
#40343=FACE_OUTER_BOUND ( 'NONE', #24058, .T. ) ;
#40345=CARTESIAN_POINT ( 'NONE',  ( -29.14841176306108039, 63.09186355671238999, -1.523999999996936250 ) ) ;
#40347=FACE_OUTER_BOUND ( 'NONE', #34312, .T. ) ;
#40349=CARTESIAN_POINT ( 'NONE',  ( -58.23655390014408084, 1.485667022650544178, 0.5301823895692101551 ) ) ;
#40352=ORIENTED_EDGE ( 'NONE', *, *, #39413, .F. ) ;
#40353=CARTESIAN_POINT ( 'NONE',  ( -56.90132276708389725, 4.901539372897764757, -1.453963793661438242 ) ) ;
#40354=ORIENTED_EDGE ( 'NONE', *, *, #12395, .T. ) ;
#40355=CARTESIAN_POINT ( 'NONE',  ( -45.65533061069547927, 20.86966646997169761, -4.138311239627009641 ) ) ;
#40359=AXIS2_PLACEMENT_3D ( 'NONE', #12623, #25611, #38621 ) ;
#40364=CARTESIAN_POINT ( 'NONE',  ( -49.91451862302049136, 16.43186916766678252, -4.943002434195075345 ) ) ;
#40365=VERTEX_POINT ( 'NONE', #12681 ) ;
#40368=CARTESIAN_POINT ( 'NONE',  ( -57.60581131635193231, 1.356655032538339967, -1.298406945959667214 ) ) ;
#40372=CARTESIAN_POINT ( 'NONE',  ( -47.71508057896579658, 20.49549959222711593, -5.111566084959475731 ) ) ;
#40373=AXIS2_PLACEMENT_3D ( 'NONE', #20387, #24218, #23800 ) ;
#40376=VERTEX_POINT ( 'NONE', #19272 ) ;
#40379=DIRECTION ( 'NONE',  ( 0.9454731675810338354, -0.3256999990547844170, 5.459396135145338185E-16 ) ) ;
#40381=CARTESIAN_POINT ( 'NONE',  ( -55.41603145274652320, 6.826612083464994818, -3.210495615568592420 ) ) ;
#40384=DIRECTION ( 'NONE',  ( 5.188838149069472160E-16, -1.699382548006136559E-16, -1.000000000000000000 ) ) ;
#40388=CIRCLE ( 'NONE', #21989, 0.6350000000000008971 ) ;
#40392=AXIS2_PLACEMENT_3D ( 'NONE', #7211, #31557, #6999 ) ;
#40393=CARTESIAN_POINT ( 'NONE',  ( -57.89731077922510849, 0.5615449381113774008, 0.05962325924456875204 ) ) ;
#40395=VERTEX_POINT ( 'NONE', #25875 ) ;
#40396=CARTESIAN_POINT ( 'NONE',  ( -46.81005371095113077, 25.73327194510126859, -1.583310528698486541 ) ) ;
#40398=CARTESIAN_POINT ( 'NONE',  ( -17.31476582418722643, 62.07284264934779827, -1.523999999999999355 ) ) ;
#40399=ORIENTED_EDGE ( 'NONE', *, *, #4821, .T. ) ;
#40410=CARTESIAN_POINT ( 'NONE',  ( -41.09670346151853693, 23.04688172093031540, -1.270085369932520303 ) ) ;
#40411=ORIENTED_EDGE ( 'NONE', *, *, #8199, .T. ) ;
#40417=CARTESIAN_POINT ( 'NONE',  ( -58.66375602224954378, -0.3143320623655576629, -0.3221285174456221534 ) ) ;
#40419=AXIS2_PLACEMENT_3D ( 'NONE', #40259, #17436, #17642 ) ;
#40422=EDGE_CURVE ( 'NONE', #15671, #40763, #40637, .T. ) ;
#40425=AXIS2_PLACEMENT_3D ( 'NONE', #20285, #30728, #7954 ) ;
#40430=ADVANCED_FACE ( 'NONE', ( #35068 ), #1187, .T. ) ;
#40435=CARTESIAN_POINT ( 'NONE',  ( -30.54923999206217289, 56.28999798340426253, -1.270000000000004903 ) ) ;
#40443=CARTESIAN_POINT ( 'NONE',  ( -57.86639066231883533, 0.7938686018777963982, 1.024763737755092885 ) ) ;
#40445=CARTESIAN_POINT ( 'NONE',  ( -58.55221842960730783, 0.5754175076986972615, 0.9757793345693576148 ) ) ;
#40446=CARTESIAN_POINT ( 'NONE',  ( -58.22293861823094829, 0.5799661241833895531, 1.107036107443613693 ) ) ;
#40452=CARTESIAN_POINT ( 'NONE',  ( -53.09398923718962493, 10.65108322687173548, 3.938325876039757478 ) ) ;
#40464=CARTESIAN_POINT ( 'NONE',  ( -41.05190940400897404, 23.09449711912554903, -1.270000000000012896 ) ) ;
#40465=CARTESIAN_POINT ( 'NONE',  ( -45.11690586071527775, 21.31720619196439159, 3.746636771226976137 ) ) ;
#40466=DIRECTION ( 'NONE',  ( -5.188838149069471174E-16, 1.699382548006136313E-16, 1.000000000000000000 ) ) ;
#40476=EDGE_LOOP ( 'NONE', ( #41543, #16653, #32726, #38870 ) ) ;
#40477=CARTESIAN_POINT ( 'NONE',  ( -51.79385399617232366, 10.81633633057992050, 0.6965991018155703873 ) ) ;
#40481=ORIENTED_EDGE ( 'NONE', *, *, #39425, .F. ) ;
#40484=DIRECTION ( 'NONE',  ( 0.4849315768086425726, 0.8745520943968309036, 1.030032898892908012E-16 ) ) ;
#40493=EDGE_CURVE ( 'NONE', #27477, #23556, #31105, .T. ) ;
#40494=DIRECTION ( 'NONE',  ( 0.8745520943968230210, -0.4849315768086570611, 6.829619984160674809E-16 ) ) ;
#40499=ORIENTED_EDGE ( 'NONE', *, *, #26963, .T. ) ;
#40508=ADVANCED_FACE ( 'NONE', ( #25471 ), #32452, .T. ) ;
#40509=FACE_OUTER_BOUND ( 'NONE', #12834, .T. ) ;
#40520=EDGE_CURVE ( 'NONE', #21812, #7720, #38678, .T. ) ;
#40522=ORIENTED_EDGE ( 'NONE', *, *, #22688, .F. ) ;
#40524=FACE_OUTER_BOUND ( 'NONE', #12034, .T. ) ;
#40537=CARTESIAN_POINT ( 'NONE',  ( -54.14414085402405163, 8.624088997049140559, 3.578441826534893622 ) ) ;
#40538=AXIS2_PLACEMENT_3D ( 'NONE', #28068, #21445, #24445 ) ;
#40546=CARTESIAN_POINT ( 'NONE',  ( -57.50808096206083775, 1.366199858870195794, -0.4699486091021616296 ) ) ;
#40549=DIRECTION ( 'NONE',  ( -0.8745520943968243532, 0.4849315768086547296, -5.361993529360573944E-16 ) ) ;
#40551=CARTESIAN_POINT ( 'NONE',  ( -20.05275907367747124, 79.68882802557934042, -1.524000000000003796 ) ) ;
#40553=ADVANCED_FACE ( 'NONE', ( #15864 ), #33164, .T. ) ;
#40559=FACE_OUTER_BOUND ( 'NONE', #792, .T. ) ;
#40560=EDGE_CURVE ( 'NONE', #28559, #29332, #34851, .T. ) ;
#40562=CARTESIAN_POINT ( 'NONE',  ( -46.50210365331269458, 20.51386735865872168, -4.739171082384393330 ) ) ;
#40569=CARTESIAN_POINT ( 'NONE',  ( -49.52378801310364054, 17.04469588244878153, -5.022789431048734876 ) ) ;
#40570=ORIENTED_EDGE ( 'NONE', *, *, #3677, .F. ) ;
#40574=CARTESIAN_POINT ( 'NONE',  ( -48.09695194791964923, 19.08878339914985034, -5.210713465316049842 ) ) ;
#40577=CARTESIAN_POINT ( 'NONE',  ( -45.14658554404967106, 22.88857079803865346, -2.562886992506571371 ) ) ;
#40579=ORIENTED_EDGE ( 'NONE', *, *, #25944, .T. ) ;
#40583=CARTESIAN_POINT ( 'NONE',  ( -57.57967628038989005, 1.451576601202181349, -1.494865757154152153 ) ) ;
#40587=VECTOR ( 'NONE', #1897, 1000.000000000000000 ) ;
#40590=CARTESIAN_POINT ( 'NONE',  ( -57.93941708942283952, 2.052042089854988483, -1.628789306319529118 ) ) ;
#40591=CIRCLE ( 'NONE', #33786, 0.2539999999999992264 ) ;
#40592=CARTESIAN_POINT ( 'NONE',  ( -41.31984638471809745, 22.80761424078405497, -1.396846000931804666 ) ) ;
#40595=CARTESIAN_POINT ( 'NONE',  ( -57.66977034847604955, 1.126272260461025354, 0.8071799157849385287 ) ) ;
#40598=CARTESIAN_POINT ( 'NONE',  ( -47.53841933257975683, 25.36174273411122115, -0.2940116119275095752 ) ) ;
#40601=ORIENTED_EDGE ( 'NONE', *, *, #1147, .F. ) ;
#40606=CIRCLE ( 'NONE', #14734, 0.2540000000000027236 ) ;
#40607=DIRECTION ( 'NONE',  ( 0.9511648638205648654, 0.3086833358527896753, 8.537024980200876052E-16 ) ) ;
#40613=LINE ( 'NONE', #24399, #1099 ) ;
#40614=ORIENTED_EDGE ( 'NONE', *, *, #34237, .T. ) ;
#40615=FACE_OUTER_BOUND ( 'NONE', #31419, .T. ) ;
#40620=CARTESIAN_POINT ( 'NONE',  ( -58.33992048227231209, -0.2288887037932701984, -0.2155571079148838054 ) ) ;
#40621=AXIS2_PLACEMENT_3D ( 'NONE', #11430, #5075, #2076 ) ;
#40626=ORIENTED_EDGE ( 'NONE', *, *, #37129, .T. ) ;
#40627=AXIS2_PLACEMENT_3D ( 'NONE', #24380, #40801, #15001 ) ;
#40637=CIRCLE ( 'NONE', #28375, 0.2539999999999980052 ) ;
#40644=CARTESIAN_POINT ( 'NONE',  ( -57.80874022462288764, 0.9184563934575655786, 1.089676212215488826 ) ) ;
#40645=CARTESIAN_POINT ( 'NONE',  ( -50.22374042606539035, 15.93784852756063586, 4.876865049933926777 ) ) ;
#40650=AXIS2_PLACEMENT_3D ( 'NONE', #2636, #27553, #14754 ) ;
#40652=CARTESIAN_POINT ( 'NONE',  ( -49.93490050754573417, 16.96705409125581099, 5.170188367178237598 ) ) ;
#40663=DIRECTION ( 'NONE',  ( -0.8745520943968243532, 0.4849315768086547296, -6.829619984160642269E-16 ) ) ;
#40664=CARTESIAN_POINT ( 'NONE',  ( -45.67969256299868164, 21.13156854447563759, 4.214927840906447010 ) ) ;
#40665=CARTESIAN_POINT ( 'NONE',  ( -47.90759336580052263, 19.42461454689798117, 5.304755467655303036 ) ) ;
#40667=CARTESIAN_POINT ( 'NONE',  ( -19.97113776634630256, 79.44829951959813741, -1.524000000000003574 ) ) ;
#40675=VECTOR ( 'NONE', #18168, 1000.000000000000227 ) ;
#40678=CARTESIAN_POINT ( 'NONE',  ( -47.83226487260633775, 16.75079348177631999, 1.615774049669061574 ) ) ;
#40693=CARTESIAN_POINT ( 'NONE',  ( -23.75997692595333177, 82.67351089148900201, -1.524000000000006239 ) ) ;
#40695=DIRECTION ( 'NONE',  ( -0.8745520943968235761, 0.4849315768086558398, -4.268512490100410909E-16 ) ) ;
#40713=ADVANCED_FACE ( 'NONE', ( #20105 ), #14074, .T. ) ;
#40718=VERTEX_POINT ( 'NONE', #759 ) ;
#40725=CARTESIAN_POINT ( 'NONE',  ( -17.14500000000466784, 71.11999999999886768, -1.524000000000000909 ) ) ;
#40732=CARTESIAN_POINT ( 'NONE',  ( -17.14500000000466784, 71.11999999999886768, 1.269999999999998241 ) ) ;
#40742=CARTESIAN_POINT ( 'NONE',  ( -58.43492521371286585, -0.3997831091909794798, 0.3282367010159537579 ) ) ;
#40749=EDGE_CURVE ( 'NONE', #14480, #1690, #33129, .T. ) ;
#40751=CARTESIAN_POINT ( 'NONE',  ( -57.60038635073814817, 1.097546858218806376, -1.033898108845213542E-14 ) ) ;
#40753=CARTESIAN_POINT ( 'NONE',  ( -29.48103325898055971, 60.42855201934086296, -1.270000000000005347 ) ) ;
#40756=CARTESIAN_POINT ( 'NONE',  ( -23.24761240069422286, 77.83567810938664877, 1.269999999999994023 ) ) ;
#40763=VERTEX_POINT ( 'NONE', #7561 ) ;
#40764=CARTESIAN_POINT ( 'NONE',  ( -58.43523997267251247, 0.9435442997105664142, -0.5849561510202232473 ) ) ;
#40767=CARTESIAN_POINT ( 'NONE',  ( -44.28332145682448839, 21.53821517059177637, -3.041508016573486461 ) ) ;
#40775=CARTESIAN_POINT ( 'NONE',  ( -49.52772409537172393, 17.03862487098385969, -5.022027238426779228 ) ) ;
#40776=ORIENTED_EDGE ( 'NONE', *, *, #41501, .F. ) ;
#40780=CARTESIAN_POINT ( 'NONE',  ( -53.26002898140129105, 10.27656598764010809, -3.765953445939742572 ) ) ;
#40783=CARTESIAN_POINT ( 'NONE',  ( -53.00789483126595769, 12.40033530745290236, -4.180047681284821515 ) ) ;
#40790=CARTESIAN_POINT ( 'NONE',  ( -57.26626398570029863, 3.526386058942967860, -2.205039086913768820 ) ) ;
#40793=DIRECTION ( 'NONE',  ( -0.3256999990547876367, -0.9454731675810326141, -8.328397965208553695E-18 ) ) ;
#40794=TOROIDAL_SURFACE ( 'NONE', #17628, 0.3809999999999990616, 0.2540000000000000036 ) ;
#40797=CARTESIAN_POINT ( 'NONE',  ( -56.21344593158320180, 5.939860726778031896, -2.828251681716873911 ) ) ;
#40798=CARTESIAN_POINT ( 'NONE',  ( -42.04356058215219605, 22.06167541775167606, -0.4953331422234020232 ) ) ;
#40799=EDGE_LOOP ( 'NONE', ( #1847, #9839, #1792, #11313 ) ) ;
#40801=DIRECTION ( 'NONE',  ( 0.6294287539884032556, 0.7770581983690836303, 1.945484789722780312E-16 ) ) ;
#40802=CARTESIAN_POINT ( 'NONE',  ( -58.31320831016853390, -0.1895118959954616988, 0.07592354283881128096 ) ) ;
#40803=CARTESIAN_POINT ( 'NONE',  ( -52.80069327121181288, 17.37962920081948681, 0.7126778406583705872 ) ) ;
#40805=ORIENTED_EDGE ( 'NONE', *, *, #16999, .F. ) ;
#40806=CARTESIAN_POINT ( 'NONE',  ( -49.18322560636019602, 21.37428572888716616, -2.217132718382757606 ) ) ;
#40817=CARTESIAN_POINT ( 'NONE',  ( -5.924740142096584172, 65.21691166894066782, -1.269999999999994023 ) ) ;
#40820=DIRECTION ( 'NONE',  ( 0.1951894777626526079, 0.9807655518882905099, -6.538892540527681903E-17 ) ) ;
#40824=ORIENTED_EDGE ( 'NONE', *, *, #6916, .F. ) ;
#40828=CARTESIAN_POINT ( 'NONE',  ( -58.30061145522432042, -0.1075020354497826652, -0.6732717543608098820 ) ) ;
#40837=DIRECTION ( 'NONE',  ( -5.188838149069471174E-16, 1.699382548006136313E-16, 1.000000000000000000 ) ) ;
#40842=DIRECTION ( 'NONE',  ( 0.8745520943968235761, -0.4849315768086558398, 0.000000000000000000 ) ) ;
#40843=VECTOR ( 'NONE', #37787, 1000.000000000000000 ) ;
#40848=CARTESIAN_POINT ( 'NONE',  ( -45.67973391888839529, 25.66060799623228661, -1.524000000000008237 ) ) ;
#40851=CARTESIAN_POINT ( 'NONE',  ( -58.36906557521628258, -0.2900353211930308817, 0.03225343758777150793 ) ) ;
#40856=ORIENTED_EDGE ( 'NONE', *, *, #29039, .T. ) ;
#40857=CARTESIAN_POINT ( 'NONE',  ( -48.08949201794742834, 19.91830422262442468, 5.194343260851632671 ) ) ;
#40870=CARTESIAN_POINT ( 'NONE',  ( -41.60680704299971922, 22.55277366187537780, 1.574601807764032468 ) ) ;
#40871=CARTESIAN_POINT ( 'NONE',  ( -19.33375693323417011, 80.42273151551299293, -1.270000000000003570 ) ) ;
#40875=DIRECTION ( 'NONE',  ( -0.4849315768086495115, -0.8745520943968271288, -7.999751396575051143E-15 ) ) ;
#40884=CARTESIAN_POINT ( 'NONE',  ( -56.42856387642236626, 3.193865871111118082, 0.1553879740655848829 ) ) ;
#40893=ORIENTED_EDGE ( 'NONE', *, *, #29629, .T. ) ;
#40895=CARTESIAN_POINT ( 'NONE',  ( -4.466782427718574588, 71.06098887363195615, 1.270000000000005791 ) ) ;
#40896=AXIS2_PLACEMENT_3D ( 'NONE', #13264, #26037, #9852 ) ;
#40899=DIRECTION ( 'NONE',  ( 0.8745520943968235761, -0.4849315768086558398, 4.268512490100410909E-16 ) ) ;
#40902=CARTESIAN_POINT ( 'NONE',  ( -42.09814309847200064, 23.46876350539121248, 1.523999999999994026 ) ) ;
#40907=FACE_OUTER_BOUND ( 'NONE', #38529, .T. ) ;
#40914=DIRECTION ( 'NONE',  ( 5.188838149069472160E-16, -1.699382548006136559E-16, -1.000000000000000000 ) ) ;
#40922=ORIENTED_EDGE ( 'NONE', *, *, #9101, .T. ) ;
#40927=AXIS2_PLACEMENT_3D ( 'NONE', #12636, #25622, #22405 ) ;
#40935=DIRECTION ( 'NONE',  ( -0.8745520943968235761, 0.4849315768086558398, -4.268512490100410909E-16 ) ) ;
#40940=CARTESIAN_POINT ( 'NONE',  ( -36.43259636504752308, 28.15155085495446485, -1.270000000000003348 ) ) ;
#40948=CARTESIAN_POINT ( 'NONE',  ( -58.60151899684544929, -0.7129426177415260080, 0.1461293658716241728 ) ) ;
#40949=EDGE_CURVE ( 'NONE', #33280, #41032, #20967, .T. ) ;
#40958=CARTESIAN_POINT ( 'NONE',  ( -57.47393550255000605, 1.325481720219651161, -0.09114234605509195786 ) ) ;
#40961=FACE_OUTER_BOUND ( 'NONE', #24899, .T. ) ;
#40962=DIRECTION ( 'NONE',  ( 5.188838149069471174E-16, -1.699382548006136313E-16, -1.000000000000000000 ) ) ;
#40965=LINE ( 'NONE', #24760, #38252 ) ;
#40971=CARTESIAN_POINT ( 'NONE',  ( -58.23655390014408084, 1.485667022650544178, -0.5301823895692313604 ) ) ;
#40972=VECTOR ( 'NONE', #18777, 1000.000000000000000 ) ;
#40974=EDGE_LOOP ( 'NONE', ( #8118, #33674, #31383, #6834, #6604 ) ) ;
#40975=CARTESIAN_POINT ( 'NONE',  ( -46.92937102808790684, 20.25120335581517850, -4.971330492145701108 ) ) ;
#40979=EDGE_CURVE ( 'NONE', #12640, #19740, #24963, .T. ) ;
#40983=CARTESIAN_POINT ( 'NONE',  ( -49.36731013057508477, 17.28484899067109737, -5.052703343809739955 ) ) ;
#40987=CARTESIAN_POINT ( 'NONE',  ( -56.41675102093069682, 3.888360460423796905, -2.207292246800581115 ) ) ;
#40990=CARTESIAN_POINT ( 'NONE',  ( -56.65231406860745977, 4.194353530936431262, -2.518504496425251205 ) ) ;
#40993=ORIENTED_EDGE ( 'NONE', *, *, #31856, .F. ) ;
#40997=CARTESIAN_POINT ( 'NONE',  ( -57.81953393267934160, 1.609514594907199392, -1.636666387507151432 ) ) ;
#41006=CARTESIAN_POINT ( 'NONE',  ( -41.31025181302593552, 22.81788724727718076, -1.523999999999993804 ) ) ;
#41008=CARTESIAN_POINT ( 'NONE',  ( -17.14500000000466784, 71.11999999999886768, 1.269999999999998241 ) ) ;
#41010=CARTESIAN_POINT ( 'NONE',  ( -57.91458998086623922, 0.5482684225795314559, 0.1438514718893008637 ) ) ;
#41011=CARTESIAN_POINT ( 'NONE',  ( -51.68408071790322822, 18.36713515631302585, 1.546689197337238753 ) ) ;
#41013=EDGE_LOOP ( 'NONE', ( #33475, #36151, #32268, #36319 ) ) ;
#41014=CARTESIAN_POINT ( 'NONE',  ( -48.35963184368405621, 21.82761434182101112, -2.838462189984265915 ) ) ;
#41017=ORIENTED_EDGE ( 'NONE', *, *, #17931, .F. ) ;
#41025=ADVANCED_FACE ( 'NONE', ( #38122 ), #16023, .F. ) ;
#41027=CARTESIAN_POINT ( 'NONE',  ( -26.29578028364076658, 73.87584665086983193, 1.269999999999993134 ) ) ;
#41030=CARTESIAN_POINT ( 'NONE',  ( -46.98357728082498852, 20.33138823660016214, -5.073745951255736131 ) ) ;
#41032=VERTEX_POINT ( 'NONE', #5197 ) ;
#41036=CARTESIAN_POINT ( 'NONE',  ( -58.52535285190720060, -0.5719483744804805259, -0.2498204902909159641 ) ) ;
#41042=ORIENTED_EDGE ( 'NONE', *, *, #7412, .T. ) ;
#41046=MECHANICAL_DESIGN_GEOMETRIC_PRESENTATION_REPRESENTATION('',(#17219),#34933);
#41047=CARTESIAN_POINT ( 'NONE',  ( -9.960492004070040650, 64.81807050032566053, -1.269999999999996021 ) ) ;
#41057=CARTESIAN_POINT ( 'NONE',  ( -42.09814309847200064, 23.46876350539121248, -1.524000000000005794 ) ) ;
#41060=CARTESIAN_POINT ( 'NONE',  ( -58.30142669622183860, -0.1470572696064289253, 0.3334503007892540283 ) ) ;
#41061=CYLINDRICAL_SURFACE ( 'NONE', #11232, 0.5080000000000000071 ) ;
#41065=VERTEX_POINT ( 'NONE', #5404 ) ;
#41066=CARTESIAN_POINT ( 'NONE',  ( -50.78166962549567387, 16.07998339508975860, 4.893817234114164805 ) ) ;
#41070=CIRCLE ( 'NONE', #28142, 0.2539999999999983937 ) ;
#41073=CARTESIAN_POINT ( 'NONE',  ( -28.65049350906917880, 77.81814547195517662, 1.269999999999990248 ) ) ;
#41075=EDGE_CURVE ( 'NONE', #2842, #17342, #5826, .T. ) ;
#41076=ORIENTED_EDGE ( 'NONE', *, *, #14506, .F. ) ;
#41078=CARTESIAN_POINT ( 'NONE',  ( -29.81772749323155836, 58.81923324275946641, 1.269999999999994023 ) ) ;
#41079=CYLINDRICAL_SURFACE ( 'NONE', #41204, 0.6350000000000006750 ) ;
#41080=CARTESIAN_POINT ( 'NONE',  ( -42.73979388487843067, 22.09733806376297238, 1.954747716863125984 ) ) ;
#41094=CARTESIAN_POINT ( 'NONE',  ( -55.83515739322318439, 4.224161455597882586, -9.574893020535344595E-15 ) ) ;
#41098=CIRCLE ( 'NONE', #31568, 0.2540000000000000036 ) ;
#41104=ORIENTED_EDGE ( 'NONE', *, *, #30723, .F. ) ;
#41107=CIRCLE ( 'NONE', #36351, 0.3810000000000007825 ) ;
#41108=CARTESIAN_POINT ( 'NONE',  ( -8.761523658392189162, 74.56051954986229191, -1.269999999999997131 ) ) ;
#41113=CARTESIAN_POINT ( 'NONE',  ( -19.21741104974024594, 79.92823415920659613, -1.524000000000003352 ) ) ;
#41114=CARTESIAN_POINT ( 'NONE',  ( -41.23752580366542020, 23.26788267949596190, -1.524000000000005128 ) ) ;
#41116=ORIENTED_EDGE ( 'NONE', *, *, #18498, .T. ) ;
#41118=DIRECTION ( 'NONE',  ( 0.4849315768086426282, 0.8745520943968310146, 1.030032898892908135E-16 ) ) ;
#41125=CARTESIAN_POINT ( 'NONE',  ( -29.94429436251954613, 71.80236127745905605, 1.269999999999991580 ) ) ;
#41136=VERTEX_POINT ( 'NONE', #41178 ) ;
#41143=VERTEX_POINT ( 'NONE', #11771 ) ;
#41147=DIRECTION ( 'NONE',  ( 0.01731298258488003436, -0.9998501190848634312, 0.000000000000000000 ) ) ;
#41151=DIRECTION ( 'NONE',  ( -0.8745520943968249084, 0.4849315768086533418, -5.271987356194193006E-16 ) ) ;
#41160=CARTESIAN_POINT ( 'NONE',  ( -54.71920516548560443, 7.857264873391931026, 3.427457936775551328 ) ) ;
#41167=ADVANCED_FACE ( 'NONE', ( #18360 ), #29746, .T. ) ;
#41170=CARTESIAN_POINT ( 'NONE',  ( -57.43854689232674815, 1.757847328446637825, -1.624773336220253439 ) ) ;
#41173=LINE ( 'NONE', #11977, #17154 ) ;
#41174=CARTESIAN_POINT ( 'NONE',  ( -5.719305292821792008, 76.92870498041706639, 1.270000000000003348 ) ) ;
#41177=CARTESIAN_POINT ( 'NONE',  ( -29.50431010628811990, 60.44740661353770150, 1.523999999999994026 ) ) ;
#41178=CARTESIAN_POINT ( 'NONE',  ( -5.878298779570172883, 78.21245918282636467, -1.269999999999996243 ) ) ;
#41182=EDGE_LOOP ( 'NONE', ( #2530, #17992, #28979, #1241 ) ) ;
#41183=CARTESIAN_POINT ( 'NONE',  ( -58.83227707057485389, -0.08366279997994163775, -5.785609034356198713E-15 ) ) ;
#41185=LINE ( 'NONE', #42032, #38945 ) ;
#41192=CARTESIAN_POINT ( 'NONE',  ( -57.87347402819683850, 1.335634876923293746, -1.488528580188531736 ) ) ;
#41197=B_SPLINE_SURFACE_WITH_KNOTS ( 'NONE', 3, 3, ( 
 ( #21584, #38233, #18616, #5441, #38015, #11598, #15423, #28425, #27997 ),
 ( #41006, #40592, #9049, #28212, #41431, #37384, #8200, #12237, #41219 ),
 ( #21374, #25228, #35044, #22015, #17775, #40798, #30773, #1623, #27583 ),
 ( #25014, #11812, #21171, #18399, #24582, #34202, #24803, #5028, #27789 ),
 ( #17985, #1823, #37796, #37588, #34400, #31190, #8416, #2034, #16045 ),
 ( #35668, #39278, #29048, #32673, #9460, #38652, #18827, #38855, #19658 ),
 ( #19453, #6478, #32463, #15628, #316, #42065, #3508, #31831, #13283 ),
 ( #19033, #2876, #15838, #32256, #26267, #22217, #16469, #25446, #2669 ),
 ( #35881, #28845, #5864, #3291, #35248, #35452, #12861, #6275, #16253 ),
 ( #22632, #22841, #29473, #28631, #10083, #26058, #29257, #38444, #23056 ),
 ( #6691, #19246, #6072, #9667, #9871, #25645, #32039, #3085, #41644 ),
 ( #12451, #9259, #41858, #12655, #103, #25848, #22424, #13068, #39069 ),
 ( #33310, #30305, #33101, #26701, #17518, #10297, #13912, #26905, #39706 ),
 ( #19874, #4354, #4139, #26487, #23692, #27328, #17100, #20711, #10508 ),
 ( #6903, #39918, #7744, #23478, #36503, #40340, #32888, #1358, #30518 ),
 ( #23910, #7123, #7324, #23266, #13499, #10712, #39491, #36301, #14117 ),
 ( #20078, #3932, #3720, #16891, #16679, #27114, #14316, #36926, #36711 ),
 ( #29893, #29683, #30103, #11133, #731, #13707, #7532, #20282, #527 ),
 ( #36089, #942, #20493, #33522, #17315, #1148, #40129, #10920, #33735 ),
 ( #4558, #33942, #34569, #14949, #11344, #5396, #2414, #15374, #8576 ),
 ( #24967, #37540, #24329, #27949, #28165, #1777, #37335, #11548, #8792 ),
 ( #41170, #37967, #28379, #41386, #37752, #5189, #4773, #11764, #30938 ),
 ( #21330, #18352, #21123, #14738, #5611, #40546, #1987, #40958, #27741 ),
 ( #7950, #31358, #34357, #14530, #24753, #24120, #18142, #21750, #40751 ),
 ( #37130, #21539, #34777, #24531, #8363, #20919, #17722, #31574, #18567 ),
 ( #11974, #8153, #31146, #34151, #1574, #2201, #27540, #4978, #15159 ),
 ( #17935, #30725, #22533, #35768, #9562, #3830, #36411, #13604, #422 ),
 ( #6585, #25744, #6795, #4039, #10088, #19552, #13392, #12961, #38753 ),
 ( #7229, #22952, #25955, #38962, #13182, #26169, #19762, #29588, #20188 ) ),
 .UNSPECIFIED., .F., .F., .F.,
 ( 4, 1, 1, 1, 1, 1, 1, 2, 1, 1, 1, 1, 1, 1, 1, 1, 1, 1, 1, 1, 1, 1, 1, 1, 1, 4 ),
 ( 4, 1, 1, 1, 1, 1, 4 ),
 ( 0.000000000000000000, 0.03307066603948304734, 0.06614133207896609468, 0.09921199811844919059, 0.1653533301974152714, 0.1984239962368983812, 0.2314946622763813522, 0.2645653283158643787, 0.3105299952961229071, 0.3564946622763812689, 0.4024593292566397418, 0.4484239962368982702, 0.5403533301974150493, 0.6322826641579321061, 0.7242119981184491628, 0.7701766650987074136, 0.8161413320789658865, 0.8850883325493537068, 0.8965794992944182695, 0.9080706660394826102, 0.9195618327845473949, 0.9310529995296121797, 0.9425441662746769644, 0.9540353330197415271, 0.9770176665098706525, 1.000000000000000000 ),
 ( 0.000000000000000000, 0.2500000000000000000, 0.4444444444444445308, 0.5000000000000000000, 0.7500000000000000000, 0.8333333333333333703, 1.000000000000000000 ),
 .UNSPECIFIED. ) ;
#41199=CARTESIAN_POINT ( 'NONE',  ( -57.36480510062817473, 1.874762252804534901, -1.516398777065382175 ) ) ;
#41202=CARTESIAN_POINT ( 'NONE',  ( -50.78166962549567387, 16.07998339508975860, -4.893817234114181680 ) ) ;
#41204=AXIS2_PLACEMENT_3D ( 'NONE', #4892, #27651, #8905 ) ;
#41206=ORIENTED_EDGE ( 'NONE', *, *, #5292, .F. ) ;
#41211=CARTESIAN_POINT ( 'NONE',  ( -57.55343345497419705, 2.880119995625998630, -1.988856187846590018 ) ) ;
#41219=CARTESIAN_POINT ( 'NONE',  ( -41.41491986784954804, 22.70581808553406233, -6.121743196690467558E-15 ) ) ;
#41220=EDGE_LOOP ( 'NONE', ( #3071, #2019, #19847, #30663 ) ) ;
#41222=CARTESIAN_POINT ( 'NONE',  ( -58.75009580408200094, 0.1057190229620807997, 0.6617493214610802310 ) ) ;
#41224=CARTESIAN_POINT ( 'NONE',  ( -17.08598887363762131, 83.79821757228496892, -1.270000000000002904 ) ) ;
#41225=CARTESIAN_POINT ( 'NONE',  ( -48.45250714818473625, 19.88962760504932348, 4.734234960885991050 ) ) ;
#41228=CARTESIAN_POINT ( 'NONE',  ( -48.87999295267864142, 23.89022491863793718, -0.5351834272454536467 ) ) ;
#41239=DIRECTION ( 'NONE',  ( -0.8745520943968240202, 0.4849315768086551737, -5.361993529360572958E-16 ) ) ;
#41253=EDGE_CURVE ( 'NONE', #26546, #21011, #22902, .T. ) ;
#41259=CARTESIAN_POINT ( 'NONE',  ( -41.97746338594183868, 23.60773098774231826, -1.524000000000005794 ) ) ;
#41261=VERTEX_POINT ( 'NONE', #2422 ) ;
#41266=CARTESIAN_POINT ( 'NONE',  ( -10.12396263145945419, 65.41168055974398499, -1.523999999999996247 ) ) ;
#41274=CARTESIAN_POINT ( 'NONE',  ( -58.30016403521963042, -0.1443550006728371859, 0.3367957002666301380 ) ) ;
#41279=ORIENTED_EDGE ( 'NONE', *, *, #36137, .F. ) ;
#41280=CARTESIAN_POINT ( 'NONE',  ( -50.29507671575587580, 15.72791930032350827, 4.796563717952097683 ) ) ;
#41283=AXIS2_PLACEMENT_3D ( 'NONE', #39374, #5959, #18918 ) ;
#41286=DIRECTION ( 'NONE',  ( -0.9816537812491077375, -0.1906721105965137331, 6.205370029530848928E-16 ) ) ;
#41288=EDGE_LOOP ( 'NONE', ( #35289, #25877, #30558, #29369 ) ) ;
#41290=CARTESIAN_POINT ( 'NONE',  ( -30.15519950990045572, 69.97033940222175374, 1.269999999999991358 ) ) ;
#41292=CARTESIAN_POINT ( 'NONE',  ( -42.22422426686605945, 22.06987237837733673, 1.558155077124570242 ) ) ;
#41298=CARTESIAN_POINT ( 'NONE',  ( -24.57769139521899149, 76.70147894597536720, 1.523999999999993804 ) ) ;
#41306=CARTESIAN_POINT ( 'NONE',  ( -56.90807066679607829, 2.849439543264234320, 1.873271221587421653 ) ) ;
#41319=AXIS2_PLACEMENT_3D ( 'NONE', #10350, #20757, #27164 ) ;
#41323=TOROIDAL_SURFACE ( 'NONE', #19525, 0.7620000000000000107, 0.2540000000000000036 ) ;
#41327=CARTESIAN_POINT ( 'NONE',  ( -46.68395179480138069, 26.03198510454123848, 1.396999999999990250 ) ) ;
#41329=CARTESIAN_POINT ( 'NONE',  ( -46.89970385779243855, 22.02655025333852379, 4.237790764466920379 ) ) ;
#41332=ORIENTED_EDGE ( 'NONE', *, *, #33876, .T. ) ;
#41334=FACE_OUTER_BOUND ( 'NONE', #20021, .T. ) ;
#41340=AXIS2_PLACEMENT_3D ( 'NONE', #396, #13363, #18376 ) ;
#41342=CARTESIAN_POINT ( 'NONE',  ( -10.75478607932181241, 82.07015292912137738, -1.523999999999999355 ) ) ;
#41347=CARTESIAN_POINT ( 'NONE',  ( -48.28978369826177186, 19.63653578263565436, 5.206999999995388428 ) ) ;
#41373=DIRECTION ( 'NONE',  ( -0.8745520943968250194, 0.4849315768086535638, -6.829619984160625506E-16 ) ) ;
#41376=CARTESIAN_POINT ( 'NONE',  ( -50.04979780823212820, 16.23027998584070275, 4.918765685678885724 ) ) ;
#41386=CARTESIAN_POINT ( 'NONE',  ( -57.40070531792823516, 1.672101763895803117, -0.9705777051858199833 ) ) ;
#41389=CARTESIAN_POINT ( 'NONE',  ( -19.15923810799328209, 79.68098548105338352, -1.524000000000003352 ) ) ;
#41393=DIRECTION ( 'NONE',  ( -0.8745520943968236871, 0.4849315768086559508, -6.829619984160659032E-16 ) ) ;
#41398=CARTESIAN_POINT ( 'NONE',  ( -58.29256068059346063, 1.279866164410503604, -0.9167068831667845030 ) ) ;
#41399=EDGE_LOOP ( 'NONE', ( #33286, #5957, #34519, #23253 ) ) ;
#41400=CARTESIAN_POINT ( 'NONE',  ( -42.32312746590514507, 22.34068395104271332, -1.752427511502158364 ) ) ;
#41407=CARTESIAN_POINT ( 'NONE',  ( -56.64692619791329520, 3.940143260488348176, -2.419031359405692250 ) ) ;
#41412=CARTESIAN_POINT ( 'NONE',  ( -54.16325525233833815, 8.500792493645910497, -3.386179713691846782 ) ) ;
#41413=AXIS2_PLACEMENT_3D ( 'NONE', #32997, #9557, #32557 ) ;
#41416=CARTESIAN_POINT ( 'NONE',  ( -49.39021242113546606, 17.77731941784099234, -5.290631085210052653 ) ) ;
#41423=CARTESIAN_POINT ( 'NONE',  ( -58.87911280034276018, -0.2081424763510641984, -1.061797465414398100E-14 ) ) ;
#41429=CARTESIAN_POINT ( 'NONE',  ( -29.89586364642802963, 71.55302121702176521, -1.270000000000007345 ) ) ;
#41430=TOROIDAL_SURFACE ( 'NONE', #4043, 0.3809999999999999498, 0.2540000000000000036 ) ;
#41431=CARTESIAN_POINT ( 'NONE',  ( -41.36952270831616119, 22.75442529069328401, -0.6632742133606294166 ) ) ;
#41432=VERTEX_POINT ( 'NONE', #7616 ) ;
#41433=DIRECTION ( 'NONE',  ( 5.188838149069472160E-16, -1.699382548006136559E-16, -1.000000000000000000 ) ) ;
#41434=TOROIDAL_SURFACE ( 'NONE', #28505, 8.794749999999996959, 0.2540000000000000036 ) ;
#41435=CARTESIAN_POINT ( 'NONE',  ( -57.50953982388014651, 1.662011999372992044, 1.631050346940570384 ) ) ;
#41436=CARTESIAN_POINT ( 'NONE',  ( -52.00466655731695909, 12.92300787752876801, 4.416453009321314127 ) ) ;
#41439=CARTESIAN_POINT ( 'NONE',  ( -51.02231935970569054, 20.76374992004582154, 0.7877321375940166126 ) ) ;
#41442=CARTESIAN_POINT ( 'NONE',  ( -50.22242355904485578, 22.76272800790864181, -0.3424289802766569690 ) ) ;
#41444=DIRECTION ( 'NONE',  ( -5.188838149069471174E-16, 1.699382548006136313E-16, 1.000000000000000000 ) ) ;
#41455=EDGE_CURVE ( 'NONE', #35910, #31840, #29769, .T. ) ;
#41458=DIRECTION ( 'NONE',  ( -0.6559537821943243197, 0.7548010569845282625, -8.537024980200743918E-16 ) ) ;
#41470=CIRCLE ( 'NONE', #27851, 2.285999999999998700 ) ;
#41472=CIRCLE ( 'NONE', #36693, 8.794749999999993406 ) ;
#41474=EDGE_CURVE ( 'NONE', #4116, #26517, #20875, .T. ) ;
#41476=ORIENTED_EDGE ( 'NONE', *, *, #2434, .F. ) ;
#41478=LINE ( 'NONE', #2294, #16787 ) ;
#41479=PLANE ( 'NONE',  #34792 ) ;
#41486=CARTESIAN_POINT ( 'NONE',  ( -58.32006471847083873, -0.1868378168976956022, 0.2819915271595720418 ) ) ;
#41489=CIRCLE ( 'NONE', #12230, 0.2540000000000000036 ) ;
#41490=CARTESIAN_POINT ( 'NONE',  ( -29.82321757229076908, 71.17901112636586447, 1.269999999999992690 ) ) ;
#41501=EDGE_CURVE ( 'NONE', #6194, #35513, #547, .T. ) ;
#41502=CARTESIAN_POINT ( 'NONE',  ( -32.57684172203629203, 51.47351799142593620, 1.524000000010915068 ) ) ;
#41505=CARTESIAN_POINT ( 'NONE',  ( -5.639506490940112471, 64.42185452804264401, 1.270000000000005569 ) ) ;
#41507=EDGE_CURVE ( 'NONE', #3540, #5200, #35903, .T. ) ;
#41515=ADVANCED_FACE ( 'NONE', ( #7405 ), #23640, .T. ) ;
#41518=CARTESIAN_POINT ( 'NONE',  ( -55.66968704194594153, 5.419822863896792242, 2.567922718055065445 ) ) ;
#41522=ORIENTED_EDGE ( 'NONE', *, *, #40026, .T. ) ;
#41524=DIRECTION ( 'NONE',  ( 5.188838149069472160E-16, -1.699382548006136559E-16, -1.000000000000000000 ) ) ;
#41536=CARTESIAN_POINT ( 'NONE',  ( -47.09845139715251605, 25.49303147219070098, 0.5484243623142188717 ) ) ;
#41539=CARTESIAN_POINT ( 'NONE',  ( -47.04837031381860157, 23.61299024743492581, 3.054033755318061871 ) ) ;
#41542=EDGE_CURVE ( 'NONE', #29748, #41570, #8671, .T. ) ;
#41543=ORIENTED_EDGE ( 'NONE', *, *, #10758, .F. ) ;
#41556=DIRECTION ( 'NONE',  ( -0.01731298258488003436, 0.9998501190848634312, 0.000000000000000000 ) ) ;
#41561=VERTEX_POINT ( 'NONE', #14765 ) ;
#41568=ORIENTED_EDGE ( 'NONE', *, *, #1518, .T. ) ;
#41569=EDGE_CURVE ( 'NONE', #332, #40156, #30440, .T. ) ;
#41570=VERTEX_POINT ( 'NONE', #4223 ) ;
#41583=VERTEX_POINT ( 'NONE', #30963 ) ;
#41588=CARTESIAN_POINT ( 'NONE',  ( -58.68789525397752271, -0.3143212917563475983, 0.3020521592211556916 ) ) ;
#41594=CARTESIAN_POINT ( 'NONE',  ( -24.24369025645185260, 82.02711331519694227, 1.269999999999992690 ) ) ;
#41599=LINE ( 'NONE', #42017, #6727 ) ;
#41600=CARTESIAN_POINT ( 'NONE',  ( -36.43259636504752308, 28.15155085495446485, -1.524000000000003352 ) ) ;
#41601=AXIS2_PLACEMENT_3D ( 'NONE', #11743, #18542, #41147 ) ;
#41604=LINE ( 'NONE', #12414, #13058 ) ;
#41609=DIRECTION ( 'NONE',  ( -0.9816537812491076265, -0.1906721105965138718, -4.769617732184456426E-16 ) ) ;
#41610=EDGE_CURVE ( 'NONE', #12215, #4082, #16971, .T. ) ;
#41611=ORIENTED_EDGE ( 'NONE', *, *, #32407, .F. ) ;
#41612=CARTESIAN_POINT ( 'NONE',  ( -17.64290547347870941, 83.78857423953914463, -1.270000000000003126 ) ) ;
#41616=EDGE_CURVE ( 'NONE', #8970, #32222, #1210, .T. ) ;
#41618=CARTESIAN_POINT ( 'NONE',  ( -57.59846039800395090, 1.925664279336513296, -1.733923949993310121 ) ) ;
#41619=ORIENTED_EDGE ( 'NONE', *, *, #22688, .T. ) ;
#41623=DIRECTION ( 'NONE',  ( -5.188838149069472160E-16, 1.699382548006136559E-16, 1.000000000000000000 ) ) ;
#41626=TOROIDAL_SURFACE ( 'NONE', #38215, 0.7620000000000000107, 0.2540000000000000036 ) ;
#41628=CARTESIAN_POINT ( 'NONE',  ( -55.60508136934060275, 7.116827924314645060, -3.170888472016298198 ) ) ;
#41630=EDGE_LOOP ( 'NONE', ( #39522, #26195, #25771, #10407 ) ) ;
#41635=CIRCLE ( 'NONE', #24601, 0.2540000000000002811 ) ;
#41637=CYLINDRICAL_SURFACE ( 'NONE', #20628, 0.6350000000000014522 ) ;
#41643=CARTESIAN_POINT ( 'NONE',  ( -10.57002714855771686, 82.40335727708655611, -1.523999999999999355 ) ) ;
#41644=CARTESIAN_POINT ( 'NONE',  ( -49.14072577824711630, 13.89916973120783972, -8.531461402113531655E-15 ) ) ;
#41647=CARTESIAN_POINT ( 'NONE',  ( -58.87911280034276018, -0.2081424763510641984, 0.2451831517279786654 ) ) ;
#41648=CARTESIAN_POINT ( 'NONE',  ( -53.87034488098446872, 9.496068333427519548, 3.775128525649497302 ) ) ;
#41651=CARTESIAN_POINT ( 'NONE',  ( -52.96141808003752516, 14.46028723511719960, 2.643142726894140537 ) ) ;
#41654=CARTESIAN_POINT ( 'NONE',  ( -47.35944255389389212, 21.37623662739411401, -4.722871667523173222 ) ) ;
#41656=DIRECTION ( 'NONE',  ( -0.9454731675810360558, 0.3256999990547780888, -5.459396135145339171E-16 ) ) ;
#41657=ORIENTED_EDGE ( 'NONE', *, *, #38139, .T. ) ;
#41663=TOROIDAL_SURFACE ( 'NONE', #163, 0.7620000000000000107, 0.2540000000000000036 ) ;
#41673=CARTESIAN_POINT ( 'NONE',  ( -58.35240408279319269, -0.2551309566431522735, -0.1643770683374448371 ) ) ;
#41688=DIRECTION ( 'NONE',  ( 0.2883665106726556182, 0.9575201071113218498, -1.461927526771632227E-15 ) ) ;
#41694=DIRECTION ( 'NONE',  ( 0.8745520943968243532, -0.4849315768086547296, 6.829619984160642269E-16 ) ) ;
#41695=CARTESIAN_POINT ( 'NONE',  ( -58.36603438765030916, -0.2837009127254847551, 0.07595423550348634478 ) ) ;
#41696=CIRCLE ( 'NONE', #27422, 0.2539999999999989488 ) ;
#41705=CARTESIAN_POINT ( 'NONE',  ( -41.05189575270519242, 23.09451173561982529, 1.270000000000008233 ) ) ;
#41707=ADVANCED_FACE ( 'NONE', ( #19735 ), #11394, .T. ) ;
#41710=CARTESIAN_POINT ( 'NONE',  ( -30.53944104307796081, 56.31939948586154543, 1.523999999999138932 ) ) ;
#41715=CARTESIAN_POINT ( 'NONE',  ( -25.54582022140424868, 74.24898932292961717, 1.269999999999993356 ) ) ;
#41720=TOROIDAL_SURFACE ( 'NONE', #23321, 8.794749999999998735, 0.2540000000000000036 ) ;
#41724=ORIENTED_EDGE ( 'NONE', *, *, #17876, .F. ) ;
#41726=CARTESIAN_POINT ( 'NONE',  ( -54.90394170586843359, 6.776736168479208011, 2.460356751892049942 ) ) ;
#41734=ADVANCED_FACE ( 'NONE', ( #12430 ), #7346, .T. ) ;
#41736=CARTESIAN_POINT ( 'NONE',  ( -41.28107547821692691, 23.22158991241129300, -1.523999999999999355 ) ) ;
#41738=ADVANCED_BREP_SHAPE_REPRESENTATION ( '', ( #24793, #3275 ), #20939 ) ;
#41740=EDGE_CURVE ( 'NONE', #37188, #31966, #24993, .T. ) ;
#41744=CARTESIAN_POINT ( 'NONE',  ( -13.99440778436217592, 79.95103047660883533, -1.270000000000000240 ) ) ;
#41747=CARTESIAN_POINT ( 'NONE',  ( -46.67763236942723637, 26.04755295256607539, 0.6632588273528772227 ) ) ;
#41749=CARTESIAN_POINT ( 'NONE',  ( -46.42538233320968288, 20.85422009098716956, 4.815137874471020041 ) ) ;
#41750=DIRECTION ( 'NONE',  ( 0.7770581983690701966, -0.6294287539884197979, 8.537024980200731099E-16 ) ) ;
#41753=ORIENTED_EDGE ( 'NONE', *, *, #26140, .F. ) ;
#41754=ORIENTED_EDGE ( 'NONE', *, *, #25333, .T. ) ;
#41761=CIRCLE ( 'NONE', #24069, 0.2539999999999998925 ) ;
#41764=CARTESIAN_POINT ( 'NONE',  ( -8.723850037987370243, 68.58388863026051752, -1.523999999999996025 ) ) ;
#41772=EDGE_LOOP ( 'NONE', ( #32425, #22928, #21318, #14375 ) ) ;
#41774=TOROIDAL_SURFACE ( 'NONE', #24747, 0.7620000000000000107, 0.2540000000000000036 ) ;
#41781=CARTESIAN_POINT ( 'NONE',  ( -41.05189575270517111, 23.09451173561986081, 1.396999999999993358 ) ) ;
#41784=DIRECTION ( 'NONE',  ( -0.9816537812491094028, -0.1906721105965052399, -7.903751763042053911E-15 ) ) ;
#41788=AXIS2_PLACEMENT_3D ( 'NONE', #17545, #26935, #23721 ) ;
#41790=CARTESIAN_POINT ( 'NONE',  ( -48.24248240369263385, 19.61030762366437585, -5.299013890195634957 ) ) ;
#41794=EDGE_CURVE ( 'NONE', #13695, #4510, #8817, .T. ) ;
#41796=DIRECTION ( 'NONE',  ( -0.8745520943968249084, 0.4849315768086536194, -5.575199987069925217E-16 ) ) ;
#41805=ADVANCED_FACE ( 'NONE', ( #11575 ), #16154, .T. ) ;
#41807=AXIS2_PLACEMENT_3D ( 'NONE', #3166, #12329, #41939 ) ;
#41808=EDGE_CURVE ( 'NONE', #4943, #41561, #27730, .T. ) ;
#41815=AXIS2_PLACEMENT_3D ( 'NONE', #8312, #11498, #11711 ) ;
#41816=CARTESIAN_POINT ( 'NONE',  ( -8.336765840796966032, 73.19241104973453105, -1.523999999999996691 ) ) ;
#41821=CARTESIAN_POINT ( 'NONE',  ( -46.96327221648707706, 24.95754849389498276, -2.007562630684416316 ) ) ;
#41828=ORIENTED_EDGE ( 'NONE', *, *, #12591, .T. ) ;
#41829=DIRECTION ( 'NONE',  ( -5.188838149069471174E-16, 1.699382548006136313E-16, 1.000000000000000000 ) ) ;
#41834=CARTESIAN_POINT ( 'NONE',  ( -58.41621559020261145, 0.1608283494537381952, -0.8351736514677311485 ) ) ;
#41836=CARTESIAN_POINT ( 'NONE',  ( -58.42460811326409242, -0.3780437665165939931, -0.3615838660060010090 ) ) ;
#41843=CARTESIAN_POINT ( 'NONE',  ( -57.39043856515510811, 2.569568763584578974, -1.997829887931768411 ) ) ;
#41850=CARTESIAN_POINT ( 'NONE',  ( -51.86985193027736329, 10.34936321858908492, -9.208787596046330052E-15 ) ) ;
#41853=FACE_OUTER_BOUND ( 'NONE', #37774, .T. ) ;
#41857=DIRECTION ( 'NONE',  ( 0.8745520943968250194, -0.4849315768086534528, 5.361993529360573944E-16 ) ) ;
#41858=CARTESIAN_POINT ( 'NONE',  ( -49.65974013515536711, 15.91765330076391116, -3.790917083309719438 ) ) ;
#41859=ORIENTED_EDGE ( 'NONE', *, *, #30286, .F. ) ;
#41860=DIRECTION ( 'NONE',  ( 5.188838149069472160E-16, -1.699382548006136559E-16, -1.000000000000000000 ) ) ;
#41861=CARTESIAN_POINT ( 'NONE',  ( -46.72244981118252838, 25.93862755320720836, -1.367307599761695025 ) ) ;
#41862=CARTESIAN_POINT ( 'NONE',  ( -51.46667322576657000, 13.85963790048950628, 4.568971727754695955 ) ) ;
#41863=DIRECTION ( 'NONE',  ( 5.188838149069472160E-16, -1.699382548006136066E-16, -1.000000000000000000 ) ) ;
#41865=CARTESIAN_POINT ( 'NONE',  ( -57.42300747107054093, 3.318281940618617032, 1.876676483338158619 ) ) ;
#41867=ORIENTED_EDGE ( 'NONE', *, *, #1409, .F. ) ;
#41868=CARTESIAN_POINT ( 'NONE',  ( -54.99893072520226411, 10.64604335972153137, -1.135982259999790855 ) ) ;
#41871=ORIENTED_EDGE ( 'NONE', *, *, #38602, .F. ) ;
#41884=ORIENTED_EDGE ( 'NONE', *, *, #1140, .F. ) ;
#41888=CARTESIAN_POINT ( 'NONE',  ( -58.36886504962463107, -0.2896226415746989691, -0.03617577931945905462 ) ) ;
#41899=CARTESIAN_POINT ( 'NONE',  ( -41.45218294293373162, 22.69057396248467384, -1.547390787314429472 ) ) ;
#41900=VERTEX_POINT ( 'NONE', #32016 ) ;
#41904=CARTESIAN_POINT ( 'NONE',  ( -8.816700480405424756, 73.94613776634058411, -1.523999999999996913 ) ) ;
#41908=CIRCLE ( 'NONE', #24857, 0.2540000000000010583 ) ;
#41911=CARTESIAN_POINT ( 'NONE',  ( -10.44685452804832160, 82.62549350906336088, 1.269999999999999796 ) ) ;
#41913=EDGE_LOOP ( 'NONE', ( #1587, #8837, #40283, #12573 ) ) ;
#41917=CARTESIAN_POINT ( 'NONE',  ( -41.05189575270520663, 23.09451173561983595, 1.523999999999993138 ) ) ;
#41921=CARTESIAN_POINT ( 'NONE',  ( -29.30242189341234393, 66.59148765007115855, 1.270000000000377272 ) ) ;
#41923=DIRECTION ( 'NONE',  ( -5.188838149069472160E-16, 1.699382548006136559E-16, 1.000000000000000000 ) ) ;
#41928=CARTESIAN_POINT ( 'NONE',  ( -54.28468382810587656, 8.706709151468123409, -3.613316249068738717 ) ) ;
#41939=DIRECTION ( 'NONE',  ( 0.6294287539884133587, 0.7770581983690755257, 0.000000000000000000 ) ) ;
#41945=CARTESIAN_POINT ( 'NONE',  ( -23.69188486464780752, 78.08202335040543574, -1.270000000000005347 ) ) ;
#41951=CARTESIAN_POINT ( 'NONE',  ( -48.86515451709912838, 17.99370625226629983, 5.095019330712561967 ) ) ;
#41952=CARTESIAN_POINT ( 'NONE',  ( -46.81330379368907302, 25.73549360603863434, 1.450859712031378201 ) ) ;
#41954=CARTESIAN_POINT ( 'NONE',  ( -45.68084146533627887, 21.25878370237693815, 4.188014402015102000 ) ) ;
#41955=DIRECTION ( 'NONE',  ( 0.6294287539884068083, 0.7770581983690809658, -6.679558114607132635E-15 ) ) ;
#41958=EDGE_LOOP ( 'NONE', ( #39265, #2118, #17330, #1524 ) ) ;
#41960=CARTESIAN_POINT ( 'NONE',  ( -6.135835944515187101, 77.40800365160224317, 1.270000000000002904 ) ) ;
#41967=LINE ( 'NONE', #12766, #3369 ) ;
#41976=ORIENTED_EDGE ( 'NONE', *, *, #17099, .F. ) ;
#41977=DIRECTION ( 'NONE',  ( -5.188838149069472160E-16, 1.699382548006136559E-16, 1.000000000000000000 ) ) ;
#41981=AXIS2_PLACEMENT_3D ( 'NONE', #34132, #15140, #4958 ) ;
#41984=ORIENTED_EDGE ( 'NONE', *, *, #37045, .F. ) ;
#41985=ORIENTED_EDGE ( 'NONE', *, *, #39384, .F. ) ;
#41986=CARTESIAN_POINT ( 'NONE',  ( -28.09515292912719175, 77.51021392068167870, -1.524000000000007571 ) ) ;
#41994=DIRECTION ( 'NONE',  ( -0.8745520943968247973, 0.4849315768086537304, -5.361993529360573944E-16 ) ) ;
#41998=TOROIDAL_SURFACE ( 'NONE', #38587, 0.3809999999999990616, 0.2540000000000000036 ) ;
#42004=DIRECTION ( 'NONE',  ( 0.9454731675810336133, -0.3256999990547843615, 5.459396135145337199E-16 ) ) ;
#42017=CARTESIAN_POINT ( 'NONE',  ( -30.15519950990045572, 69.97033940222175374, -1.524000000000007349 ) ) ;
#42018=CARTESIAN_POINT ( 'NONE',  ( -7.772068811996249771, 69.25462295839062676, 1.524000000000003796 ) ) ;
#42022=CARTESIAN_POINT ( 'NONE',  ( -18.88649316419433788, 79.99958772249931371, -1.524000000000003130 ) ) ;
#42027=VERTEX_POINT ( 'NONE', #14975 ) ;
#42028=ADVANCED_FACE ( 'NONE', ( #37776 ), #35024, .T. ) ;
#42032=CARTESIAN_POINT ( 'NONE',  ( -10.44685452804831804, 82.62549350906336088, -1.523999999999999355 ) ) ;
#42037=CARTESIAN_POINT ( 'NONE',  ( -56.39531427985796341, 4.462078775273103481, -2.567773104673984452 ) ) ;
#42039=CARTESIAN_POINT ( 'NONE',  ( -55.35389262108408559, 6.100188123699015641, -2.822635004244650414 ) ) ;
#42043=CARTESIAN_POINT ( 'NONE',  ( -19.33375693323417011, 80.42273151551299293, -1.524000000000003574 ) ) ;
#42044=EDGE_CURVE ( 'NONE', #16174, #21262, #4617, .T. ) ;
#42047=CARTESIAN_POINT ( 'NONE',  ( -57.78858274104275949, 1.044662872677112997, -1.355440516197766732 ) ) ;
#42056=CARTESIAN_POINT ( 'NONE',  ( -6.401666570281891566, 64.12941061790216679, -1.523999999999994026 ) ) ;
#42057=CARTESIAN_POINT ( 'NONE',  ( -50.02669608763528686, 12.78473261814649931, -8.449425852006687485E-15 ) ) ;
#42058=EDGE_CURVE ( 'NONE', #28714, #40169, #36597, .T. ) ;
#42065=CARTESIAN_POINT ( 'NONE',  ( -46.53889185657398286, 18.10826295091780835, -1.459106928557441618 ) ) ;
#42066=ORIENTED_EDGE ( 'NONE', *, *, #14611, .F. ) ;
#42067=DIRECTION ( 'NONE',  ( 0.5149185422762221354, -0.8572391118119438991, 4.128606161907600514E-16 ) ) ;
#42068=CARTESIAN_POINT ( 'NONE',  ( -46.74256434184148645, 25.89113524595070359, -1.391884290063961416 ) ) ;
#42069=CARTESIAN_POINT ( 'NONE',  ( -49.06145255062209287, 17.74692478680227836, 5.108567701946085116 ) ) ;
#42070=PLANE ( 'NONE',  #39254 ) ;
#42073=CARTESIAN_POINT ( 'NONE',  ( -56.90441949580814196, 4.712873715160811550, 1.842411344577081556 ) ) ;
#42075=CARTESIAN_POINT ( 'NONE',  ( -57.55343345497419705, 2.880119995625998630, 1.988856187846569146 ) ) ;
#42079=CARTESIAN_POINT ( 'NONE',  ( -49.59816314059868603, 17.91649583374772092, -5.069000701391663810 ) ) ;
#42081=ORIENTED_EDGE ( 'NONE', *, *, #27666, .T. ) ;
#42086=CARTESIAN_POINT ( 'NONE',  ( -22.98045850745951313, 78.35500052582088415, 1.523999999999994248 ) ) ;
#42089=DIRECTION ( 'NONE',  ( 0.7770581983690852956, -0.6294287539884014793, 6.050078592469978860E-15 ) ) ;
#42092=DIRECTION ( 'NONE',  ( 0.4849315768086533973, 0.8745520943968251304, 1.030032898892973955E-16 ) ) ;
#42096=ORIENTED_EDGE ( 'NONE', *, *, #5827, .T. ) ;
#42097=CARTESIAN_POINT ( 'NONE',  ( -58.36945504494742920, -0.2908306025726871136, -0.02357894785790005943 ) ) ;
#42101=TOROIDAL_SURFACE ( 'NONE', #29136, 0.7620000000000000107, 0.2540000000000000036 ) ;
#42110=CARTESIAN_POINT ( 'NONE',  ( -44.13308345971568514, 24.21351174012166396, -1.567149544246662973 ) ) ;
#42114=CIRCLE ( 'NONE', #36661, 0.6350000000000014522 ) ;
#42115=AXIS2_PLACEMENT_3D ( 'NONE', #24822, #21820, #21605 ) ;
#42121=CARTESIAN_POINT ( 'NONE',  ( -26.07365872405947727, 72.73903180058835005, -1.524000000000005794 ) ) ;
#42129=CARTESIAN_POINT ( 'NONE',  ( -10.57002714855771686, 82.40335727708655611, 1.524000000000000243 ) ) ;
#42138=AXIS2_PLACEMENT_3D ( 'NONE', #32959, #16746, #19096 ) ;
#42141=CYLINDRICAL_SURFACE ( 'NONE', #11594, 0.2539999999999989488 ) ;
#42147=ORIENTED_EDGE ( 'NONE', *, *, #2962, .T. ) ;
#42150=DIRECTION ( 'NONE',  ( -0.8745520943968235761, 0.4849315768086558953, -5.361993529360570985E-16 ) ) ;
#42157=CIRCLE ( 'NONE', #8129, 0.6350000000000006750 ) ;
#42159=CARTESIAN_POINT ( 'NONE',  ( -50.74392696651327839, 14.91217558840365953, 4.616263131616780591 ) ) ;
#42160=CARTESIAN_POINT ( 'NONE',  ( -46.68114719912644262, 26.04180998113828238, 1.171086909392312636 ) ) ;
ENDSEC;
END-ISO-10303-21;
